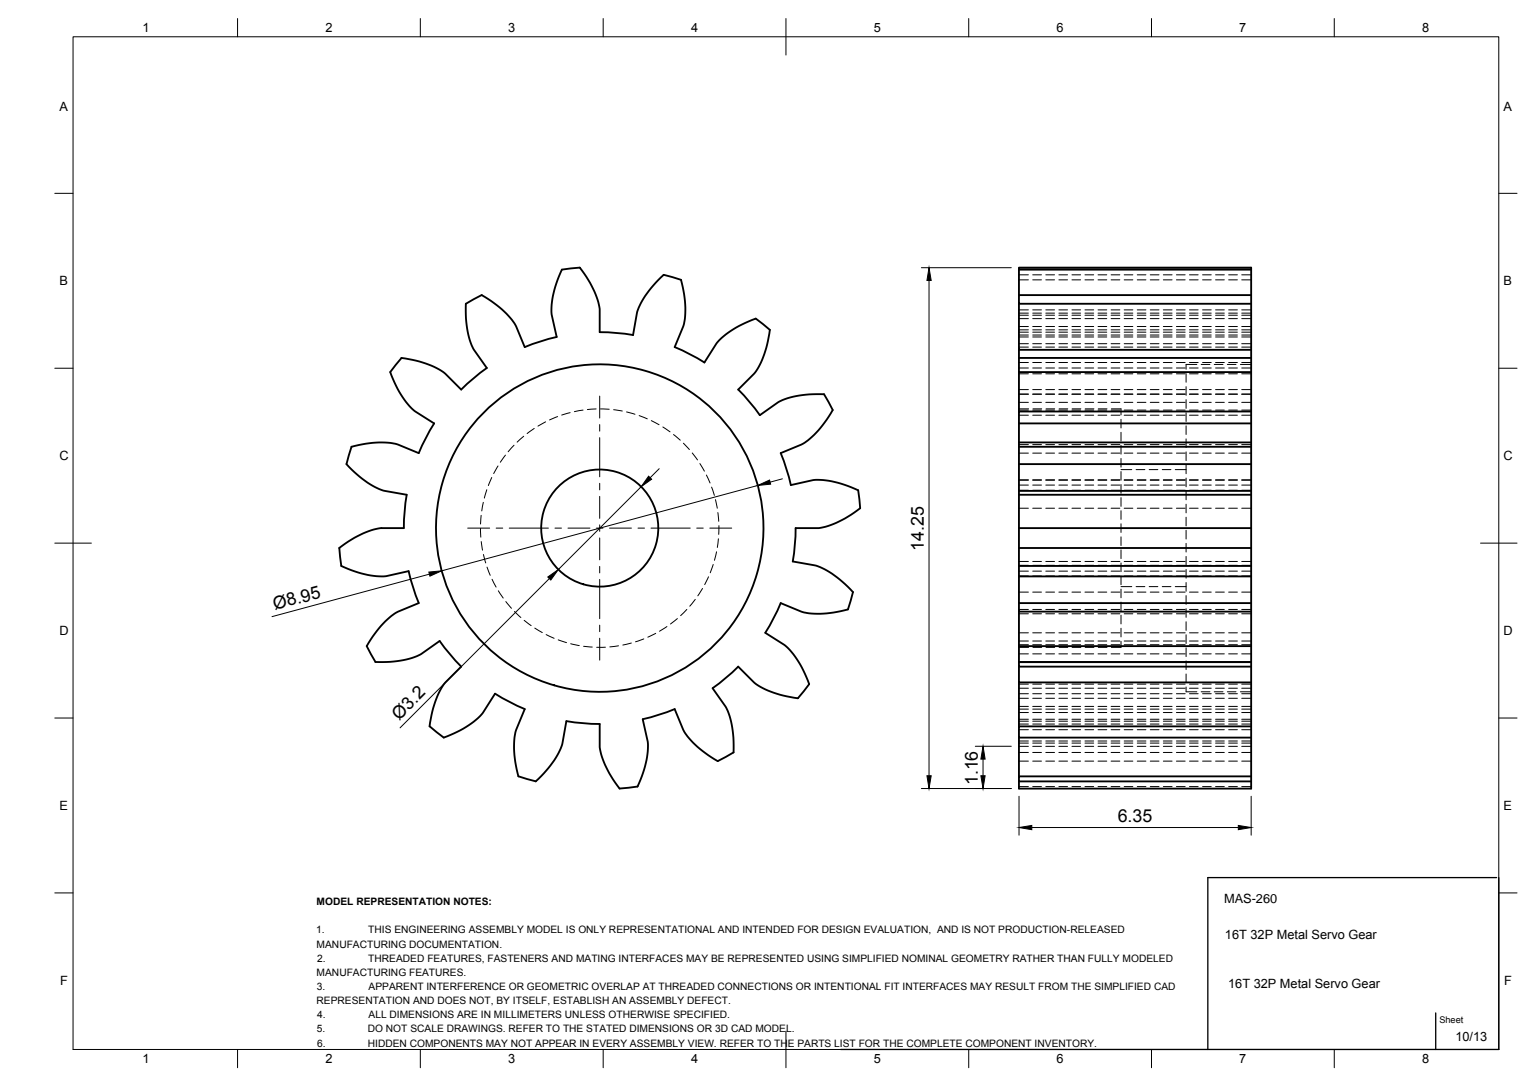
ISO-10303-21;
HEADER;
/* Generated by software containing ST-Developer
 * from STEP Tools, Inc. (www.steptools.com) 
 */

FILE_DESCRIPTION(
/* description */ (''),
/* implementation_level */ '2;1');

FILE_NAME(
/* name */ '16T 32P Metal Servo Gear.step',
/* time_stamp */ '2026-10-15T13:29:10-07:00',
/* author */ (''),
/* organization */ (''),
/* preprocessor_version */ 'ST-DEVELOPER v20.2',
/* originating_system */ 'Autodesk Translation Framework v15.15.0.0',
/* authorisation */ '');

FILE_SCHEMA (('AUTOMOTIVE_DESIGN { 1 0 10303 214 3 1 1 }'));
ENDSEC;

DATA;
#10=MECHANICAL_DESIGN_GEOMETRIC_PRESENTATION_REPRESENTATION('',(#936),#83219);
#508=B_SPLINE_CURVE_WITH_KNOTS('',5,(#37220,#37221,#37222,#37223,#37224,
#37225,#37226,#37227,#37228,#37229,#37230,#37231,#37232,#37233,#37234,#37235,
#37236,#37237,#37238,#37239,#37240,#37241,#37242,#37243,#37244,#37245,#37246,
#37247,#37248,#37249,#37250,#37251,#37252,#37253,#37254),.UNSPECIFIED.,
 .F.,.F.,(6,1,1,1,1,1,1,1,1,1,1,1,1,1,1,1,1,1,1,1,1,1,1,1,1,1,1,1,1,1,6),
(0.,0.0333333333333333,0.0666666666666667,0.1,0.133333333333333,0.166666666666667,
0.2,0.233333333333333,0.266666666666667,0.3,0.333333333333333,0.366666666666667,
0.4,0.433333333333333,0.466666666666667,0.5,0.533333333333333,0.566666666666667,
0.6,0.633333333333333,0.666666666666667,0.7,0.733333333333333,0.766666666666667,
0.8,0.833333333333333,0.866666666666667,0.9,0.933333333333333,0.966666666666667,
1.),.UNSPECIFIED.);
#509=B_SPLINE_CURVE_WITH_KNOTS('',5,(#37256,#37257,#37258,#37259,#37260,
#37261,#37262,#37263,#37264,#37265,#37266,#37267,#37268,#37269,#37270,#37271,
#37272,#37273,#37274,#37275,#37276,#37277,#37278,#37279,#37280,#37281,#37282,
#37283,#37284,#37285,#37286,#37287,#37288,#37289,#37290),.UNSPECIFIED.,
 .F.,.F.,(6,1,1,1,1,1,1,1,1,1,1,1,1,1,1,1,1,1,1,1,1,1,1,1,1,1,1,1,1,1,6),
(0.,0.0333333333333333,0.0666666666666667,0.1,0.133333333333333,0.166666666666667,
0.2,0.233333333333333,0.266666666666667,0.3,0.333333333333333,0.366666666666667,
0.4,0.433333333333333,0.466666666666667,0.5,0.533333333333333,0.566666666666667,
0.6,0.633333333333333,0.666666666666667,0.7,0.733333333333333,0.766666666666667,
0.8,0.833333333333333,0.866666666666667,0.9,0.933333333333333,0.966666666666667,
1.),.UNSPECIFIED.);
#510=B_SPLINE_CURVE_WITH_KNOTS('',5,(#37368,#37369,#37370,#37371,#37372,
#37373,#37374,#37375,#37376,#37377,#37378,#37379,#37380,#37381,#37382,#37383,
#37384,#37385,#37386,#37387,#37388,#37389,#37390,#37391,#37392,#37393,#37394,
#37395,#37396,#37397,#37398,#37399,#37400,#37401,#37402),.UNSPECIFIED.,
 .F.,.F.,(6,1,1,1,1,1,1,1,1,1,1,1,1,1,1,1,1,1,1,1,1,1,1,1,1,1,1,1,1,1,6),
(0.,0.0333333333333333,0.0666666666666667,0.1,0.133333333333333,0.166666666666667,
0.2,0.233333333333333,0.266666666666667,0.3,0.333333333333333,0.366666666666667,
0.4,0.433333333333333,0.466666666666667,0.5,0.533333333333333,0.566666666666667,
0.6,0.633333333333333,0.666666666666667,0.7,0.733333333333333,0.766666666666667,
0.8,0.833333333333333,0.866666666666667,0.9,0.933333333333333,0.966666666666667,
1.),.UNSPECIFIED.);
#511=B_SPLINE_CURVE_WITH_KNOTS('',5,(#37403,#37404,#37405,#37406,#37407,
#37408,#37409,#37410,#37411,#37412,#37413,#37414,#37415,#37416,#37417,#37418,
#37419,#37420,#37421,#37422,#37423,#37424,#37425,#37426,#37427,#37428,#37429,
#37430,#37431,#37432,#37433,#37434,#37435,#37436,#37437),.UNSPECIFIED.,
 .F.,.F.,(6,1,1,1,1,1,1,1,1,1,1,1,1,1,1,1,1,1,1,1,1,1,1,1,1,1,1,1,1,1,6),
(-1.,-0.966666666666667,-0.933333333333333,-0.9,-0.866666666666667,-0.833333333333333,
-0.8,-0.766666666666667,-0.733333333333333,-0.7,-0.666666666666667,-0.633333333333333,
-0.6,-0.566666666666667,-0.533333333333333,-0.5,-0.466666666666667,-0.433333333333333,
-0.4,-0.366666666666667,-0.333333333333333,-0.3,-0.266666666666667,-0.233333333333333,
-0.2,-0.166666666666667,-0.133333333333333,-0.1,-0.0666666666666667,-0.0333333333333333,
0.),.UNSPECIFIED.);
#512=B_SPLINE_CURVE_WITH_KNOTS('',5,(#37444,#37445,#37446,#37447,#37448,
#37449,#37450,#37451,#37452,#37453,#37454,#37455,#37456,#37457,#37458,#37459,
#37460,#37461,#37462,#37463,#37464,#37465,#37466,#37467,#37468,#37469,#37470,
#37471,#37472,#37473,#37474,#37475,#37476,#37477,#37478),.UNSPECIFIED.,
 .F.,.F.,(6,1,1,1,1,1,1,1,1,1,1,1,1,1,1,1,1,1,1,1,1,1,1,1,1,1,1,1,1,1,6),
(0.,0.0333333333333333,0.0666666666666667,0.1,0.133333333333333,0.166666666666667,
0.2,0.233333333333333,0.266666666666667,0.3,0.333333333333333,0.366666666666667,
0.4,0.433333333333333,0.466666666666667,0.5,0.533333333333333,0.566666666666667,
0.6,0.633333333333333,0.666666666666667,0.7,0.733333333333333,0.766666666666667,
0.8,0.833333333333333,0.866666666666667,0.9,0.933333333333333,0.966666666666667,
1.),.UNSPECIFIED.);
#513=B_SPLINE_CURVE_WITH_KNOTS('',5,(#37482,#37483,#37484,#37485,#37486,
#37487,#37488,#37489,#37490,#37491,#37492,#37493,#37494,#37495,#37496,#37497,
#37498,#37499,#37500,#37501,#37502,#37503,#37504,#37505,#37506,#37507,#37508,
#37509,#37510,#37511,#37512,#37513,#37514,#37515,#37516),.UNSPECIFIED.,
 .F.,.F.,(6,1,1,1,1,1,1,1,1,1,1,1,1,1,1,1,1,1,1,1,1,1,1,1,1,1,1,1,1,1,6),
(0.,0.0333333333333333,0.0666666666666667,0.1,0.133333333333333,0.166666666666667,
0.2,0.233333333333333,0.266666666666667,0.3,0.333333333333333,0.366666666666667,
0.4,0.433333333333333,0.466666666666667,0.5,0.533333333333333,0.566666666666667,
0.6,0.633333333333333,0.666666666666667,0.7,0.733333333333333,0.766666666666667,
0.8,0.833333333333333,0.866666666666667,0.9,0.933333333333333,0.966666666666667,
1.),.UNSPECIFIED.);
#514=B_SPLINE_CURVE_WITH_KNOTS('',5,(#37524,#37525,#37526,#37527,#37528,
#37529,#37530,#37531,#37532,#37533,#37534,#37535,#37536,#37537,#37538,#37539,
#37540,#37541,#37542,#37543,#37544,#37545,#37546,#37547,#37548,#37549,#37550,
#37551,#37552,#37553,#37554,#37555,#37556,#37557,#37558),.UNSPECIFIED.,
 .F.,.F.,(6,1,1,1,1,1,1,1,1,1,1,1,1,1,1,1,1,1,1,1,1,1,1,1,1,1,1,1,1,1,6),
(0.,0.0333333333333333,0.0666666666666667,0.1,0.133333333333333,0.166666666666667,
0.2,0.233333333333333,0.266666666666667,0.3,0.333333333333333,0.366666666666667,
0.4,0.433333333333333,0.466666666666667,0.5,0.533333333333333,0.566666666666667,
0.6,0.633333333333333,0.666666666666667,0.7,0.733333333333333,0.766666666666667,
0.8,0.833333333333333,0.866666666666667,0.9,0.933333333333333,0.966666666666667,
1.),.UNSPECIFIED.);
#515=B_SPLINE_CURVE_WITH_KNOTS('',5,(#37562,#37563,#37564,#37565,#37566,
#37567,#37568,#37569,#37570,#37571,#37572,#37573,#37574,#37575,#37576,#37577,
#37578,#37579,#37580,#37581,#37582,#37583,#37584,#37585,#37586,#37587,#37588,
#37589,#37590,#37591,#37592,#37593,#37594,#37595,#37596),.UNSPECIFIED.,
 .F.,.F.,(6,1,1,1,1,1,1,1,1,1,1,1,1,1,1,1,1,1,1,1,1,1,1,1,1,1,1,1,1,1,6),
(0.,0.0333333333333333,0.0666666666666667,0.1,0.133333333333333,0.166666666666667,
0.2,0.233333333333333,0.266666666666667,0.3,0.333333333333333,0.366666666666667,
0.4,0.433333333333333,0.466666666666667,0.5,0.533333333333333,0.566666666666667,
0.6,0.633333333333333,0.666666666666667,0.7,0.733333333333333,0.766666666666667,
0.8,0.833333333333333,0.866666666666667,0.9,0.933333333333333,0.966666666666667,
1.),.UNSPECIFIED.);
#516=B_SPLINE_CURVE_WITH_KNOTS('',5,(#37604,#37605,#37606,#37607,#37608,
#37609,#37610,#37611,#37612,#37613,#37614,#37615,#37616,#37617,#37618,#37619,
#37620,#37621,#37622,#37623,#37624,#37625,#37626,#37627,#37628,#37629,#37630,
#37631,#37632,#37633,#37634,#37635,#37636,#37637,#37638),.UNSPECIFIED.,
 .F.,.F.,(6,1,1,1,1,1,1,1,1,1,1,1,1,1,1,1,1,1,1,1,1,1,1,1,1,1,1,1,1,1,6),
(0.,0.0333333333333333,0.0666666666666667,0.1,0.133333333333333,0.166666666666667,
0.2,0.233333333333333,0.266666666666667,0.3,0.333333333333333,0.366666666666667,
0.4,0.433333333333333,0.466666666666667,0.5,0.533333333333333,0.566666666666667,
0.6,0.633333333333333,0.666666666666667,0.7,0.733333333333333,0.766666666666667,
0.8,0.833333333333333,0.866666666666667,0.9,0.933333333333333,0.966666666666667,
1.),.UNSPECIFIED.);
#517=B_SPLINE_CURVE_WITH_KNOTS('',5,(#37642,#37643,#37644,#37645,#37646,
#37647,#37648,#37649,#37650,#37651,#37652,#37653,#37654,#37655,#37656,#37657,
#37658,#37659,#37660,#37661,#37662,#37663,#37664,#37665,#37666,#37667,#37668,
#37669,#37670,#37671,#37672,#37673,#37674,#37675,#37676),.UNSPECIFIED.,
 .F.,.F.,(6,1,1,1,1,1,1,1,1,1,1,1,1,1,1,1,1,1,1,1,1,1,1,1,1,1,1,1,1,1,6),
(0.,0.0333333333333333,0.0666666666666667,0.1,0.133333333333333,0.166666666666667,
0.2,0.233333333333333,0.266666666666667,0.3,0.333333333333333,0.366666666666667,
0.4,0.433333333333333,0.466666666666667,0.5,0.533333333333333,0.566666666666667,
0.6,0.633333333333333,0.666666666666667,0.7,0.733333333333333,0.766666666666667,
0.8,0.833333333333333,0.866666666666667,0.9,0.933333333333333,0.966666666666667,
1.),.UNSPECIFIED.);
#518=B_SPLINE_CURVE_WITH_KNOTS('',5,(#37684,#37685,#37686,#37687,#37688,
#37689,#37690,#37691,#37692,#37693,#37694,#37695,#37696,#37697,#37698,#37699,
#37700,#37701,#37702,#37703,#37704,#37705,#37706,#37707,#37708,#37709,#37710,
#37711,#37712,#37713,#37714,#37715,#37716,#37717,#37718),.UNSPECIFIED.,
 .F.,.F.,(6,1,1,1,1,1,1,1,1,1,1,1,1,1,1,1,1,1,1,1,1,1,1,1,1,1,1,1,1,1,6),
(0.,0.0333333333333333,0.0666666666666667,0.1,0.133333333333333,0.166666666666667,
0.2,0.233333333333333,0.266666666666667,0.3,0.333333333333333,0.366666666666667,
0.4,0.433333333333333,0.466666666666667,0.5,0.533333333333333,0.566666666666667,
0.6,0.633333333333333,0.666666666666667,0.7,0.733333333333333,0.766666666666667,
0.8,0.833333333333333,0.866666666666667,0.9,0.933333333333333,0.966666666666667,
1.),.UNSPECIFIED.);
#519=B_SPLINE_CURVE_WITH_KNOTS('',5,(#37722,#37723,#37724,#37725,#37726,
#37727,#37728,#37729,#37730,#37731,#37732,#37733,#37734,#37735,#37736,#37737,
#37738,#37739,#37740,#37741,#37742,#37743,#37744,#37745,#37746,#37747,#37748,
#37749,#37750,#37751,#37752,#37753,#37754,#37755,#37756),.UNSPECIFIED.,
 .F.,.F.,(6,1,1,1,1,1,1,1,1,1,1,1,1,1,1,1,1,1,1,1,1,1,1,1,1,1,1,1,1,1,6),
(0.,0.0333333333333333,0.0666666666666667,0.1,0.133333333333333,0.166666666666667,
0.2,0.233333333333333,0.266666666666667,0.3,0.333333333333333,0.366666666666667,
0.4,0.433333333333333,0.466666666666667,0.5,0.533333333333333,0.566666666666667,
0.6,0.633333333333333,0.666666666666667,0.7,0.733333333333333,0.766666666666667,
0.8,0.833333333333333,0.866666666666667,0.9,0.933333333333333,0.966666666666667,
1.),.UNSPECIFIED.);
#520=B_SPLINE_CURVE_WITH_KNOTS('',5,(#37764,#37765,#37766,#37767,#37768,
#37769,#37770,#37771,#37772,#37773,#37774,#37775,#37776,#37777,#37778,#37779,
#37780,#37781,#37782,#37783,#37784,#37785,#37786,#37787,#37788,#37789,#37790,
#37791,#37792,#37793,#37794,#37795,#37796,#37797,#37798),.UNSPECIFIED.,
 .F.,.F.,(6,1,1,1,1,1,1,1,1,1,1,1,1,1,1,1,1,1,1,1,1,1,1,1,1,1,1,1,1,1,6),
(0.,0.0333333333333333,0.0666666666666667,0.1,0.133333333333333,0.166666666666667,
0.2,0.233333333333333,0.266666666666667,0.3,0.333333333333333,0.366666666666667,
0.4,0.433333333333333,0.466666666666667,0.5,0.533333333333333,0.566666666666667,
0.6,0.633333333333333,0.666666666666667,0.7,0.733333333333333,0.766666666666667,
0.8,0.833333333333333,0.866666666666667,0.9,0.933333333333333,0.966666666666667,
1.),.UNSPECIFIED.);
#521=B_SPLINE_CURVE_WITH_KNOTS('',5,(#37802,#37803,#37804,#37805,#37806,
#37807,#37808,#37809,#37810,#37811,#37812,#37813,#37814,#37815,#37816,#37817,
#37818,#37819,#37820,#37821,#37822,#37823,#37824,#37825,#37826,#37827,#37828,
#37829,#37830,#37831,#37832,#37833,#37834,#37835,#37836),.UNSPECIFIED.,
 .F.,.F.,(6,1,1,1,1,1,1,1,1,1,1,1,1,1,1,1,1,1,1,1,1,1,1,1,1,1,1,1,1,1,6),
(0.,0.0333333333333333,0.0666666666666667,0.1,0.133333333333333,0.166666666666667,
0.2,0.233333333333333,0.266666666666667,0.3,0.333333333333333,0.366666666666667,
0.4,0.433333333333333,0.466666666666667,0.5,0.533333333333333,0.566666666666667,
0.6,0.633333333333333,0.666666666666667,0.7,0.733333333333333,0.766666666666667,
0.8,0.833333333333333,0.866666666666667,0.9,0.933333333333333,0.966666666666667,
1.),.UNSPECIFIED.);
#522=B_SPLINE_CURVE_WITH_KNOTS('',5,(#37844,#37845,#37846,#37847,#37848,
#37849,#37850,#37851,#37852,#37853,#37854,#37855,#37856,#37857,#37858,#37859,
#37860,#37861,#37862,#37863,#37864,#37865,#37866,#37867,#37868,#37869,#37870,
#37871,#37872,#37873,#37874,#37875,#37876,#37877,#37878),.UNSPECIFIED.,
 .F.,.F.,(6,1,1,1,1,1,1,1,1,1,1,1,1,1,1,1,1,1,1,1,1,1,1,1,1,1,1,1,1,1,6),
(0.,0.0333333333333333,0.0666666666666667,0.1,0.133333333333333,0.166666666666667,
0.2,0.233333333333333,0.266666666666667,0.3,0.333333333333333,0.366666666666667,
0.4,0.433333333333333,0.466666666666667,0.5,0.533333333333333,0.566666666666667,
0.6,0.633333333333333,0.666666666666667,0.7,0.733333333333333,0.766666666666667,
0.8,0.833333333333333,0.866666666666667,0.9,0.933333333333333,0.966666666666667,
1.),.UNSPECIFIED.);
#523=B_SPLINE_CURVE_WITH_KNOTS('',5,(#37882,#37883,#37884,#37885,#37886,
#37887,#37888,#37889,#37890,#37891,#37892,#37893,#37894,#37895,#37896,#37897,
#37898,#37899,#37900,#37901,#37902,#37903,#37904,#37905,#37906,#37907,#37908,
#37909,#37910,#37911,#37912,#37913,#37914,#37915,#37916),.UNSPECIFIED.,
 .F.,.F.,(6,1,1,1,1,1,1,1,1,1,1,1,1,1,1,1,1,1,1,1,1,1,1,1,1,1,1,1,1,1,6),
(0.,0.0333333333333333,0.0666666666666667,0.1,0.133333333333333,0.166666666666667,
0.2,0.233333333333333,0.266666666666667,0.3,0.333333333333333,0.366666666666667,
0.4,0.433333333333333,0.466666666666667,0.5,0.533333333333333,0.566666666666667,
0.6,0.633333333333333,0.666666666666667,0.7,0.733333333333333,0.766666666666667,
0.8,0.833333333333333,0.866666666666667,0.9,0.933333333333333,0.966666666666667,
1.),.UNSPECIFIED.);
#524=B_SPLINE_CURVE_WITH_KNOTS('',5,(#37924,#37925,#37926,#37927,#37928,
#37929,#37930,#37931,#37932,#37933,#37934,#37935,#37936,#37937,#37938,#37939,
#37940,#37941,#37942,#37943,#37944,#37945,#37946,#37947,#37948,#37949,#37950,
#37951,#37952,#37953,#37954,#37955,#37956,#37957,#37958),.UNSPECIFIED.,
 .F.,.F.,(6,1,1,1,1,1,1,1,1,1,1,1,1,1,1,1,1,1,1,1,1,1,1,1,1,1,1,1,1,1,6),
(0.,0.0333333333333333,0.0666666666666667,0.1,0.133333333333333,0.166666666666667,
0.2,0.233333333333333,0.266666666666667,0.3,0.333333333333333,0.366666666666667,
0.4,0.433333333333333,0.466666666666667,0.5,0.533333333333333,0.566666666666667,
0.6,0.633333333333333,0.666666666666667,0.7,0.733333333333333,0.766666666666667,
0.8,0.833333333333333,0.866666666666667,0.9,0.933333333333333,0.966666666666667,
1.),.UNSPECIFIED.);
#525=B_SPLINE_CURVE_WITH_KNOTS('',5,(#37962,#37963,#37964,#37965,#37966,
#37967,#37968,#37969,#37970,#37971,#37972,#37973,#37974,#37975,#37976,#37977,
#37978,#37979,#37980,#37981,#37982,#37983,#37984,#37985,#37986,#37987,#37988,
#37989,#37990,#37991,#37992,#37993,#37994,#37995,#37996),.UNSPECIFIED.,
 .F.,.F.,(6,1,1,1,1,1,1,1,1,1,1,1,1,1,1,1,1,1,1,1,1,1,1,1,1,1,1,1,1,1,6),
(0.,0.0333333333333333,0.0666666666666667,0.1,0.133333333333333,0.166666666666667,
0.2,0.233333333333333,0.266666666666667,0.3,0.333333333333333,0.366666666666667,
0.4,0.433333333333333,0.466666666666667,0.5,0.533333333333333,0.566666666666667,
0.6,0.633333333333333,0.666666666666667,0.7,0.733333333333333,0.766666666666667,
0.8,0.833333333333333,0.866666666666667,0.9,0.933333333333333,0.966666666666667,
1.),.UNSPECIFIED.);
#526=B_SPLINE_CURVE_WITH_KNOTS('',5,(#38004,#38005,#38006,#38007,#38008,
#38009,#38010,#38011,#38012,#38013,#38014,#38015,#38016,#38017,#38018,#38019,
#38020,#38021,#38022,#38023,#38024,#38025,#38026,#38027,#38028,#38029,#38030,
#38031,#38032,#38033,#38034,#38035,#38036,#38037,#38038),.UNSPECIFIED.,
 .F.,.F.,(6,1,1,1,1,1,1,1,1,1,1,1,1,1,1,1,1,1,1,1,1,1,1,1,1,1,1,1,1,1,6),
(0.,0.0333333333333333,0.0666666666666667,0.1,0.133333333333333,0.166666666666667,
0.2,0.233333333333333,0.266666666666667,0.3,0.333333333333333,0.366666666666667,
0.4,0.433333333333333,0.466666666666667,0.5,0.533333333333333,0.566666666666667,
0.6,0.633333333333333,0.666666666666667,0.7,0.733333333333333,0.766666666666667,
0.8,0.833333333333333,0.866666666666667,0.9,0.933333333333333,0.966666666666667,
1.),.UNSPECIFIED.);
#527=B_SPLINE_CURVE_WITH_KNOTS('',5,(#38042,#38043,#38044,#38045,#38046,
#38047,#38048,#38049,#38050,#38051,#38052,#38053,#38054,#38055,#38056,#38057,
#38058,#38059,#38060,#38061,#38062,#38063,#38064,#38065,#38066,#38067,#38068,
#38069,#38070,#38071,#38072,#38073,#38074,#38075,#38076),.UNSPECIFIED.,
 .F.,.F.,(6,1,1,1,1,1,1,1,1,1,1,1,1,1,1,1,1,1,1,1,1,1,1,1,1,1,1,1,1,1,6),
(0.,0.0333333333333333,0.0666666666666667,0.1,0.133333333333333,0.166666666666667,
0.2,0.233333333333333,0.266666666666667,0.3,0.333333333333333,0.366666666666667,
0.4,0.433333333333333,0.466666666666667,0.5,0.533333333333333,0.566666666666667,
0.6,0.633333333333333,0.666666666666667,0.7,0.733333333333333,0.766666666666667,
0.8,0.833333333333333,0.866666666666667,0.9,0.933333333333333,0.966666666666667,
1.),.UNSPECIFIED.);
#528=B_SPLINE_CURVE_WITH_KNOTS('',5,(#38084,#38085,#38086,#38087,#38088,
#38089,#38090,#38091,#38092,#38093,#38094,#38095,#38096,#38097,#38098,#38099,
#38100,#38101,#38102,#38103,#38104,#38105,#38106,#38107,#38108,#38109,#38110,
#38111,#38112,#38113,#38114,#38115,#38116,#38117,#38118),.UNSPECIFIED.,
 .F.,.F.,(6,1,1,1,1,1,1,1,1,1,1,1,1,1,1,1,1,1,1,1,1,1,1,1,1,1,1,1,1,1,6),
(0.,0.0333333333333333,0.0666666666666667,0.1,0.133333333333333,0.166666666666667,
0.2,0.233333333333333,0.266666666666667,0.3,0.333333333333333,0.366666666666667,
0.4,0.433333333333333,0.466666666666667,0.5,0.533333333333333,0.566666666666667,
0.6,0.633333333333333,0.666666666666667,0.7,0.733333333333333,0.766666666666667,
0.8,0.833333333333333,0.866666666666667,0.9,0.933333333333333,0.966666666666667,
1.),.UNSPECIFIED.);
#529=B_SPLINE_CURVE_WITH_KNOTS('',5,(#38122,#38123,#38124,#38125,#38126,
#38127,#38128,#38129,#38130,#38131,#38132,#38133,#38134,#38135,#38136,#38137,
#38138,#38139,#38140,#38141,#38142,#38143,#38144,#38145,#38146,#38147,#38148,
#38149,#38150,#38151,#38152,#38153,#38154,#38155,#38156),.UNSPECIFIED.,
 .F.,.F.,(6,1,1,1,1,1,1,1,1,1,1,1,1,1,1,1,1,1,1,1,1,1,1,1,1,1,1,1,1,1,6),
(0.,0.0333333333333333,0.0666666666666667,0.1,0.133333333333333,0.166666666666667,
0.2,0.233333333333333,0.266666666666667,0.3,0.333333333333333,0.366666666666667,
0.4,0.433333333333333,0.466666666666667,0.5,0.533333333333333,0.566666666666667,
0.6,0.633333333333333,0.666666666666667,0.7,0.733333333333333,0.766666666666667,
0.8,0.833333333333333,0.866666666666667,0.9,0.933333333333333,0.966666666666667,
1.),.UNSPECIFIED.);
#530=B_SPLINE_CURVE_WITH_KNOTS('',5,(#38164,#38165,#38166,#38167,#38168,
#38169,#38170,#38171,#38172,#38173,#38174,#38175,#38176,#38177,#38178,#38179,
#38180,#38181,#38182,#38183,#38184,#38185,#38186,#38187,#38188,#38189,#38190,
#38191,#38192,#38193,#38194,#38195,#38196,#38197,#38198),.UNSPECIFIED.,
 .F.,.F.,(6,1,1,1,1,1,1,1,1,1,1,1,1,1,1,1,1,1,1,1,1,1,1,1,1,1,1,1,1,1,6),
(0.,0.0333333333333333,0.0666666666666667,0.1,0.133333333333333,0.166666666666667,
0.2,0.233333333333333,0.266666666666667,0.3,0.333333333333333,0.366666666666667,
0.4,0.433333333333333,0.466666666666667,0.5,0.533333333333333,0.566666666666667,
0.6,0.633333333333333,0.666666666666667,0.7,0.733333333333333,0.766666666666667,
0.8,0.833333333333333,0.866666666666667,0.9,0.933333333333333,0.966666666666667,
1.),.UNSPECIFIED.);
#531=B_SPLINE_CURVE_WITH_KNOTS('',5,(#38202,#38203,#38204,#38205,#38206,
#38207,#38208,#38209,#38210,#38211,#38212,#38213,#38214,#38215,#38216,#38217,
#38218,#38219,#38220,#38221,#38222,#38223,#38224,#38225,#38226,#38227,#38228,
#38229,#38230,#38231,#38232,#38233,#38234,#38235,#38236),.UNSPECIFIED.,
 .F.,.F.,(6,1,1,1,1,1,1,1,1,1,1,1,1,1,1,1,1,1,1,1,1,1,1,1,1,1,1,1,1,1,6),
(0.,0.0333333333333333,0.0666666666666667,0.1,0.133333333333333,0.166666666666667,
0.2,0.233333333333333,0.266666666666667,0.3,0.333333333333333,0.366666666666667,
0.4,0.433333333333333,0.466666666666667,0.5,0.533333333333333,0.566666666666667,
0.6,0.633333333333333,0.666666666666667,0.7,0.733333333333333,0.766666666666667,
0.8,0.833333333333333,0.866666666666667,0.9,0.933333333333333,0.966666666666667,
1.),.UNSPECIFIED.);
#532=B_SPLINE_CURVE_WITH_KNOTS('',5,(#38244,#38245,#38246,#38247,#38248,
#38249,#38250,#38251,#38252,#38253,#38254,#38255,#38256,#38257,#38258,#38259,
#38260,#38261,#38262,#38263,#38264,#38265,#38266,#38267,#38268,#38269,#38270,
#38271,#38272,#38273,#38274,#38275,#38276,#38277,#38278),.UNSPECIFIED.,
 .F.,.F.,(6,1,1,1,1,1,1,1,1,1,1,1,1,1,1,1,1,1,1,1,1,1,1,1,1,1,1,1,1,1,6),
(0.,0.0333333333333333,0.0666666666666667,0.1,0.133333333333333,0.166666666666667,
0.2,0.233333333333333,0.266666666666667,0.3,0.333333333333333,0.366666666666667,
0.4,0.433333333333333,0.466666666666667,0.5,0.533333333333333,0.566666666666667,
0.6,0.633333333333333,0.666666666666667,0.7,0.733333333333333,0.766666666666667,
0.8,0.833333333333333,0.866666666666667,0.9,0.933333333333333,0.966666666666667,
1.),.UNSPECIFIED.);
#533=B_SPLINE_CURVE_WITH_KNOTS('',5,(#38282,#38283,#38284,#38285,#38286,
#38287,#38288,#38289,#38290,#38291,#38292,#38293,#38294,#38295,#38296,#38297,
#38298,#38299,#38300,#38301,#38302,#38303,#38304,#38305,#38306,#38307,#38308,
#38309,#38310,#38311,#38312,#38313,#38314,#38315,#38316),.UNSPECIFIED.,
 .F.,.F.,(6,1,1,1,1,1,1,1,1,1,1,1,1,1,1,1,1,1,1,1,1,1,1,1,1,1,1,1,1,1,6),
(0.,0.0333333333333333,0.0666666666666667,0.1,0.133333333333333,0.166666666666667,
0.2,0.233333333333333,0.266666666666667,0.3,0.333333333333333,0.366666666666667,
0.4,0.433333333333333,0.466666666666667,0.5,0.533333333333333,0.566666666666667,
0.6,0.633333333333333,0.666666666666667,0.7,0.733333333333333,0.766666666666667,
0.8,0.833333333333333,0.866666666666667,0.9,0.933333333333333,0.966666666666667,
1.),.UNSPECIFIED.);
#534=B_SPLINE_CURVE_WITH_KNOTS('',5,(#38324,#38325,#38326,#38327,#38328,
#38329,#38330,#38331,#38332,#38333,#38334,#38335,#38336,#38337,#38338,#38339,
#38340,#38341,#38342,#38343,#38344,#38345,#38346,#38347,#38348,#38349,#38350,
#38351,#38352,#38353,#38354,#38355,#38356,#38357,#38358),.UNSPECIFIED.,
 .F.,.F.,(6,1,1,1,1,1,1,1,1,1,1,1,1,1,1,1,1,1,1,1,1,1,1,1,1,1,1,1,1,1,6),
(0.,0.0333333333333333,0.0666666666666667,0.1,0.133333333333333,0.166666666666667,
0.2,0.233333333333333,0.266666666666667,0.3,0.333333333333333,0.366666666666667,
0.4,0.433333333333333,0.466666666666667,0.5,0.533333333333333,0.566666666666667,
0.6,0.633333333333333,0.666666666666667,0.7,0.733333333333333,0.766666666666667,
0.8,0.833333333333333,0.866666666666667,0.9,0.933333333333333,0.966666666666667,
1.),.UNSPECIFIED.);
#535=B_SPLINE_CURVE_WITH_KNOTS('',5,(#38362,#38363,#38364,#38365,#38366,
#38367,#38368,#38369,#38370,#38371,#38372,#38373,#38374,#38375,#38376,#38377,
#38378,#38379,#38380,#38381,#38382,#38383,#38384,#38385,#38386,#38387,#38388,
#38389,#38390,#38391,#38392,#38393,#38394,#38395,#38396),.UNSPECIFIED.,
 .F.,.F.,(6,1,1,1,1,1,1,1,1,1,1,1,1,1,1,1,1,1,1,1,1,1,1,1,1,1,1,1,1,1,6),
(0.,0.0333333333333333,0.0666666666666667,0.1,0.133333333333333,0.166666666666667,
0.2,0.233333333333333,0.266666666666667,0.3,0.333333333333333,0.366666666666667,
0.4,0.433333333333333,0.466666666666667,0.5,0.533333333333333,0.566666666666667,
0.6,0.633333333333333,0.666666666666667,0.7,0.733333333333333,0.766666666666667,
0.8,0.833333333333333,0.866666666666667,0.9,0.933333333333333,0.966666666666667,
1.),.UNSPECIFIED.);
#536=B_SPLINE_CURVE_WITH_KNOTS('',5,(#38404,#38405,#38406,#38407,#38408,
#38409,#38410,#38411,#38412,#38413,#38414,#38415,#38416,#38417,#38418,#38419,
#38420,#38421,#38422,#38423,#38424,#38425,#38426,#38427,#38428,#38429,#38430,
#38431,#38432,#38433,#38434,#38435,#38436,#38437,#38438),.UNSPECIFIED.,
 .F.,.F.,(6,1,1,1,1,1,1,1,1,1,1,1,1,1,1,1,1,1,1,1,1,1,1,1,1,1,1,1,1,1,6),
(0.,0.0333333333333333,0.0666666666666667,0.1,0.133333333333333,0.166666666666667,
0.2,0.233333333333333,0.266666666666667,0.3,0.333333333333333,0.366666666666667,
0.4,0.433333333333333,0.466666666666667,0.5,0.533333333333333,0.566666666666667,
0.6,0.633333333333333,0.666666666666667,0.7,0.733333333333333,0.766666666666667,
0.8,0.833333333333333,0.866666666666667,0.9,0.933333333333333,0.966666666666667,
1.),.UNSPECIFIED.);
#537=B_SPLINE_CURVE_WITH_KNOTS('',5,(#38442,#38443,#38444,#38445,#38446,
#38447,#38448,#38449,#38450,#38451,#38452,#38453,#38454,#38455,#38456,#38457,
#38458,#38459,#38460,#38461,#38462,#38463,#38464,#38465,#38466,#38467,#38468,
#38469,#38470,#38471,#38472,#38473,#38474,#38475,#38476),.UNSPECIFIED.,
 .F.,.F.,(6,1,1,1,1,1,1,1,1,1,1,1,1,1,1,1,1,1,1,1,1,1,1,1,1,1,1,1,1,1,6),
(0.,0.0333333333333333,0.0666666666666667,0.1,0.133333333333333,0.166666666666667,
0.2,0.233333333333333,0.266666666666667,0.3,0.333333333333333,0.366666666666667,
0.4,0.433333333333333,0.466666666666667,0.5,0.533333333333333,0.566666666666667,
0.6,0.633333333333333,0.666666666666667,0.7,0.733333333333333,0.766666666666667,
0.8,0.833333333333333,0.866666666666667,0.9,0.933333333333333,0.966666666666667,
1.),.UNSPECIFIED.);
#538=B_SPLINE_CURVE_WITH_KNOTS('',5,(#38484,#38485,#38486,#38487,#38488,
#38489,#38490,#38491,#38492,#38493,#38494,#38495,#38496,#38497,#38498,#38499,
#38500,#38501,#38502,#38503,#38504,#38505,#38506,#38507,#38508,#38509,#38510,
#38511,#38512,#38513,#38514,#38515,#38516,#38517,#38518),.UNSPECIFIED.,
 .F.,.F.,(6,1,1,1,1,1,1,1,1,1,1,1,1,1,1,1,1,1,1,1,1,1,1,1,1,1,1,1,1,1,6),
(0.,0.0333333333333333,0.0666666666666667,0.1,0.133333333333333,0.166666666666667,
0.2,0.233333333333333,0.266666666666667,0.3,0.333333333333333,0.366666666666667,
0.4,0.433333333333333,0.466666666666667,0.5,0.533333333333333,0.566666666666667,
0.6,0.633333333333333,0.666666666666667,0.7,0.733333333333333,0.766666666666667,
0.8,0.833333333333333,0.866666666666667,0.9,0.933333333333333,0.966666666666667,
1.),.UNSPECIFIED.);
#539=B_SPLINE_CURVE_WITH_KNOTS('',5,(#38522,#38523,#38524,#38525,#38526,
#38527,#38528,#38529,#38530,#38531,#38532,#38533,#38534,#38535,#38536,#38537,
#38538,#38539,#38540,#38541,#38542,#38543,#38544,#38545,#38546,#38547,#38548,
#38549,#38550,#38551,#38552,#38553,#38554,#38555,#38556),.UNSPECIFIED.,
 .F.,.F.,(6,1,1,1,1,1,1,1,1,1,1,1,1,1,1,1,1,1,1,1,1,1,1,1,1,1,1,1,1,1,6),
(0.,0.0333333333333333,0.0666666666666667,0.1,0.133333333333333,0.166666666666667,
0.2,0.233333333333333,0.266666666666667,0.3,0.333333333333333,0.366666666666667,
0.4,0.433333333333333,0.466666666666667,0.5,0.533333333333333,0.566666666666667,
0.6,0.633333333333333,0.666666666666667,0.7,0.733333333333333,0.766666666666667,
0.8,0.833333333333333,0.866666666666667,0.9,0.933333333333333,0.966666666666667,
1.),.UNSPECIFIED.);
#540=B_SPLINE_CURVE_WITH_KNOTS('',5,(#38564,#38565,#38566,#38567,#38568,
#38569,#38570,#38571,#38572,#38573,#38574,#38575,#38576,#38577,#38578,#38579,
#38580,#38581,#38582,#38583,#38584,#38585,#38586,#38587,#38588,#38589,#38590,
#38591,#38592,#38593,#38594,#38595,#38596,#38597,#38598),.UNSPECIFIED.,
 .F.,.F.,(6,1,1,1,1,1,1,1,1,1,1,1,1,1,1,1,1,1,1,1,1,1,1,1,1,1,1,1,1,1,6),
(0.,0.0333333333333333,0.0666666666666667,0.1,0.133333333333333,0.166666666666667,
0.2,0.233333333333333,0.266666666666667,0.3,0.333333333333333,0.366666666666667,
0.4,0.433333333333333,0.466666666666667,0.5,0.533333333333333,0.566666666666667,
0.6,0.633333333333333,0.666666666666667,0.7,0.733333333333333,0.766666666666667,
0.8,0.833333333333333,0.866666666666667,0.9,0.933333333333333,0.966666666666667,
1.),.UNSPECIFIED.);
#541=B_SPLINE_CURVE_WITH_KNOTS('',5,(#38602,#38603,#38604,#38605,#38606,
#38607,#38608,#38609,#38610,#38611,#38612,#38613,#38614,#38615,#38616,#38617,
#38618,#38619,#38620,#38621,#38622,#38623,#38624,#38625,#38626,#38627,#38628,
#38629,#38630,#38631,#38632,#38633,#38634,#38635,#38636),.UNSPECIFIED.,
 .F.,.F.,(6,1,1,1,1,1,1,1,1,1,1,1,1,1,1,1,1,1,1,1,1,1,1,1,1,1,1,1,1,1,6),
(0.,0.0333333333333333,0.0666666666666667,0.1,0.133333333333333,0.166666666666667,
0.2,0.233333333333333,0.266666666666667,0.3,0.333333333333333,0.366666666666667,
0.4,0.433333333333333,0.466666666666667,0.5,0.533333333333333,0.566666666666667,
0.6,0.633333333333333,0.666666666666667,0.7,0.733333333333333,0.766666666666667,
0.8,0.833333333333333,0.866666666666667,0.9,0.933333333333333,0.966666666666667,
1.),.UNSPECIFIED.);
#542=B_SPLINE_CURVE_WITH_KNOTS('',5,(#38727,#38728,#38729,#38730,#38731,
#38732,#38733,#38734,#38735,#38736,#38737,#38738,#38739,#38740,#38741,#38742,
#38743,#38744,#38745,#38746,#38747,#38748,#38749,#38750,#38751,#38752,#38753,
#38754,#38755,#38756,#38757,#38758,#38759,#38760,#38761),.UNSPECIFIED.,
 .F.,.F.,(6,1,1,1,1,1,1,1,1,1,1,1,1,1,1,1,1,1,1,1,1,1,1,1,1,1,1,1,1,1,6),
(0.,0.0333333333333333,0.0666666666666667,0.1,0.133333333333333,0.166666666666667,
0.2,0.233333333333333,0.266666666666667,0.3,0.333333333333333,0.366666666666667,
0.4,0.433333333333333,0.466666666666667,0.5,0.533333333333333,0.566666666666667,
0.6,0.633333333333333,0.666666666666667,0.7,0.733333333333333,0.766666666666667,
0.8,0.833333333333333,0.866666666666667,0.9,0.933333333333333,0.966666666666667,
1.),.UNSPECIFIED.);
#543=B_SPLINE_CURVE_WITH_KNOTS('',5,(#38837,#38838,#38839,#38840,#38841,
#38842,#38843,#38844,#38845,#38846,#38847,#38848,#38849,#38850,#38851,#38852,
#38853,#38854,#38855,#38856,#38857,#38858,#38859,#38860,#38861,#38862,#38863,
#38864,#38865,#38866,#38867,#38868,#38869,#38870,#38871),.UNSPECIFIED.,
 .F.,.F.,(6,1,1,1,1,1,1,1,1,1,1,1,1,1,1,1,1,1,1,1,1,1,1,1,1,1,1,1,1,1,6),
(-1.,-0.966666666666667,-0.933333333333333,-0.9,-0.866666666666667,-0.833333333333333,
-0.8,-0.766666666666667,-0.733333333333333,-0.7,-0.666666666666667,-0.633333333333333,
-0.6,-0.566666666666667,-0.533333333333333,-0.5,-0.466666666666667,-0.433333333333333,
-0.4,-0.366666666666667,-0.333333333333333,-0.3,-0.266666666666667,-0.233333333333333,
-0.2,-0.166666666666667,-0.133333333333333,-0.1,-0.0666666666666667,-0.0333333333333333,
0.),.UNSPECIFIED.);
#544=B_SPLINE_CURVE_WITH_KNOTS('',5,(#38957,#38958,#38959,#38960,#38961,
#38962,#38963,#38964,#38965,#38966,#38967,#38968,#38969,#38970,#38971,#38972,
#38973,#38974,#38975,#38976,#38977,#38978,#38979,#38980,#38981,#38982,#38983,
#38984,#38985,#38986,#38987,#38988,#38989,#38990,#38991),.UNSPECIFIED.,
 .F.,.F.,(6,1,1,1,1,1,1,1,1,1,1,1,1,1,1,1,1,1,1,1,1,1,1,1,1,1,1,1,1,1,6),
(0.,0.0333333333333333,0.0666666666666667,0.1,0.133333333333333,0.166666666666667,
0.2,0.233333333333333,0.266666666666667,0.3,0.333333333333333,0.366666666666667,
0.4,0.433333333333333,0.466666666666667,0.5,0.533333333333333,0.566666666666667,
0.6,0.633333333333333,0.666666666666667,0.7,0.733333333333333,0.766666666666667,
0.8,0.833333333333333,0.866666666666667,0.9,0.933333333333333,0.966666666666667,
1.),.UNSPECIFIED.);
#545=B_SPLINE_CURVE_WITH_KNOTS('',5,(#39067,#39068,#39069,#39070,#39071,
#39072,#39073,#39074,#39075,#39076,#39077,#39078,#39079,#39080,#39081,#39082,
#39083,#39084,#39085,#39086,#39087,#39088,#39089,#39090,#39091,#39092,#39093,
#39094,#39095,#39096,#39097,#39098,#39099,#39100,#39101),.UNSPECIFIED.,
 .F.,.F.,(6,1,1,1,1,1,1,1,1,1,1,1,1,1,1,1,1,1,1,1,1,1,1,1,1,1,1,1,1,1,6),
(-1.,-0.966666666666667,-0.933333333333333,-0.9,-0.866666666666667,-0.833333333333333,
-0.8,-0.766666666666667,-0.733333333333333,-0.7,-0.666666666666667,-0.633333333333333,
-0.6,-0.566666666666667,-0.533333333333333,-0.5,-0.466666666666667,-0.433333333333333,
-0.4,-0.366666666666667,-0.333333333333333,-0.3,-0.266666666666667,-0.233333333333333,
-0.2,-0.166666666666667,-0.133333333333333,-0.1,-0.0666666666666667,-0.0333333333333333,
0.),.UNSPECIFIED.);
#546=B_SPLINE_CURVE_WITH_KNOTS('',5,(#39187,#39188,#39189,#39190,#39191,
#39192,#39193,#39194,#39195,#39196,#39197,#39198,#39199,#39200,#39201,#39202,
#39203,#39204,#39205,#39206,#39207,#39208,#39209,#39210,#39211,#39212,#39213,
#39214,#39215,#39216,#39217,#39218,#39219,#39220,#39221),.UNSPECIFIED.,
 .F.,.F.,(6,1,1,1,1,1,1,1,1,1,1,1,1,1,1,1,1,1,1,1,1,1,1,1,1,1,1,1,1,1,6),
(0.,0.0333333333333333,0.0666666666666667,0.1,0.133333333333333,0.166666666666667,
0.2,0.233333333333333,0.266666666666667,0.3,0.333333333333333,0.366666666666667,
0.4,0.433333333333333,0.466666666666667,0.5,0.533333333333333,0.566666666666667,
0.6,0.633333333333333,0.666666666666667,0.7,0.733333333333333,0.766666666666667,
0.8,0.833333333333333,0.866666666666667,0.9,0.933333333333333,0.966666666666667,
1.),.UNSPECIFIED.);
#547=B_SPLINE_CURVE_WITH_KNOTS('',5,(#39297,#39298,#39299,#39300,#39301,
#39302,#39303,#39304,#39305,#39306,#39307,#39308,#39309,#39310,#39311,#39312,
#39313,#39314,#39315,#39316,#39317,#39318,#39319,#39320,#39321,#39322,#39323,
#39324,#39325,#39326,#39327,#39328,#39329,#39330,#39331),.UNSPECIFIED.,
 .F.,.F.,(6,1,1,1,1,1,1,1,1,1,1,1,1,1,1,1,1,1,1,1,1,1,1,1,1,1,1,1,1,1,6),
(-1.,-0.966666666666667,-0.933333333333333,-0.9,-0.866666666666667,-0.833333333333333,
-0.8,-0.766666666666667,-0.733333333333333,-0.7,-0.666666666666667,-0.633333333333333,
-0.6,-0.566666666666667,-0.533333333333333,-0.5,-0.466666666666667,-0.433333333333333,
-0.4,-0.366666666666667,-0.333333333333333,-0.3,-0.266666666666667,-0.233333333333333,
-0.2,-0.166666666666667,-0.133333333333333,-0.1,-0.0666666666666667,-0.0333333333333333,
0.),.UNSPECIFIED.);
#548=B_SPLINE_CURVE_WITH_KNOTS('',5,(#39417,#39418,#39419,#39420,#39421,
#39422,#39423,#39424,#39425,#39426,#39427,#39428,#39429,#39430,#39431,#39432,
#39433,#39434,#39435,#39436,#39437,#39438,#39439,#39440,#39441,#39442,#39443,
#39444,#39445,#39446,#39447,#39448,#39449,#39450,#39451),.UNSPECIFIED.,
 .F.,.F.,(6,1,1,1,1,1,1,1,1,1,1,1,1,1,1,1,1,1,1,1,1,1,1,1,1,1,1,1,1,1,6),
(0.,0.0333333333333333,0.0666666666666667,0.1,0.133333333333333,0.166666666666667,
0.2,0.233333333333333,0.266666666666667,0.3,0.333333333333333,0.366666666666667,
0.4,0.433333333333333,0.466666666666667,0.5,0.533333333333333,0.566666666666667,
0.6,0.633333333333333,0.666666666666667,0.7,0.733333333333333,0.766666666666667,
0.8,0.833333333333333,0.866666666666667,0.9,0.933333333333333,0.966666666666667,
1.),.UNSPECIFIED.);
#549=B_SPLINE_CURVE_WITH_KNOTS('',5,(#39527,#39528,#39529,#39530,#39531,
#39532,#39533,#39534,#39535,#39536,#39537,#39538,#39539,#39540,#39541,#39542,
#39543,#39544,#39545,#39546,#39547,#39548,#39549,#39550,#39551,#39552,#39553,
#39554,#39555,#39556,#39557,#39558,#39559,#39560,#39561),.UNSPECIFIED.,
 .F.,.F.,(6,1,1,1,1,1,1,1,1,1,1,1,1,1,1,1,1,1,1,1,1,1,1,1,1,1,1,1,1,1,6),
(-1.,-0.966666666666667,-0.933333333333333,-0.9,-0.866666666666667,-0.833333333333333,
-0.8,-0.766666666666667,-0.733333333333333,-0.7,-0.666666666666667,-0.633333333333333,
-0.6,-0.566666666666667,-0.533333333333333,-0.5,-0.466666666666667,-0.433333333333333,
-0.4,-0.366666666666667,-0.333333333333333,-0.3,-0.266666666666667,-0.233333333333333,
-0.2,-0.166666666666667,-0.133333333333333,-0.1,-0.0666666666666667,-0.0333333333333333,
0.),.UNSPECIFIED.);
#550=B_SPLINE_CURVE_WITH_KNOTS('',5,(#39647,#39648,#39649,#39650,#39651,
#39652,#39653,#39654,#39655,#39656,#39657,#39658,#39659,#39660,#39661,#39662,
#39663,#39664,#39665,#39666,#39667,#39668,#39669,#39670,#39671,#39672,#39673,
#39674,#39675,#39676,#39677,#39678,#39679,#39680,#39681),.UNSPECIFIED.,
 .F.,.F.,(6,1,1,1,1,1,1,1,1,1,1,1,1,1,1,1,1,1,1,1,1,1,1,1,1,1,1,1,1,1,6),
(0.,0.0333333333333333,0.0666666666666667,0.1,0.133333333333333,0.166666666666667,
0.2,0.233333333333333,0.266666666666667,0.3,0.333333333333333,0.366666666666667,
0.4,0.433333333333333,0.466666666666667,0.5,0.533333333333333,0.566666666666667,
0.6,0.633333333333333,0.666666666666667,0.7,0.733333333333333,0.766666666666667,
0.8,0.833333333333333,0.866666666666667,0.9,0.933333333333333,0.966666666666667,
1.),.UNSPECIFIED.);
#551=B_SPLINE_CURVE_WITH_KNOTS('',5,(#39757,#39758,#39759,#39760,#39761,
#39762,#39763,#39764,#39765,#39766,#39767,#39768,#39769,#39770,#39771,#39772,
#39773,#39774,#39775,#39776,#39777,#39778,#39779,#39780,#39781,#39782,#39783,
#39784,#39785,#39786,#39787,#39788,#39789,#39790,#39791),.UNSPECIFIED.,
 .F.,.F.,(6,1,1,1,1,1,1,1,1,1,1,1,1,1,1,1,1,1,1,1,1,1,1,1,1,1,1,1,1,1,6),
(-1.,-0.966666666666667,-0.933333333333333,-0.9,-0.866666666666667,-0.833333333333333,
-0.8,-0.766666666666667,-0.733333333333333,-0.7,-0.666666666666667,-0.633333333333333,
-0.6,-0.566666666666667,-0.533333333333333,-0.5,-0.466666666666667,-0.433333333333333,
-0.4,-0.366666666666667,-0.333333333333333,-0.3,-0.266666666666667,-0.233333333333333,
-0.2,-0.166666666666667,-0.133333333333333,-0.1,-0.0666666666666667,-0.0333333333333333,
0.),.UNSPECIFIED.);
#552=B_SPLINE_CURVE_WITH_KNOTS('',5,(#39877,#39878,#39879,#39880,#39881,
#39882,#39883,#39884,#39885,#39886,#39887,#39888,#39889,#39890,#39891,#39892,
#39893,#39894,#39895,#39896,#39897,#39898,#39899,#39900,#39901,#39902,#39903,
#39904,#39905,#39906,#39907,#39908,#39909,#39910,#39911),.UNSPECIFIED.,
 .F.,.F.,(6,1,1,1,1,1,1,1,1,1,1,1,1,1,1,1,1,1,1,1,1,1,1,1,1,1,1,1,1,1,6),
(0.,0.0333333333333333,0.0666666666666667,0.1,0.133333333333333,0.166666666666667,
0.2,0.233333333333333,0.266666666666667,0.3,0.333333333333333,0.366666666666667,
0.4,0.433333333333333,0.466666666666667,0.5,0.533333333333333,0.566666666666667,
0.6,0.633333333333333,0.666666666666667,0.7,0.733333333333333,0.766666666666667,
0.8,0.833333333333333,0.866666666666667,0.9,0.933333333333333,0.966666666666667,
1.),.UNSPECIFIED.);
#553=B_SPLINE_CURVE_WITH_KNOTS('',5,(#39987,#39988,#39989,#39990,#39991,
#39992,#39993,#39994,#39995,#39996,#39997,#39998,#39999,#40000,#40001,#40002,
#40003,#40004,#40005,#40006,#40007,#40008,#40009,#40010,#40011,#40012,#40013,
#40014,#40015,#40016,#40017,#40018,#40019,#40020,#40021),.UNSPECIFIED.,
 .F.,.F.,(6,1,1,1,1,1,1,1,1,1,1,1,1,1,1,1,1,1,1,1,1,1,1,1,1,1,1,1,1,1,6),
(-1.,-0.966666666666667,-0.933333333333333,-0.9,-0.866666666666667,-0.833333333333333,
-0.8,-0.766666666666667,-0.733333333333333,-0.7,-0.666666666666667,-0.633333333333333,
-0.6,-0.566666666666667,-0.533333333333333,-0.5,-0.466666666666667,-0.433333333333333,
-0.4,-0.366666666666667,-0.333333333333333,-0.3,-0.266666666666667,-0.233333333333333,
-0.2,-0.166666666666667,-0.133333333333333,-0.1,-0.0666666666666667,-0.0333333333333333,
0.),.UNSPECIFIED.);
#554=B_SPLINE_CURVE_WITH_KNOTS('',5,(#40107,#40108,#40109,#40110,#40111,
#40112,#40113,#40114,#40115,#40116,#40117,#40118,#40119,#40120,#40121,#40122,
#40123,#40124,#40125,#40126,#40127,#40128,#40129,#40130,#40131,#40132,#40133,
#40134,#40135,#40136,#40137,#40138,#40139,#40140,#40141),.UNSPECIFIED.,
 .F.,.F.,(6,1,1,1,1,1,1,1,1,1,1,1,1,1,1,1,1,1,1,1,1,1,1,1,1,1,1,1,1,1,6),
(0.,0.0333333333333333,0.0666666666666667,0.1,0.133333333333333,0.166666666666667,
0.2,0.233333333333333,0.266666666666667,0.3,0.333333333333333,0.366666666666667,
0.4,0.433333333333333,0.466666666666667,0.5,0.533333333333333,0.566666666666667,
0.6,0.633333333333333,0.666666666666667,0.7,0.733333333333333,0.766666666666667,
0.8,0.833333333333333,0.866666666666667,0.9,0.933333333333333,0.966666666666667,
1.),.UNSPECIFIED.);
#555=B_SPLINE_CURVE_WITH_KNOTS('',5,(#40217,#40218,#40219,#40220,#40221,
#40222,#40223,#40224,#40225,#40226,#40227,#40228,#40229,#40230,#40231,#40232,
#40233,#40234,#40235,#40236,#40237,#40238,#40239,#40240,#40241,#40242,#40243,
#40244,#40245,#40246,#40247,#40248,#40249,#40250,#40251),.UNSPECIFIED.,
 .F.,.F.,(6,1,1,1,1,1,1,1,1,1,1,1,1,1,1,1,1,1,1,1,1,1,1,1,1,1,1,1,1,1,6),
(-1.,-0.966666666666667,-0.933333333333333,-0.9,-0.866666666666667,-0.833333333333333,
-0.8,-0.766666666666667,-0.733333333333333,-0.7,-0.666666666666667,-0.633333333333333,
-0.6,-0.566666666666667,-0.533333333333333,-0.5,-0.466666666666667,-0.433333333333333,
-0.4,-0.366666666666667,-0.333333333333333,-0.3,-0.266666666666667,-0.233333333333333,
-0.2,-0.166666666666667,-0.133333333333333,-0.1,-0.0666666666666667,-0.0333333333333333,
0.),.UNSPECIFIED.);
#556=B_SPLINE_CURVE_WITH_KNOTS('',5,(#40337,#40338,#40339,#40340,#40341,
#40342,#40343,#40344,#40345,#40346,#40347,#40348,#40349,#40350,#40351,#40352,
#40353,#40354,#40355,#40356,#40357,#40358,#40359,#40360,#40361,#40362,#40363,
#40364,#40365,#40366,#40367,#40368,#40369,#40370,#40371),.UNSPECIFIED.,
 .F.,.F.,(6,1,1,1,1,1,1,1,1,1,1,1,1,1,1,1,1,1,1,1,1,1,1,1,1,1,1,1,1,1,6),
(0.,0.0333333333333333,0.0666666666666667,0.1,0.133333333333333,0.166666666666667,
0.2,0.233333333333333,0.266666666666667,0.3,0.333333333333333,0.366666666666667,
0.4,0.433333333333333,0.466666666666667,0.5,0.533333333333333,0.566666666666667,
0.6,0.633333333333333,0.666666666666667,0.7,0.733333333333333,0.766666666666667,
0.8,0.833333333333333,0.866666666666667,0.9,0.933333333333333,0.966666666666667,
1.),.UNSPECIFIED.);
#557=B_SPLINE_CURVE_WITH_KNOTS('',5,(#40447,#40448,#40449,#40450,#40451,
#40452,#40453,#40454,#40455,#40456,#40457,#40458,#40459,#40460,#40461,#40462,
#40463,#40464,#40465,#40466,#40467,#40468,#40469,#40470,#40471,#40472,#40473,
#40474,#40475,#40476,#40477,#40478,#40479,#40480,#40481),.UNSPECIFIED.,
 .F.,.F.,(6,1,1,1,1,1,1,1,1,1,1,1,1,1,1,1,1,1,1,1,1,1,1,1,1,1,1,1,1,1,6),
(-1.,-0.966666666666667,-0.933333333333333,-0.9,-0.866666666666667,-0.833333333333333,
-0.8,-0.766666666666667,-0.733333333333333,-0.7,-0.666666666666667,-0.633333333333333,
-0.6,-0.566666666666667,-0.533333333333333,-0.5,-0.466666666666667,-0.433333333333333,
-0.4,-0.366666666666667,-0.333333333333333,-0.3,-0.266666666666667,-0.233333333333333,
-0.2,-0.166666666666667,-0.133333333333333,-0.1,-0.0666666666666667,-0.0333333333333333,
0.),.UNSPECIFIED.);
#558=B_SPLINE_CURVE_WITH_KNOTS('',5,(#40567,#40568,#40569,#40570,#40571,
#40572,#40573,#40574,#40575,#40576,#40577,#40578,#40579,#40580,#40581,#40582,
#40583,#40584,#40585,#40586,#40587,#40588,#40589,#40590,#40591,#40592,#40593,
#40594,#40595,#40596,#40597,#40598,#40599,#40600,#40601),.UNSPECIFIED.,
 .F.,.F.,(6,1,1,1,1,1,1,1,1,1,1,1,1,1,1,1,1,1,1,1,1,1,1,1,1,1,1,1,1,1,6),
(0.,0.0333333333333333,0.0666666666666667,0.1,0.133333333333333,0.166666666666667,
0.2,0.233333333333333,0.266666666666667,0.3,0.333333333333333,0.366666666666667,
0.4,0.433333333333333,0.466666666666667,0.5,0.533333333333333,0.566666666666667,
0.6,0.633333333333333,0.666666666666667,0.7,0.733333333333333,0.766666666666667,
0.8,0.833333333333333,0.866666666666667,0.9,0.933333333333333,0.966666666666667,
1.),.UNSPECIFIED.);
#559=B_SPLINE_CURVE_WITH_KNOTS('',5,(#40677,#40678,#40679,#40680,#40681,
#40682,#40683,#40684,#40685,#40686,#40687,#40688,#40689,#40690,#40691,#40692,
#40693,#40694,#40695,#40696,#40697,#40698,#40699,#40700,#40701,#40702,#40703,
#40704,#40705,#40706,#40707,#40708,#40709,#40710,#40711),.UNSPECIFIED.,
 .F.,.F.,(6,1,1,1,1,1,1,1,1,1,1,1,1,1,1,1,1,1,1,1,1,1,1,1,1,1,1,1,1,1,6),
(-1.,-0.966666666666667,-0.933333333333333,-0.9,-0.866666666666667,-0.833333333333333,
-0.8,-0.766666666666667,-0.733333333333333,-0.7,-0.666666666666667,-0.633333333333333,
-0.6,-0.566666666666667,-0.533333333333333,-0.5,-0.466666666666667,-0.433333333333333,
-0.4,-0.366666666666667,-0.333333333333333,-0.3,-0.266666666666667,-0.233333333333333,
-0.2,-0.166666666666667,-0.133333333333333,-0.1,-0.0666666666666667,-0.0333333333333333,
0.),.UNSPECIFIED.);
#560=B_SPLINE_CURVE_WITH_KNOTS('',5,(#40797,#40798,#40799,#40800,#40801,
#40802,#40803,#40804,#40805,#40806,#40807,#40808,#40809,#40810,#40811,#40812,
#40813,#40814,#40815,#40816,#40817,#40818,#40819,#40820,#40821,#40822,#40823,
#40824,#40825,#40826,#40827,#40828,#40829,#40830,#40831),.UNSPECIFIED.,
 .F.,.F.,(6,1,1,1,1,1,1,1,1,1,1,1,1,1,1,1,1,1,1,1,1,1,1,1,1,1,1,1,1,1,6),
(0.,0.0333333333333333,0.0666666666666667,0.1,0.133333333333333,0.166666666666667,
0.2,0.233333333333333,0.266666666666667,0.3,0.333333333333333,0.366666666666667,
0.4,0.433333333333333,0.466666666666667,0.5,0.533333333333333,0.566666666666667,
0.6,0.633333333333333,0.666666666666667,0.7,0.733333333333333,0.766666666666667,
0.8,0.833333333333333,0.866666666666667,0.9,0.933333333333333,0.966666666666667,
1.),.UNSPECIFIED.);
#561=B_SPLINE_CURVE_WITH_KNOTS('',5,(#40907,#40908,#40909,#40910,#40911,
#40912,#40913,#40914,#40915,#40916,#40917,#40918,#40919,#40920,#40921,#40922,
#40923,#40924,#40925,#40926,#40927,#40928,#40929,#40930,#40931,#40932,#40933,
#40934,#40935,#40936,#40937,#40938,#40939,#40940,#40941),.UNSPECIFIED.,
 .F.,.F.,(6,1,1,1,1,1,1,1,1,1,1,1,1,1,1,1,1,1,1,1,1,1,1,1,1,1,1,1,1,1,6),
(-1.,-0.966666666666667,-0.933333333333333,-0.9,-0.866666666666667,-0.833333333333333,
-0.8,-0.766666666666667,-0.733333333333333,-0.7,-0.666666666666667,-0.633333333333333,
-0.6,-0.566666666666667,-0.533333333333333,-0.5,-0.466666666666667,-0.433333333333333,
-0.4,-0.366666666666667,-0.333333333333333,-0.3,-0.266666666666667,-0.233333333333333,
-0.2,-0.166666666666667,-0.133333333333333,-0.1,-0.0666666666666667,-0.0333333333333333,
0.),.UNSPECIFIED.);
#562=B_SPLINE_CURVE_WITH_KNOTS('',5,(#41027,#41028,#41029,#41030,#41031,
#41032,#41033,#41034,#41035,#41036,#41037,#41038,#41039,#41040,#41041,#41042,
#41043,#41044,#41045,#41046,#41047,#41048,#41049,#41050,#41051,#41052,#41053,
#41054,#41055,#41056,#41057,#41058,#41059,#41060,#41061),.UNSPECIFIED.,
 .F.,.F.,(6,1,1,1,1,1,1,1,1,1,1,1,1,1,1,1,1,1,1,1,1,1,1,1,1,1,1,1,1,1,6),
(0.,0.0333333333333333,0.0666666666666667,0.1,0.133333333333333,0.166666666666667,
0.2,0.233333333333333,0.266666666666667,0.3,0.333333333333333,0.366666666666667,
0.4,0.433333333333333,0.466666666666667,0.5,0.533333333333333,0.566666666666667,
0.6,0.633333333333333,0.666666666666667,0.7,0.733333333333333,0.766666666666667,
0.8,0.833333333333333,0.866666666666667,0.9,0.933333333333333,0.966666666666667,
1.),.UNSPECIFIED.);
#563=B_SPLINE_CURVE_WITH_KNOTS('',5,(#41137,#41138,#41139,#41140,#41141,
#41142,#41143,#41144,#41145,#41146,#41147,#41148,#41149,#41150,#41151,#41152,
#41153,#41154,#41155,#41156,#41157,#41158,#41159,#41160,#41161,#41162,#41163,
#41164,#41165,#41166,#41167,#41168,#41169,#41170,#41171),.UNSPECIFIED.,
 .F.,.F.,(6,1,1,1,1,1,1,1,1,1,1,1,1,1,1,1,1,1,1,1,1,1,1,1,1,1,1,1,1,1,6),
(-1.,-0.966666666666667,-0.933333333333333,-0.9,-0.866666666666667,-0.833333333333333,
-0.8,-0.766666666666667,-0.733333333333333,-0.7,-0.666666666666667,-0.633333333333333,
-0.6,-0.566666666666667,-0.533333333333333,-0.5,-0.466666666666667,-0.433333333333333,
-0.4,-0.366666666666667,-0.333333333333333,-0.3,-0.266666666666667,-0.233333333333333,
-0.2,-0.166666666666667,-0.133333333333333,-0.1,-0.0666666666666667,-0.0333333333333333,
0.),.UNSPECIFIED.);
#564=B_SPLINE_CURVE_WITH_KNOTS('',5,(#41257,#41258,#41259,#41260,#41261,
#41262,#41263,#41264,#41265,#41266,#41267,#41268,#41269,#41270,#41271,#41272,
#41273,#41274,#41275,#41276,#41277,#41278,#41279,#41280,#41281,#41282,#41283,
#41284,#41285,#41286,#41287,#41288,#41289,#41290,#41291),.UNSPECIFIED.,
 .F.,.F.,(6,1,1,1,1,1,1,1,1,1,1,1,1,1,1,1,1,1,1,1,1,1,1,1,1,1,1,1,1,1,6),
(0.,0.0333333333333333,0.0666666666666667,0.1,0.133333333333333,0.166666666666667,
0.2,0.233333333333333,0.266666666666667,0.3,0.333333333333333,0.366666666666667,
0.4,0.433333333333333,0.466666666666667,0.5,0.533333333333333,0.566666666666667,
0.6,0.633333333333333,0.666666666666667,0.7,0.733333333333333,0.766666666666667,
0.8,0.833333333333333,0.866666666666667,0.9,0.933333333333333,0.966666666666667,
1.),.UNSPECIFIED.);
#565=B_SPLINE_CURVE_WITH_KNOTS('',5,(#41367,#41368,#41369,#41370,#41371,
#41372,#41373,#41374,#41375,#41376,#41377,#41378,#41379,#41380,#41381,#41382,
#41383,#41384,#41385,#41386,#41387,#41388,#41389,#41390,#41391,#41392,#41393,
#41394,#41395,#41396,#41397,#41398,#41399,#41400,#41401),.UNSPECIFIED.,
 .F.,.F.,(6,1,1,1,1,1,1,1,1,1,1,1,1,1,1,1,1,1,1,1,1,1,1,1,1,1,1,1,1,1,6),
(-1.,-0.966666666666667,-0.933333333333333,-0.9,-0.866666666666667,-0.833333333333333,
-0.8,-0.766666666666667,-0.733333333333333,-0.7,-0.666666666666667,-0.633333333333333,
-0.6,-0.566666666666667,-0.533333333333333,-0.5,-0.466666666666667,-0.433333333333333,
-0.4,-0.366666666666667,-0.333333333333333,-0.3,-0.266666666666667,-0.233333333333333,
-0.2,-0.166666666666667,-0.133333333333333,-0.1,-0.0666666666666667,-0.0333333333333333,
0.),.UNSPECIFIED.);
#566=B_SPLINE_CURVE_WITH_KNOTS('',5,(#41487,#41488,#41489,#41490,#41491,
#41492,#41493,#41494,#41495,#41496,#41497,#41498,#41499,#41500,#41501,#41502,
#41503,#41504,#41505,#41506,#41507,#41508,#41509,#41510,#41511,#41512,#41513,
#41514,#41515,#41516,#41517,#41518,#41519,#41520,#41521),.UNSPECIFIED.,
 .F.,.F.,(6,1,1,1,1,1,1,1,1,1,1,1,1,1,1,1,1,1,1,1,1,1,1,1,1,1,1,1,1,1,6),
(0.,0.0333333333333333,0.0666666666666667,0.1,0.133333333333333,0.166666666666667,
0.2,0.233333333333333,0.266666666666667,0.3,0.333333333333333,0.366666666666667,
0.4,0.433333333333333,0.466666666666667,0.5,0.533333333333333,0.566666666666667,
0.6,0.633333333333333,0.666666666666667,0.7,0.733333333333333,0.766666666666667,
0.8,0.833333333333333,0.866666666666667,0.9,0.933333333333333,0.966666666666667,
1.),.UNSPECIFIED.);
#567=B_SPLINE_CURVE_WITH_KNOTS('',5,(#41597,#41598,#41599,#41600,#41601,
#41602,#41603,#41604,#41605,#41606,#41607,#41608,#41609,#41610,#41611,#41612,
#41613,#41614,#41615,#41616,#41617,#41618,#41619,#41620,#41621,#41622,#41623,
#41624,#41625,#41626,#41627,#41628,#41629,#41630,#41631),.UNSPECIFIED.,
 .F.,.F.,(6,1,1,1,1,1,1,1,1,1,1,1,1,1,1,1,1,1,1,1,1,1,1,1,1,1,1,1,1,1,6),
(-1.,-0.966666666666667,-0.933333333333333,-0.9,-0.866666666666667,-0.833333333333333,
-0.8,-0.766666666666667,-0.733333333333333,-0.7,-0.666666666666667,-0.633333333333333,
-0.6,-0.566666666666667,-0.533333333333333,-0.5,-0.466666666666667,-0.433333333333333,
-0.4,-0.366666666666667,-0.333333333333333,-0.3,-0.266666666666667,-0.233333333333333,
-0.2,-0.166666666666667,-0.133333333333333,-0.1,-0.0666666666666667,-0.0333333333333333,
0.),.UNSPECIFIED.);
#568=B_SPLINE_CURVE_WITH_KNOTS('',5,(#41722,#41723,#41724,#41725,#41726,
#41727,#41728,#41729,#41730,#41731,#41732,#41733,#41734,#41735,#41736,#41737,
#41738,#41739,#41740,#41741,#41742,#41743,#41744,#41745,#41746,#41747,#41748,
#41749,#41750,#41751,#41752,#41753,#41754,#41755,#41756),.UNSPECIFIED.,
 .F.,.F.,(6,1,1,1,1,1,1,1,1,1,1,1,1,1,1,1,1,1,1,1,1,1,1,1,1,1,1,1,1,1,6),
(0.,0.0333333333333333,0.0666666666666667,0.1,0.133333333333333,0.166666666666667,
0.2,0.233333333333333,0.266666666666667,0.3,0.333333333333333,0.366666666666667,
0.4,0.433333333333333,0.466666666666667,0.5,0.533333333333333,0.566666666666667,
0.6,0.633333333333333,0.666666666666667,0.7,0.733333333333333,0.766666666666667,
0.8,0.833333333333333,0.866666666666667,0.9,0.933333333333333,0.966666666666667,
1.),.UNSPECIFIED.);
#569=B_SPLINE_CURVE_WITH_KNOTS('',5,(#41827,#41828,#41829,#41830,#41831,
#41832,#41833,#41834,#41835,#41836,#41837,#41838,#41839,#41840,#41841,#41842,
#41843,#41844,#41845,#41846,#41847,#41848,#41849,#41850,#41851,#41852,#41853,
#41854,#41855,#41856,#41857,#41858,#41859,#41860,#41861),.UNSPECIFIED.,
 .F.,.F.,(6,1,1,1,1,1,1,1,1,1,1,1,1,1,1,1,1,1,1,1,1,1,1,1,1,1,1,1,1,1,6),
(-1.,-0.966666666666667,-0.933333333333333,-0.9,-0.866666666666667,-0.833333333333333,
-0.8,-0.766666666666667,-0.733333333333333,-0.7,-0.666666666666667,-0.633333333333333,
-0.6,-0.566666666666667,-0.533333333333333,-0.5,-0.466666666666667,-0.433333333333333,
-0.4,-0.366666666666667,-0.333333333333333,-0.3,-0.266666666666667,-0.233333333333333,
-0.2,-0.166666666666667,-0.133333333333333,-0.1,-0.0666666666666667,-0.0333333333333333,
0.),.UNSPECIFIED.);
#570=B_SPLINE_CURVE_WITH_KNOTS('',5,(#41868,#41869,#41870,#41871,#41872,
#41873,#41874,#41875,#41876,#41877,#41878,#41879,#41880,#41881,#41882,#41883,
#41884,#41885,#41886,#41887,#41888,#41889,#41890,#41891,#41892,#41893,#41894,
#41895,#41896,#41897,#41898,#41899,#41900,#41901,#41902),.UNSPECIFIED.,
 .F.,.F.,(6,1,1,1,1,1,1,1,1,1,1,1,1,1,1,1,1,1,1,1,1,1,1,1,1,1,1,1,1,1,6),
(0.,0.0333333333333333,0.0666666666666667,0.1,0.133333333333333,0.166666666666667,
0.2,0.233333333333333,0.266666666666667,0.3,0.333333333333333,0.366666666666667,
0.4,0.433333333333333,0.466666666666667,0.5,0.533333333333333,0.566666666666667,
0.6,0.633333333333333,0.666666666666667,0.7,0.733333333333333,0.766666666666667,
0.8,0.833333333333333,0.866666666666667,0.9,0.933333333333333,0.966666666666667,
1.),.UNSPECIFIED.);
#571=B_SPLINE_CURVE_WITH_KNOTS('',5,(#41906,#41907,#41908,#41909,#41910,
#41911,#41912,#41913,#41914,#41915,#41916,#41917,#41918,#41919,#41920,#41921,
#41922,#41923,#41924,#41925,#41926,#41927,#41928,#41929,#41930,#41931,#41932,
#41933,#41934,#41935,#41936,#41937,#41938,#41939,#41940),.UNSPECIFIED.,
 .F.,.F.,(6,1,1,1,1,1,1,1,1,1,1,1,1,1,1,1,1,1,1,1,1,1,1,1,1,1,1,1,1,1,6),
(-1.,-0.966666666666667,-0.933333333333333,-0.9,-0.866666666666667,-0.833333333333333,
-0.8,-0.766666666666667,-0.733333333333333,-0.7,-0.666666666666667,-0.633333333333333,
-0.6,-0.566666666666667,-0.533333333333333,-0.5,-0.466666666666667,-0.433333333333333,
-0.4,-0.366666666666667,-0.333333333333333,-0.3,-0.266666666666667,-0.233333333333333,
-0.2,-0.166666666666667,-0.133333333333333,-0.1,-0.0666666666666667,-0.0333333333333333,
0.),.UNSPECIFIED.);
#865=B_SPLINE_SURFACE_WITH_KNOTS('',5,1,((#37149,#37150),(#37151,#37152),
(#37153,#37154),(#37155,#37156),(#37157,#37158),(#37159,#37160),(#37161,
#37162),(#37163,#37164),(#37165,#37166),(#37167,#37168),(#37169,#37170),
(#37171,#37172),(#37173,#37174),(#37175,#37176),(#37177,#37178),(#37179,
#37180),(#37181,#37182),(#37183,#37184),(#37185,#37186),(#37187,#37188),
(#37189,#37190),(#37191,#37192),(#37193,#37194),(#37195,#37196),(#37197,
#37198),(#37199,#37200),(#37201,#37202),(#37203,#37204),(#37205,#37206),
(#37207,#37208),(#37209,#37210),(#37211,#37212),(#37213,#37214),(#37215,
#37216),(#37217,#37218)),.UNSPECIFIED.,.F.,.F.,.F.,(6,1,1,1,1,1,1,1,1,1,
1,1,1,1,1,1,1,1,1,1,1,1,1,1,1,1,1,1,1,1,6),(2,2),(0.,0.0333333333333333,
0.0666666666666667,0.1,0.133333333333333,0.166666666666667,0.2,0.233333333333333,
0.266666666666667,0.3,0.333333333333333,0.366666666666667,0.4,0.433333333333333,
0.466666666666667,0.5,0.533333333333333,0.566666666666667,0.6,0.633333333333333,
0.666666666666667,0.7,0.733333333333333,0.766666666666667,0.8,0.833333333333333,
0.866666666666667,0.9,0.933333333333333,0.966666666666667,1.),(0.,0.762),
 .UNSPECIFIED.);
#866=B_SPLINE_SURFACE_WITH_KNOTS('',5,1,((#37298,#37299),(#37300,#37301),
(#37302,#37303),(#37304,#37305),(#37306,#37307),(#37308,#37309),(#37310,
#37311),(#37312,#37313),(#37314,#37315),(#37316,#37317),(#37318,#37319),
(#37320,#37321),(#37322,#37323),(#37324,#37325),(#37326,#37327),(#37328,
#37329),(#37330,#37331),(#37332,#37333),(#37334,#37335),(#37336,#37337),
(#37338,#37339),(#37340,#37341),(#37342,#37343),(#37344,#37345),(#37346,
#37347),(#37348,#37349),(#37350,#37351),(#37352,#37353),(#37354,#37355),
(#37356,#37357),(#37358,#37359),(#37360,#37361),(#37362,#37363),(#37364,
#37365),(#37366,#37367)),.UNSPECIFIED.,.F.,.F.,.F.,(6,1,1,1,1,1,1,1,1,1,
1,1,1,1,1,1,1,1,1,1,1,1,1,1,1,1,1,1,1,1,6),(2,2),(-1.,-0.966666666666667,
-0.933333333333333,-0.9,-0.866666666666667,-0.833333333333333,-0.8,-0.766666666666667,
-0.733333333333333,-0.7,-0.666666666666667,-0.633333333333333,-0.6,-0.566666666666667,
-0.533333333333333,-0.5,-0.466666666666667,-0.433333333333333,-0.4,-0.366666666666667,
-0.333333333333333,-0.3,-0.266666666666667,-0.233333333333333,-0.2,-0.166666666666667,
-0.133333333333333,-0.1,-0.0666666666666667,-0.0333333333333333,0.),(0.,
0.762),.UNSPECIFIED.);
#867=B_SPLINE_SURFACE_WITH_KNOTS('',5,1,((#38656,#38657),(#38658,#38659),
(#38660,#38661),(#38662,#38663),(#38664,#38665),(#38666,#38667),(#38668,
#38669),(#38670,#38671),(#38672,#38673),(#38674,#38675),(#38676,#38677),
(#38678,#38679),(#38680,#38681),(#38682,#38683),(#38684,#38685),(#38686,
#38687),(#38688,#38689),(#38690,#38691),(#38692,#38693),(#38694,#38695),
(#38696,#38697),(#38698,#38699),(#38700,#38701),(#38702,#38703),(#38704,
#38705),(#38706,#38707),(#38708,#38709),(#38710,#38711),(#38712,#38713),
(#38714,#38715),(#38716,#38717),(#38718,#38719),(#38720,#38721),(#38722,
#38723),(#38724,#38725)),.UNSPECIFIED.,.F.,.F.,.F.,(6,1,1,1,1,1,1,1,1,1,
1,1,1,1,1,1,1,1,1,1,1,1,1,1,1,1,1,1,1,1,6),(2,2),(0.,0.0333333333333333,
0.0666666666666667,0.1,0.133333333333333,0.166666666666667,0.2,0.233333333333333,
0.266666666666667,0.3,0.333333333333333,0.366666666666667,0.4,0.433333333333333,
0.466666666666667,0.5,0.533333333333333,0.566666666666667,0.6,0.633333333333333,
0.666666666666667,0.7,0.733333333333333,0.766666666666667,0.8,0.833333333333333,
0.866666666666667,0.9,0.933333333333333,0.966666666666667,1.),(0.,0.762),
 .UNSPECIFIED.);
#868=B_SPLINE_SURFACE_WITH_KNOTS('',5,1,((#38767,#38768),(#38769,#38770),
(#38771,#38772),(#38773,#38774),(#38775,#38776),(#38777,#38778),(#38779,
#38780),(#38781,#38782),(#38783,#38784),(#38785,#38786),(#38787,#38788),
(#38789,#38790),(#38791,#38792),(#38793,#38794),(#38795,#38796),(#38797,
#38798),(#38799,#38800),(#38801,#38802),(#38803,#38804),(#38805,#38806),
(#38807,#38808),(#38809,#38810),(#38811,#38812),(#38813,#38814),(#38815,
#38816),(#38817,#38818),(#38819,#38820),(#38821,#38822),(#38823,#38824),
(#38825,#38826),(#38827,#38828),(#38829,#38830),(#38831,#38832),(#38833,
#38834),(#38835,#38836)),.UNSPECIFIED.,.F.,.F.,.F.,(6,1,1,1,1,1,1,1,1,1,
1,1,1,1,1,1,1,1,1,1,1,1,1,1,1,1,1,1,1,1,6),(2,2),(-1.,-0.966666666666667,
-0.933333333333333,-0.9,-0.866666666666667,-0.833333333333333,-0.8,-0.766666666666667,
-0.733333333333333,-0.7,-0.666666666666667,-0.633333333333333,-0.6,-0.566666666666667,
-0.533333333333333,-0.5,-0.466666666666667,-0.433333333333333,-0.4,-0.366666666666667,
-0.333333333333333,-0.3,-0.266666666666667,-0.233333333333333,-0.2,-0.166666666666667,
-0.133333333333333,-0.1,-0.0666666666666667,-0.0333333333333333,0.),(0.,
0.762),.UNSPECIFIED.);
#869=B_SPLINE_SURFACE_WITH_KNOTS('',5,1,((#38886,#38887),(#38888,#38889),
(#38890,#38891),(#38892,#38893),(#38894,#38895),(#38896,#38897),(#38898,
#38899),(#38900,#38901),(#38902,#38903),(#38904,#38905),(#38906,#38907),
(#38908,#38909),(#38910,#38911),(#38912,#38913),(#38914,#38915),(#38916,
#38917),(#38918,#38919),(#38920,#38921),(#38922,#38923),(#38924,#38925),
(#38926,#38927),(#38928,#38929),(#38930,#38931),(#38932,#38933),(#38934,
#38935),(#38936,#38937),(#38938,#38939),(#38940,#38941),(#38942,#38943),
(#38944,#38945),(#38946,#38947),(#38948,#38949),(#38950,#38951),(#38952,
#38953),(#38954,#38955)),.UNSPECIFIED.,.F.,.F.,.F.,(6,1,1,1,1,1,1,1,1,1,
1,1,1,1,1,1,1,1,1,1,1,1,1,1,1,1,1,1,1,1,6),(2,2),(0.,0.0333333333333333,
0.0666666666666667,0.1,0.133333333333333,0.166666666666667,0.2,0.233333333333333,
0.266666666666667,0.3,0.333333333333333,0.366666666666667,0.4,0.433333333333333,
0.466666666666667,0.5,0.533333333333333,0.566666666666667,0.6,0.633333333333333,
0.666666666666667,0.7,0.733333333333333,0.766666666666667,0.8,0.833333333333333,
0.866666666666667,0.9,0.933333333333333,0.966666666666667,1.),(0.,0.762),
 .UNSPECIFIED.);
#870=B_SPLINE_SURFACE_WITH_KNOTS('',5,1,((#38997,#38998),(#38999,#39000),
(#39001,#39002),(#39003,#39004),(#39005,#39006),(#39007,#39008),(#39009,
#39010),(#39011,#39012),(#39013,#39014),(#39015,#39016),(#39017,#39018),
(#39019,#39020),(#39021,#39022),(#39023,#39024),(#39025,#39026),(#39027,
#39028),(#39029,#39030),(#39031,#39032),(#39033,#39034),(#39035,#39036),
(#39037,#39038),(#39039,#39040),(#39041,#39042),(#39043,#39044),(#39045,
#39046),(#39047,#39048),(#39049,#39050),(#39051,#39052),(#39053,#39054),
(#39055,#39056),(#39057,#39058),(#39059,#39060),(#39061,#39062),(#39063,
#39064),(#39065,#39066)),.UNSPECIFIED.,.F.,.F.,.F.,(6,1,1,1,1,1,1,1,1,1,
1,1,1,1,1,1,1,1,1,1,1,1,1,1,1,1,1,1,1,1,6),(2,2),(-1.,-0.966666666666667,
-0.933333333333333,-0.9,-0.866666666666667,-0.833333333333333,-0.8,-0.766666666666667,
-0.733333333333333,-0.7,-0.666666666666667,-0.633333333333333,-0.6,-0.566666666666667,
-0.533333333333333,-0.5,-0.466666666666667,-0.433333333333333,-0.4,-0.366666666666667,
-0.333333333333333,-0.3,-0.266666666666667,-0.233333333333333,-0.2,-0.166666666666667,
-0.133333333333333,-0.1,-0.0666666666666667,-0.0333333333333333,0.),(0.,
0.762),.UNSPECIFIED.);
#871=B_SPLINE_SURFACE_WITH_KNOTS('',5,1,((#39116,#39117),(#39118,#39119),
(#39120,#39121),(#39122,#39123),(#39124,#39125),(#39126,#39127),(#39128,
#39129),(#39130,#39131),(#39132,#39133),(#39134,#39135),(#39136,#39137),
(#39138,#39139),(#39140,#39141),(#39142,#39143),(#39144,#39145),(#39146,
#39147),(#39148,#39149),(#39150,#39151),(#39152,#39153),(#39154,#39155),
(#39156,#39157),(#39158,#39159),(#39160,#39161),(#39162,#39163),(#39164,
#39165),(#39166,#39167),(#39168,#39169),(#39170,#39171),(#39172,#39173),
(#39174,#39175),(#39176,#39177),(#39178,#39179),(#39180,#39181),(#39182,
#39183),(#39184,#39185)),.UNSPECIFIED.,.F.,.F.,.F.,(6,1,1,1,1,1,1,1,1,1,
1,1,1,1,1,1,1,1,1,1,1,1,1,1,1,1,1,1,1,1,6),(2,2),(0.,0.0333333333333333,
0.0666666666666667,0.1,0.133333333333333,0.166666666666667,0.2,0.233333333333333,
0.266666666666667,0.3,0.333333333333333,0.366666666666667,0.4,0.433333333333333,
0.466666666666667,0.5,0.533333333333333,0.566666666666667,0.6,0.633333333333333,
0.666666666666667,0.7,0.733333333333333,0.766666666666667,0.8,0.833333333333333,
0.866666666666667,0.9,0.933333333333333,0.966666666666667,1.),(0.,0.762),
 .UNSPECIFIED.);
#872=B_SPLINE_SURFACE_WITH_KNOTS('',5,1,((#39227,#39228),(#39229,#39230),
(#39231,#39232),(#39233,#39234),(#39235,#39236),(#39237,#39238),(#39239,
#39240),(#39241,#39242),(#39243,#39244),(#39245,#39246),(#39247,#39248),
(#39249,#39250),(#39251,#39252),(#39253,#39254),(#39255,#39256),(#39257,
#39258),(#39259,#39260),(#39261,#39262),(#39263,#39264),(#39265,#39266),
(#39267,#39268),(#39269,#39270),(#39271,#39272),(#39273,#39274),(#39275,
#39276),(#39277,#39278),(#39279,#39280),(#39281,#39282),(#39283,#39284),
(#39285,#39286),(#39287,#39288),(#39289,#39290),(#39291,#39292),(#39293,
#39294),(#39295,#39296)),.UNSPECIFIED.,.F.,.F.,.F.,(6,1,1,1,1,1,1,1,1,1,
1,1,1,1,1,1,1,1,1,1,1,1,1,1,1,1,1,1,1,1,6),(2,2),(-1.,-0.966666666666667,
-0.933333333333333,-0.9,-0.866666666666667,-0.833333333333333,-0.8,-0.766666666666667,
-0.733333333333333,-0.7,-0.666666666666667,-0.633333333333333,-0.6,-0.566666666666667,
-0.533333333333333,-0.5,-0.466666666666667,-0.433333333333333,-0.4,-0.366666666666667,
-0.333333333333333,-0.3,-0.266666666666667,-0.233333333333333,-0.2,-0.166666666666667,
-0.133333333333333,-0.1,-0.0666666666666667,-0.0333333333333333,0.),(0.,
0.762),.UNSPECIFIED.);
#873=B_SPLINE_SURFACE_WITH_KNOTS('',5,1,((#39346,#39347),(#39348,#39349),
(#39350,#39351),(#39352,#39353),(#39354,#39355),(#39356,#39357),(#39358,
#39359),(#39360,#39361),(#39362,#39363),(#39364,#39365),(#39366,#39367),
(#39368,#39369),(#39370,#39371),(#39372,#39373),(#39374,#39375),(#39376,
#39377),(#39378,#39379),(#39380,#39381),(#39382,#39383),(#39384,#39385),
(#39386,#39387),(#39388,#39389),(#39390,#39391),(#39392,#39393),(#39394,
#39395),(#39396,#39397),(#39398,#39399),(#39400,#39401),(#39402,#39403),
(#39404,#39405),(#39406,#39407),(#39408,#39409),(#39410,#39411),(#39412,
#39413),(#39414,#39415)),.UNSPECIFIED.,.F.,.F.,.F.,(6,1,1,1,1,1,1,1,1,1,
1,1,1,1,1,1,1,1,1,1,1,1,1,1,1,1,1,1,1,1,6),(2,2),(0.,0.0333333333333333,
0.0666666666666667,0.1,0.133333333333333,0.166666666666667,0.2,0.233333333333333,
0.266666666666667,0.3,0.333333333333333,0.366666666666667,0.4,0.433333333333333,
0.466666666666667,0.5,0.533333333333333,0.566666666666667,0.6,0.633333333333333,
0.666666666666667,0.7,0.733333333333333,0.766666666666667,0.8,0.833333333333333,
0.866666666666667,0.9,0.933333333333333,0.966666666666667,1.),(0.,0.762),
 .UNSPECIFIED.);
#874=B_SPLINE_SURFACE_WITH_KNOTS('',5,1,((#39457,#39458),(#39459,#39460),
(#39461,#39462),(#39463,#39464),(#39465,#39466),(#39467,#39468),(#39469,
#39470),(#39471,#39472),(#39473,#39474),(#39475,#39476),(#39477,#39478),
(#39479,#39480),(#39481,#39482),(#39483,#39484),(#39485,#39486),(#39487,
#39488),(#39489,#39490),(#39491,#39492),(#39493,#39494),(#39495,#39496),
(#39497,#39498),(#39499,#39500),(#39501,#39502),(#39503,#39504),(#39505,
#39506),(#39507,#39508),(#39509,#39510),(#39511,#39512),(#39513,#39514),
(#39515,#39516),(#39517,#39518),(#39519,#39520),(#39521,#39522),(#39523,
#39524),(#39525,#39526)),.UNSPECIFIED.,.F.,.F.,.F.,(6,1,1,1,1,1,1,1,1,1,
1,1,1,1,1,1,1,1,1,1,1,1,1,1,1,1,1,1,1,1,6),(2,2),(-1.,-0.966666666666667,
-0.933333333333333,-0.9,-0.866666666666667,-0.833333333333333,-0.8,-0.766666666666667,
-0.733333333333333,-0.7,-0.666666666666667,-0.633333333333333,-0.6,-0.566666666666667,
-0.533333333333333,-0.5,-0.466666666666667,-0.433333333333333,-0.4,-0.366666666666667,
-0.333333333333333,-0.3,-0.266666666666667,-0.233333333333333,-0.2,-0.166666666666667,
-0.133333333333333,-0.1,-0.0666666666666667,-0.0333333333333333,0.),(0.,
0.762),.UNSPECIFIED.);
#875=B_SPLINE_SURFACE_WITH_KNOTS('',5,1,((#39576,#39577),(#39578,#39579),
(#39580,#39581),(#39582,#39583),(#39584,#39585),(#39586,#39587),(#39588,
#39589),(#39590,#39591),(#39592,#39593),(#39594,#39595),(#39596,#39597),
(#39598,#39599),(#39600,#39601),(#39602,#39603),(#39604,#39605),(#39606,
#39607),(#39608,#39609),(#39610,#39611),(#39612,#39613),(#39614,#39615),
(#39616,#39617),(#39618,#39619),(#39620,#39621),(#39622,#39623),(#39624,
#39625),(#39626,#39627),(#39628,#39629),(#39630,#39631),(#39632,#39633),
(#39634,#39635),(#39636,#39637),(#39638,#39639),(#39640,#39641),(#39642,
#39643),(#39644,#39645)),.UNSPECIFIED.,.F.,.F.,.F.,(6,1,1,1,1,1,1,1,1,1,
1,1,1,1,1,1,1,1,1,1,1,1,1,1,1,1,1,1,1,1,6),(2,2),(0.,0.0333333333333333,
0.0666666666666667,0.1,0.133333333333333,0.166666666666667,0.2,0.233333333333333,
0.266666666666667,0.3,0.333333333333333,0.366666666666667,0.4,0.433333333333333,
0.466666666666667,0.5,0.533333333333333,0.566666666666667,0.6,0.633333333333333,
0.666666666666667,0.7,0.733333333333333,0.766666666666667,0.8,0.833333333333333,
0.866666666666667,0.9,0.933333333333333,0.966666666666667,1.),(0.,0.762),
 .UNSPECIFIED.);
#876=B_SPLINE_SURFACE_WITH_KNOTS('',5,1,((#39687,#39688),(#39689,#39690),
(#39691,#39692),(#39693,#39694),(#39695,#39696),(#39697,#39698),(#39699,
#39700),(#39701,#39702),(#39703,#39704),(#39705,#39706),(#39707,#39708),
(#39709,#39710),(#39711,#39712),(#39713,#39714),(#39715,#39716),(#39717,
#39718),(#39719,#39720),(#39721,#39722),(#39723,#39724),(#39725,#39726),
(#39727,#39728),(#39729,#39730),(#39731,#39732),(#39733,#39734),(#39735,
#39736),(#39737,#39738),(#39739,#39740),(#39741,#39742),(#39743,#39744),
(#39745,#39746),(#39747,#39748),(#39749,#39750),(#39751,#39752),(#39753,
#39754),(#39755,#39756)),.UNSPECIFIED.,.F.,.F.,.F.,(6,1,1,1,1,1,1,1,1,1,
1,1,1,1,1,1,1,1,1,1,1,1,1,1,1,1,1,1,1,1,6),(2,2),(-1.,-0.966666666666667,
-0.933333333333333,-0.9,-0.866666666666667,-0.833333333333333,-0.8,-0.766666666666667,
-0.733333333333333,-0.7,-0.666666666666667,-0.633333333333333,-0.6,-0.566666666666667,
-0.533333333333333,-0.5,-0.466666666666667,-0.433333333333333,-0.4,-0.366666666666667,
-0.333333333333333,-0.3,-0.266666666666667,-0.233333333333333,-0.2,-0.166666666666667,
-0.133333333333333,-0.1,-0.0666666666666667,-0.0333333333333333,0.),(0.,
0.762),.UNSPECIFIED.);
#877=B_SPLINE_SURFACE_WITH_KNOTS('',5,1,((#39806,#39807),(#39808,#39809),
(#39810,#39811),(#39812,#39813),(#39814,#39815),(#39816,#39817),(#39818,
#39819),(#39820,#39821),(#39822,#39823),(#39824,#39825),(#39826,#39827),
(#39828,#39829),(#39830,#39831),(#39832,#39833),(#39834,#39835),(#39836,
#39837),(#39838,#39839),(#39840,#39841),(#39842,#39843),(#39844,#39845),
(#39846,#39847),(#39848,#39849),(#39850,#39851),(#39852,#39853),(#39854,
#39855),(#39856,#39857),(#39858,#39859),(#39860,#39861),(#39862,#39863),
(#39864,#39865),(#39866,#39867),(#39868,#39869),(#39870,#39871),(#39872,
#39873),(#39874,#39875)),.UNSPECIFIED.,.F.,.F.,.F.,(6,1,1,1,1,1,1,1,1,1,
1,1,1,1,1,1,1,1,1,1,1,1,1,1,1,1,1,1,1,1,6),(2,2),(0.,0.0333333333333333,
0.0666666666666667,0.1,0.133333333333333,0.166666666666667,0.2,0.233333333333333,
0.266666666666667,0.3,0.333333333333333,0.366666666666667,0.4,0.433333333333333,
0.466666666666667,0.5,0.533333333333333,0.566666666666667,0.6,0.633333333333333,
0.666666666666667,0.7,0.733333333333333,0.766666666666667,0.8,0.833333333333333,
0.866666666666667,0.9,0.933333333333333,0.966666666666667,1.),(0.,0.762),
 .UNSPECIFIED.);
#878=B_SPLINE_SURFACE_WITH_KNOTS('',5,1,((#39917,#39918),(#39919,#39920),
(#39921,#39922),(#39923,#39924),(#39925,#39926),(#39927,#39928),(#39929,
#39930),(#39931,#39932),(#39933,#39934),(#39935,#39936),(#39937,#39938),
(#39939,#39940),(#39941,#39942),(#39943,#39944),(#39945,#39946),(#39947,
#39948),(#39949,#39950),(#39951,#39952),(#39953,#39954),(#39955,#39956),
(#39957,#39958),(#39959,#39960),(#39961,#39962),(#39963,#39964),(#39965,
#39966),(#39967,#39968),(#39969,#39970),(#39971,#39972),(#39973,#39974),
(#39975,#39976),(#39977,#39978),(#39979,#39980),(#39981,#39982),(#39983,
#39984),(#39985,#39986)),.UNSPECIFIED.,.F.,.F.,.F.,(6,1,1,1,1,1,1,1,1,1,
1,1,1,1,1,1,1,1,1,1,1,1,1,1,1,1,1,1,1,1,6),(2,2),(-1.,-0.966666666666667,
-0.933333333333333,-0.9,-0.866666666666667,-0.833333333333333,-0.8,-0.766666666666667,
-0.733333333333333,-0.7,-0.666666666666667,-0.633333333333333,-0.6,-0.566666666666667,
-0.533333333333333,-0.5,-0.466666666666667,-0.433333333333333,-0.4,-0.366666666666667,
-0.333333333333333,-0.3,-0.266666666666667,-0.233333333333333,-0.2,-0.166666666666667,
-0.133333333333333,-0.1,-0.0666666666666667,-0.0333333333333333,0.),(0.,
0.762),.UNSPECIFIED.);
#879=B_SPLINE_SURFACE_WITH_KNOTS('',5,1,((#40036,#40037),(#40038,#40039),
(#40040,#40041),(#40042,#40043),(#40044,#40045),(#40046,#40047),(#40048,
#40049),(#40050,#40051),(#40052,#40053),(#40054,#40055),(#40056,#40057),
(#40058,#40059),(#40060,#40061),(#40062,#40063),(#40064,#40065),(#40066,
#40067),(#40068,#40069),(#40070,#40071),(#40072,#40073),(#40074,#40075),
(#40076,#40077),(#40078,#40079),(#40080,#40081),(#40082,#40083),(#40084,
#40085),(#40086,#40087),(#40088,#40089),(#40090,#40091),(#40092,#40093),
(#40094,#40095),(#40096,#40097),(#40098,#40099),(#40100,#40101),(#40102,
#40103),(#40104,#40105)),.UNSPECIFIED.,.F.,.F.,.F.,(6,1,1,1,1,1,1,1,1,1,
1,1,1,1,1,1,1,1,1,1,1,1,1,1,1,1,1,1,1,1,6),(2,2),(0.,0.0333333333333333,
0.0666666666666667,0.1,0.133333333333333,0.166666666666667,0.2,0.233333333333333,
0.266666666666667,0.3,0.333333333333333,0.366666666666667,0.4,0.433333333333333,
0.466666666666667,0.5,0.533333333333333,0.566666666666667,0.6,0.633333333333333,
0.666666666666667,0.7,0.733333333333333,0.766666666666667,0.8,0.833333333333333,
0.866666666666667,0.9,0.933333333333333,0.966666666666667,1.),(0.,0.762),
 .UNSPECIFIED.);
#880=B_SPLINE_SURFACE_WITH_KNOTS('',5,1,((#40147,#40148),(#40149,#40150),
(#40151,#40152),(#40153,#40154),(#40155,#40156),(#40157,#40158),(#40159,
#40160),(#40161,#40162),(#40163,#40164),(#40165,#40166),(#40167,#40168),
(#40169,#40170),(#40171,#40172),(#40173,#40174),(#40175,#40176),(#40177,
#40178),(#40179,#40180),(#40181,#40182),(#40183,#40184),(#40185,#40186),
(#40187,#40188),(#40189,#40190),(#40191,#40192),(#40193,#40194),(#40195,
#40196),(#40197,#40198),(#40199,#40200),(#40201,#40202),(#40203,#40204),
(#40205,#40206),(#40207,#40208),(#40209,#40210),(#40211,#40212),(#40213,
#40214),(#40215,#40216)),.UNSPECIFIED.,.F.,.F.,.F.,(6,1,1,1,1,1,1,1,1,1,
1,1,1,1,1,1,1,1,1,1,1,1,1,1,1,1,1,1,1,1,6),(2,2),(-1.,-0.966666666666667,
-0.933333333333333,-0.9,-0.866666666666667,-0.833333333333333,-0.8,-0.766666666666667,
-0.733333333333333,-0.7,-0.666666666666667,-0.633333333333333,-0.6,-0.566666666666667,
-0.533333333333333,-0.5,-0.466666666666667,-0.433333333333333,-0.4,-0.366666666666667,
-0.333333333333333,-0.3,-0.266666666666667,-0.233333333333333,-0.2,-0.166666666666667,
-0.133333333333333,-0.1,-0.0666666666666667,-0.0333333333333333,0.),(0.,
0.762),.UNSPECIFIED.);
#881=B_SPLINE_SURFACE_WITH_KNOTS('',5,1,((#40266,#40267),(#40268,#40269),
(#40270,#40271),(#40272,#40273),(#40274,#40275),(#40276,#40277),(#40278,
#40279),(#40280,#40281),(#40282,#40283),(#40284,#40285),(#40286,#40287),
(#40288,#40289),(#40290,#40291),(#40292,#40293),(#40294,#40295),(#40296,
#40297),(#40298,#40299),(#40300,#40301),(#40302,#40303),(#40304,#40305),
(#40306,#40307),(#40308,#40309),(#40310,#40311),(#40312,#40313),(#40314,
#40315),(#40316,#40317),(#40318,#40319),(#40320,#40321),(#40322,#40323),
(#40324,#40325),(#40326,#40327),(#40328,#40329),(#40330,#40331),(#40332,
#40333),(#40334,#40335)),.UNSPECIFIED.,.F.,.F.,.F.,(6,1,1,1,1,1,1,1,1,1,
1,1,1,1,1,1,1,1,1,1,1,1,1,1,1,1,1,1,1,1,6),(2,2),(0.,0.0333333333333333,
0.0666666666666667,0.1,0.133333333333333,0.166666666666667,0.2,0.233333333333333,
0.266666666666667,0.3,0.333333333333333,0.366666666666667,0.4,0.433333333333333,
0.466666666666667,0.5,0.533333333333333,0.566666666666667,0.6,0.633333333333333,
0.666666666666667,0.7,0.733333333333333,0.766666666666667,0.8,0.833333333333333,
0.866666666666667,0.9,0.933333333333333,0.966666666666667,1.),(0.,0.762),
 .UNSPECIFIED.);
#882=B_SPLINE_SURFACE_WITH_KNOTS('',5,1,((#40377,#40378),(#40379,#40380),
(#40381,#40382),(#40383,#40384),(#40385,#40386),(#40387,#40388),(#40389,
#40390),(#40391,#40392),(#40393,#40394),(#40395,#40396),(#40397,#40398),
(#40399,#40400),(#40401,#40402),(#40403,#40404),(#40405,#40406),(#40407,
#40408),(#40409,#40410),(#40411,#40412),(#40413,#40414),(#40415,#40416),
(#40417,#40418),(#40419,#40420),(#40421,#40422),(#40423,#40424),(#40425,
#40426),(#40427,#40428),(#40429,#40430),(#40431,#40432),(#40433,#40434),
(#40435,#40436),(#40437,#40438),(#40439,#40440),(#40441,#40442),(#40443,
#40444),(#40445,#40446)),.UNSPECIFIED.,.F.,.F.,.F.,(6,1,1,1,1,1,1,1,1,1,
1,1,1,1,1,1,1,1,1,1,1,1,1,1,1,1,1,1,1,1,6),(2,2),(-1.,-0.966666666666667,
-0.933333333333333,-0.9,-0.866666666666667,-0.833333333333333,-0.8,-0.766666666666667,
-0.733333333333333,-0.7,-0.666666666666667,-0.633333333333333,-0.6,-0.566666666666667,
-0.533333333333333,-0.5,-0.466666666666667,-0.433333333333333,-0.4,-0.366666666666667,
-0.333333333333333,-0.3,-0.266666666666667,-0.233333333333333,-0.2,-0.166666666666667,
-0.133333333333333,-0.1,-0.0666666666666667,-0.0333333333333333,0.),(0.,
0.762),.UNSPECIFIED.);
#883=B_SPLINE_SURFACE_WITH_KNOTS('',5,1,((#40496,#40497),(#40498,#40499),
(#40500,#40501),(#40502,#40503),(#40504,#40505),(#40506,#40507),(#40508,
#40509),(#40510,#40511),(#40512,#40513),(#40514,#40515),(#40516,#40517),
(#40518,#40519),(#40520,#40521),(#40522,#40523),(#40524,#40525),(#40526,
#40527),(#40528,#40529),(#40530,#40531),(#40532,#40533),(#40534,#40535),
(#40536,#40537),(#40538,#40539),(#40540,#40541),(#40542,#40543),(#40544,
#40545),(#40546,#40547),(#40548,#40549),(#40550,#40551),(#40552,#40553),
(#40554,#40555),(#40556,#40557),(#40558,#40559),(#40560,#40561),(#40562,
#40563),(#40564,#40565)),.UNSPECIFIED.,.F.,.F.,.F.,(6,1,1,1,1,1,1,1,1,1,
1,1,1,1,1,1,1,1,1,1,1,1,1,1,1,1,1,1,1,1,6),(2,2),(0.,0.0333333333333333,
0.0666666666666667,0.1,0.133333333333333,0.166666666666667,0.2,0.233333333333333,
0.266666666666667,0.3,0.333333333333333,0.366666666666667,0.4,0.433333333333333,
0.466666666666667,0.5,0.533333333333333,0.566666666666667,0.6,0.633333333333333,
0.666666666666667,0.7,0.733333333333333,0.766666666666667,0.8,0.833333333333333,
0.866666666666667,0.9,0.933333333333333,0.966666666666667,1.),(0.,0.762),
 .UNSPECIFIED.);
#884=B_SPLINE_SURFACE_WITH_KNOTS('',5,1,((#40607,#40608),(#40609,#40610),
(#40611,#40612),(#40613,#40614),(#40615,#40616),(#40617,#40618),(#40619,
#40620),(#40621,#40622),(#40623,#40624),(#40625,#40626),(#40627,#40628),
(#40629,#40630),(#40631,#40632),(#40633,#40634),(#40635,#40636),(#40637,
#40638),(#40639,#40640),(#40641,#40642),(#40643,#40644),(#40645,#40646),
(#40647,#40648),(#40649,#40650),(#40651,#40652),(#40653,#40654),(#40655,
#40656),(#40657,#40658),(#40659,#40660),(#40661,#40662),(#40663,#40664),
(#40665,#40666),(#40667,#40668),(#40669,#40670),(#40671,#40672),(#40673,
#40674),(#40675,#40676)),.UNSPECIFIED.,.F.,.F.,.F.,(6,1,1,1,1,1,1,1,1,1,
1,1,1,1,1,1,1,1,1,1,1,1,1,1,1,1,1,1,1,1,6),(2,2),(-1.,-0.966666666666667,
-0.933333333333333,-0.9,-0.866666666666667,-0.833333333333333,-0.8,-0.766666666666667,
-0.733333333333333,-0.7,-0.666666666666667,-0.633333333333333,-0.6,-0.566666666666667,
-0.533333333333333,-0.5,-0.466666666666667,-0.433333333333333,-0.4,-0.366666666666667,
-0.333333333333333,-0.3,-0.266666666666667,-0.233333333333333,-0.2,-0.166666666666667,
-0.133333333333333,-0.1,-0.0666666666666667,-0.0333333333333333,0.),(0.,
0.762),.UNSPECIFIED.);
#885=B_SPLINE_SURFACE_WITH_KNOTS('',5,1,((#40726,#40727),(#40728,#40729),
(#40730,#40731),(#40732,#40733),(#40734,#40735),(#40736,#40737),(#40738,
#40739),(#40740,#40741),(#40742,#40743),(#40744,#40745),(#40746,#40747),
(#40748,#40749),(#40750,#40751),(#40752,#40753),(#40754,#40755),(#40756,
#40757),(#40758,#40759),(#40760,#40761),(#40762,#40763),(#40764,#40765),
(#40766,#40767),(#40768,#40769),(#40770,#40771),(#40772,#40773),(#40774,
#40775),(#40776,#40777),(#40778,#40779),(#40780,#40781),(#40782,#40783),
(#40784,#40785),(#40786,#40787),(#40788,#40789),(#40790,#40791),(#40792,
#40793),(#40794,#40795)),.UNSPECIFIED.,.F.,.F.,.F.,(6,1,1,1,1,1,1,1,1,1,
1,1,1,1,1,1,1,1,1,1,1,1,1,1,1,1,1,1,1,1,6),(2,2),(0.,0.0333333333333333,
0.0666666666666667,0.1,0.133333333333333,0.166666666666667,0.2,0.233333333333333,
0.266666666666667,0.3,0.333333333333333,0.366666666666667,0.4,0.433333333333333,
0.466666666666667,0.5,0.533333333333333,0.566666666666667,0.6,0.633333333333333,
0.666666666666667,0.7,0.733333333333333,0.766666666666667,0.8,0.833333333333333,
0.866666666666667,0.9,0.933333333333333,0.966666666666667,1.),(0.,0.762),
 .UNSPECIFIED.);
#886=B_SPLINE_SURFACE_WITH_KNOTS('',5,1,((#40837,#40838),(#40839,#40840),
(#40841,#40842),(#40843,#40844),(#40845,#40846),(#40847,#40848),(#40849,
#40850),(#40851,#40852),(#40853,#40854),(#40855,#40856),(#40857,#40858),
(#40859,#40860),(#40861,#40862),(#40863,#40864),(#40865,#40866),(#40867,
#40868),(#40869,#40870),(#40871,#40872),(#40873,#40874),(#40875,#40876),
(#40877,#40878),(#40879,#40880),(#40881,#40882),(#40883,#40884),(#40885,
#40886),(#40887,#40888),(#40889,#40890),(#40891,#40892),(#40893,#40894),
(#40895,#40896),(#40897,#40898),(#40899,#40900),(#40901,#40902),(#40903,
#40904),(#40905,#40906)),.UNSPECIFIED.,.F.,.F.,.F.,(6,1,1,1,1,1,1,1,1,1,
1,1,1,1,1,1,1,1,1,1,1,1,1,1,1,1,1,1,1,1,6),(2,2),(-1.,-0.966666666666667,
-0.933333333333333,-0.9,-0.866666666666667,-0.833333333333333,-0.8,-0.766666666666667,
-0.733333333333333,-0.7,-0.666666666666667,-0.633333333333333,-0.6,-0.566666666666667,
-0.533333333333333,-0.5,-0.466666666666667,-0.433333333333333,-0.4,-0.366666666666667,
-0.333333333333333,-0.3,-0.266666666666667,-0.233333333333333,-0.2,-0.166666666666667,
-0.133333333333333,-0.1,-0.0666666666666667,-0.0333333333333333,0.),(0.,
0.762),.UNSPECIFIED.);
#887=B_SPLINE_SURFACE_WITH_KNOTS('',5,1,((#40956,#40957),(#40958,#40959),
(#40960,#40961),(#40962,#40963),(#40964,#40965),(#40966,#40967),(#40968,
#40969),(#40970,#40971),(#40972,#40973),(#40974,#40975),(#40976,#40977),
(#40978,#40979),(#40980,#40981),(#40982,#40983),(#40984,#40985),(#40986,
#40987),(#40988,#40989),(#40990,#40991),(#40992,#40993),(#40994,#40995),
(#40996,#40997),(#40998,#40999),(#41000,#41001),(#41002,#41003),(#41004,
#41005),(#41006,#41007),(#41008,#41009),(#41010,#41011),(#41012,#41013),
(#41014,#41015),(#41016,#41017),(#41018,#41019),(#41020,#41021),(#41022,
#41023),(#41024,#41025)),.UNSPECIFIED.,.F.,.F.,.F.,(6,1,1,1,1,1,1,1,1,1,
1,1,1,1,1,1,1,1,1,1,1,1,1,1,1,1,1,1,1,1,6),(2,2),(0.,0.0333333333333333,
0.0666666666666667,0.1,0.133333333333333,0.166666666666667,0.2,0.233333333333333,
0.266666666666667,0.3,0.333333333333333,0.366666666666667,0.4,0.433333333333333,
0.466666666666667,0.5,0.533333333333333,0.566666666666667,0.6,0.633333333333333,
0.666666666666667,0.7,0.733333333333333,0.766666666666667,0.8,0.833333333333333,
0.866666666666667,0.9,0.933333333333333,0.966666666666667,1.),(0.,0.762),
 .UNSPECIFIED.);
#888=B_SPLINE_SURFACE_WITH_KNOTS('',5,1,((#41067,#41068),(#41069,#41070),
(#41071,#41072),(#41073,#41074),(#41075,#41076),(#41077,#41078),(#41079,
#41080),(#41081,#41082),(#41083,#41084),(#41085,#41086),(#41087,#41088),
(#41089,#41090),(#41091,#41092),(#41093,#41094),(#41095,#41096),(#41097,
#41098),(#41099,#41100),(#41101,#41102),(#41103,#41104),(#41105,#41106),
(#41107,#41108),(#41109,#41110),(#41111,#41112),(#41113,#41114),(#41115,
#41116),(#41117,#41118),(#41119,#41120),(#41121,#41122),(#41123,#41124),
(#41125,#41126),(#41127,#41128),(#41129,#41130),(#41131,#41132),(#41133,
#41134),(#41135,#41136)),.UNSPECIFIED.,.F.,.F.,.F.,(6,1,1,1,1,1,1,1,1,1,
1,1,1,1,1,1,1,1,1,1,1,1,1,1,1,1,1,1,1,1,6),(2,2),(-1.,-0.966666666666667,
-0.933333333333333,-0.9,-0.866666666666667,-0.833333333333333,-0.8,-0.766666666666667,
-0.733333333333333,-0.7,-0.666666666666667,-0.633333333333333,-0.6,-0.566666666666667,
-0.533333333333333,-0.5,-0.466666666666667,-0.433333333333333,-0.4,-0.366666666666667,
-0.333333333333333,-0.3,-0.266666666666667,-0.233333333333333,-0.2,-0.166666666666667,
-0.133333333333333,-0.1,-0.0666666666666667,-0.0333333333333333,0.),(0.,
0.762),.UNSPECIFIED.);
#889=B_SPLINE_SURFACE_WITH_KNOTS('',5,1,((#41186,#41187),(#41188,#41189),
(#41190,#41191),(#41192,#41193),(#41194,#41195),(#41196,#41197),(#41198,
#41199),(#41200,#41201),(#41202,#41203),(#41204,#41205),(#41206,#41207),
(#41208,#41209),(#41210,#41211),(#41212,#41213),(#41214,#41215),(#41216,
#41217),(#41218,#41219),(#41220,#41221),(#41222,#41223),(#41224,#41225),
(#41226,#41227),(#41228,#41229),(#41230,#41231),(#41232,#41233),(#41234,
#41235),(#41236,#41237),(#41238,#41239),(#41240,#41241),(#41242,#41243),
(#41244,#41245),(#41246,#41247),(#41248,#41249),(#41250,#41251),(#41252,
#41253),(#41254,#41255)),.UNSPECIFIED.,.F.,.F.,.F.,(6,1,1,1,1,1,1,1,1,1,
1,1,1,1,1,1,1,1,1,1,1,1,1,1,1,1,1,1,1,1,6),(2,2),(0.,0.0333333333333333,
0.0666666666666667,0.1,0.133333333333333,0.166666666666667,0.2,0.233333333333333,
0.266666666666667,0.3,0.333333333333333,0.366666666666667,0.4,0.433333333333333,
0.466666666666667,0.5,0.533333333333333,0.566666666666667,0.6,0.633333333333333,
0.666666666666667,0.7,0.733333333333333,0.766666666666667,0.8,0.833333333333333,
0.866666666666667,0.9,0.933333333333333,0.966666666666667,1.),(0.,0.762),
 .UNSPECIFIED.);
#890=B_SPLINE_SURFACE_WITH_KNOTS('',5,1,((#41297,#41298),(#41299,#41300),
(#41301,#41302),(#41303,#41304),(#41305,#41306),(#41307,#41308),(#41309,
#41310),(#41311,#41312),(#41313,#41314),(#41315,#41316),(#41317,#41318),
(#41319,#41320),(#41321,#41322),(#41323,#41324),(#41325,#41326),(#41327,
#41328),(#41329,#41330),(#41331,#41332),(#41333,#41334),(#41335,#41336),
(#41337,#41338),(#41339,#41340),(#41341,#41342),(#41343,#41344),(#41345,
#41346),(#41347,#41348),(#41349,#41350),(#41351,#41352),(#41353,#41354),
(#41355,#41356),(#41357,#41358),(#41359,#41360),(#41361,#41362),(#41363,
#41364),(#41365,#41366)),.UNSPECIFIED.,.F.,.F.,.F.,(6,1,1,1,1,1,1,1,1,1,
1,1,1,1,1,1,1,1,1,1,1,1,1,1,1,1,1,1,1,1,6),(2,2),(-1.,-0.966666666666667,
-0.933333333333333,-0.9,-0.866666666666667,-0.833333333333333,-0.8,-0.766666666666667,
-0.733333333333333,-0.7,-0.666666666666667,-0.633333333333333,-0.6,-0.566666666666667,
-0.533333333333333,-0.5,-0.466666666666667,-0.433333333333333,-0.4,-0.366666666666667,
-0.333333333333333,-0.3,-0.266666666666667,-0.233333333333333,-0.2,-0.166666666666667,
-0.133333333333333,-0.1,-0.0666666666666667,-0.0333333333333333,0.),(0.,
0.762),.UNSPECIFIED.);
#891=B_SPLINE_SURFACE_WITH_KNOTS('',5,1,((#41416,#41417),(#41418,#41419),
(#41420,#41421),(#41422,#41423),(#41424,#41425),(#41426,#41427),(#41428,
#41429),(#41430,#41431),(#41432,#41433),(#41434,#41435),(#41436,#41437),
(#41438,#41439),(#41440,#41441),(#41442,#41443),(#41444,#41445),(#41446,
#41447),(#41448,#41449),(#41450,#41451),(#41452,#41453),(#41454,#41455),
(#41456,#41457),(#41458,#41459),(#41460,#41461),(#41462,#41463),(#41464,
#41465),(#41466,#41467),(#41468,#41469),(#41470,#41471),(#41472,#41473),
(#41474,#41475),(#41476,#41477),(#41478,#41479),(#41480,#41481),(#41482,
#41483),(#41484,#41485)),.UNSPECIFIED.,.F.,.F.,.F.,(6,1,1,1,1,1,1,1,1,1,
1,1,1,1,1,1,1,1,1,1,1,1,1,1,1,1,1,1,1,1,6),(2,2),(0.,0.0333333333333333,
0.0666666666666667,0.1,0.133333333333333,0.166666666666667,0.2,0.233333333333333,
0.266666666666667,0.3,0.333333333333333,0.366666666666667,0.4,0.433333333333333,
0.466666666666667,0.5,0.533333333333333,0.566666666666667,0.6,0.633333333333333,
0.666666666666667,0.7,0.733333333333333,0.766666666666667,0.8,0.833333333333333,
0.866666666666667,0.9,0.933333333333333,0.966666666666667,1.),(0.,0.762),
 .UNSPECIFIED.);
#892=B_SPLINE_SURFACE_WITH_KNOTS('',5,1,((#41527,#41528),(#41529,#41530),
(#41531,#41532),(#41533,#41534),(#41535,#41536),(#41537,#41538),(#41539,
#41540),(#41541,#41542),(#41543,#41544),(#41545,#41546),(#41547,#41548),
(#41549,#41550),(#41551,#41552),(#41553,#41554),(#41555,#41556),(#41557,
#41558),(#41559,#41560),(#41561,#41562),(#41563,#41564),(#41565,#41566),
(#41567,#41568),(#41569,#41570),(#41571,#41572),(#41573,#41574),(#41575,
#41576),(#41577,#41578),(#41579,#41580),(#41581,#41582),(#41583,#41584),
(#41585,#41586),(#41587,#41588),(#41589,#41590),(#41591,#41592),(#41593,
#41594),(#41595,#41596)),.UNSPECIFIED.,.F.,.F.,.F.,(6,1,1,1,1,1,1,1,1,1,
1,1,1,1,1,1,1,1,1,1,1,1,1,1,1,1,1,1,1,1,6),(2,2),(-1.,-0.966666666666667,
-0.933333333333333,-0.9,-0.866666666666667,-0.833333333333333,-0.8,-0.766666666666667,
-0.733333333333333,-0.7,-0.666666666666667,-0.633333333333333,-0.6,-0.566666666666667,
-0.533333333333333,-0.5,-0.466666666666667,-0.433333333333333,-0.4,-0.366666666666667,
-0.333333333333333,-0.3,-0.266666666666667,-0.233333333333333,-0.2,-0.166666666666667,
-0.133333333333333,-0.1,-0.0666666666666667,-0.0333333333333333,0.),(0.,
0.762),.UNSPECIFIED.);
#893=B_SPLINE_SURFACE_WITH_KNOTS('',5,1,((#41652,#41653),(#41654,#41655),
(#41656,#41657),(#41658,#41659),(#41660,#41661),(#41662,#41663),(#41664,
#41665),(#41666,#41667),(#41668,#41669),(#41670,#41671),(#41672,#41673),
(#41674,#41675),(#41676,#41677),(#41678,#41679),(#41680,#41681),(#41682,
#41683),(#41684,#41685),(#41686,#41687),(#41688,#41689),(#41690,#41691),
(#41692,#41693),(#41694,#41695),(#41696,#41697),(#41698,#41699),(#41700,
#41701),(#41702,#41703),(#41704,#41705),(#41706,#41707),(#41708,#41709),
(#41710,#41711),(#41712,#41713),(#41714,#41715),(#41716,#41717),(#41718,
#41719),(#41720,#41721)),.UNSPECIFIED.,.F.,.F.,.F.,(6,1,1,1,1,1,1,1,1,1,
1,1,1,1,1,1,1,1,1,1,1,1,1,1,1,1,1,1,1,1,6),(2,2),(0.,0.0333333333333333,
0.0666666666666667,0.1,0.133333333333333,0.166666666666667,0.2,0.233333333333333,
0.266666666666667,0.3,0.333333333333333,0.366666666666667,0.4,0.433333333333333,
0.466666666666667,0.5,0.533333333333333,0.566666666666667,0.6,0.633333333333333,
0.666666666666667,0.7,0.733333333333333,0.766666666666667,0.8,0.833333333333333,
0.866666666666667,0.9,0.933333333333333,0.966666666666667,1.),(0.,0.762),
 .UNSPECIFIED.);
#894=B_SPLINE_SURFACE_WITH_KNOTS('',5,1,((#41757,#41758),(#41759,#41760),
(#41761,#41762),(#41763,#41764),(#41765,#41766),(#41767,#41768),(#41769,
#41770),(#41771,#41772),(#41773,#41774),(#41775,#41776),(#41777,#41778),
(#41779,#41780),(#41781,#41782),(#41783,#41784),(#41785,#41786),(#41787,
#41788),(#41789,#41790),(#41791,#41792),(#41793,#41794),(#41795,#41796),
(#41797,#41798),(#41799,#41800),(#41801,#41802),(#41803,#41804),(#41805,
#41806),(#41807,#41808),(#41809,#41810),(#41811,#41812),(#41813,#41814),
(#41815,#41816),(#41817,#41818),(#41819,#41820),(#41821,#41822),(#41823,
#41824),(#41825,#41826)),.UNSPECIFIED.,.F.,.F.,.F.,(6,1,1,1,1,1,1,1,1,1,
1,1,1,1,1,1,1,1,1,1,1,1,1,1,1,1,1,1,1,1,6),(2,2),(-1.,-0.966666666666667,
-0.933333333333333,-0.9,-0.866666666666667,-0.833333333333333,-0.8,-0.766666666666667,
-0.733333333333333,-0.7,-0.666666666666667,-0.633333333333333,-0.6,-0.566666666666667,
-0.533333333333333,-0.5,-0.466666666666667,-0.433333333333333,-0.4,-0.366666666666667,
-0.333333333333333,-0.3,-0.266666666666667,-0.233333333333333,-0.2,-0.166666666666667,
-0.133333333333333,-0.1,-0.0666666666666667,-0.0333333333333333,0.),(0.,
0.762),.UNSPECIFIED.);
#895=B_SPLINE_SURFACE_WITH_KNOTS('',5,1,((#41953,#41954),(#41955,#41956),
(#41957,#41958),(#41959,#41960),(#41961,#41962),(#41963,#41964),(#41965,
#41966),(#41967,#41968),(#41969,#41970),(#41971,#41972),(#41973,#41974),
(#41975,#41976),(#41977,#41978),(#41979,#41980),(#41981,#41982),(#41983,
#41984),(#41985,#41986),(#41987,#41988),(#41989,#41990),(#41991,#41992),
(#41993,#41994),(#41995,#41996),(#41997,#41998),(#41999,#42000),(#42001,
#42002),(#42003,#42004),(#42005,#42006),(#42007,#42008),(#42009,#42010),
(#42011,#42012),(#42013,#42014),(#42015,#42016),(#42017,#42018),(#42019,
#42020),(#42021,#42022)),.UNSPECIFIED.,.F.,.F.,.F.,(6,1,1,1,1,1,1,1,1,1,
1,1,1,1,1,1,1,1,1,1,1,1,1,1,1,1,1,1,1,1,6),(2,2),(0.,0.0333333333333333,
0.0666666666666667,0.1,0.133333333333333,0.166666666666667,0.2,0.233333333333333,
0.266666666666667,0.3,0.333333333333333,0.366666666666667,0.4,0.433333333333333,
0.466666666666667,0.5,0.533333333333333,0.566666666666667,0.6,0.633333333333333,
0.666666666666667,0.7,0.733333333333333,0.766666666666667,0.8,0.833333333333333,
0.866666666666667,0.9,0.933333333333333,0.966666666666667,1.),(0.,0.762),
 .UNSPECIFIED.);
#896=B_SPLINE_SURFACE_WITH_KNOTS('',5,1,((#42026,#42027),(#42028,#42029),
(#42030,#42031),(#42032,#42033),(#42034,#42035),(#42036,#42037),(#42038,
#42039),(#42040,#42041),(#42042,#42043),(#42044,#42045),(#42046,#42047),
(#42048,#42049),(#42050,#42051),(#42052,#42053),(#42054,#42055),(#42056,
#42057),(#42058,#42059),(#42060,#42061),(#42062,#42063),(#42064,#42065),
(#42066,#42067),(#42068,#42069),(#42070,#42071),(#42072,#42073),(#42074,
#42075),(#42076,#42077),(#42078,#42079),(#42080,#42081),(#42082,#42083),
(#42084,#42085),(#42086,#42087),(#42088,#42089),(#42090,#42091),(#42092,
#42093),(#42094,#42095)),.UNSPECIFIED.,.F.,.F.,.F.,(6,1,1,1,1,1,1,1,1,1,
1,1,1,1,1,1,1,1,1,1,1,1,1,1,1,1,1,1,1,1,6),(2,2),(-1.,-0.966666666666667,
-0.933333333333333,-0.9,-0.866666666666667,-0.833333333333333,-0.8,-0.766666666666667,
-0.733333333333333,-0.7,-0.666666666666667,-0.633333333333333,-0.6,-0.566666666666667,
-0.533333333333333,-0.5,-0.466666666666667,-0.433333333333333,-0.4,-0.366666666666667,
-0.333333333333333,-0.3,-0.266666666666667,-0.233333333333333,-0.2,-0.166666666666667,
-0.133333333333333,-0.1,-0.0666666666666667,-0.0333333333333333,0.),(0.,
0.762),.UNSPECIFIED.);
#908=SHAPE_REPRESENTATION_RELATIONSHIP('SRR','None',#83303,#922);
#922=ADVANCED_BREP_SHAPE_REPRESENTATION('',(#950),#83208);
#936=STYLED_ITEM('',(#83382),#950);
#950=MANIFOLD_SOLID_BREP('Body1',#26932);
#1013=FACE_BOUND('',#4005,.T.);
#1014=FACE_BOUND('',#4091,.T.);
#1015=FACE_BOUND('',#4100,.T.);
#1016=FACE_BOUND('',#4103,.T.);
#1248=PLANE('',#27454);
#1249=PLANE('',#27458);
#1250=PLANE('',#27459);
#1251=PLANE('',#27494);
#1252=PLANE('',#27497);
#1253=PLANE('',#27500);
#1254=PLANE('',#27503);
#1255=PLANE('',#27506);
#1256=PLANE('',#27509);
#1257=PLANE('',#27512);
#1258=PLANE('',#27515);
#1259=PLANE('',#27518);
#1260=PLANE('',#27521);
#1261=PLANE('',#27524);
#1262=PLANE('',#27527);
#1263=PLANE('',#27530);
#1264=PLANE('',#27533);
#1265=PLANE('',#27536);
#1266=PLANE('',#27539);
#1267=PLANE('',#27542);
#1268=PLANE('',#27545);
#1269=PLANE('',#27548);
#1270=PLANE('',#27551);
#1271=PLANE('',#27554);
#1272=PLANE('',#27557);
#1273=PLANE('',#27560);
#1274=PLANE('',#27563);
#1275=PLANE('',#27566);
#1276=PLANE('',#27569);
#1277=PLANE('',#27572);
#1278=PLANE('',#27573);
#1279=PLANE('',#27576);
#1280=PLANE('',#27582);
#1281=PLANE('',#27584);
#1282=PLANE('',#27586);
#1283=PLANE('',#27591);
#2193=CYLINDRICAL_SURFACE('',#27455,7.14399999999837);
#2194=CYLINDRICAL_SURFACE('',#27492,5.358);
#2195=CYLINDRICAL_SURFACE('',#27495,7.14399999999837);
#2196=CYLINDRICAL_SURFACE('',#27498,5.358);
#2197=CYLINDRICAL_SURFACE('',#27501,7.14399999999837);
#2198=CYLINDRICAL_SURFACE('',#27504,5.358);
#2199=CYLINDRICAL_SURFACE('',#27507,7.14399999999837);
#2200=CYLINDRICAL_SURFACE('',#27510,5.358);
#2201=CYLINDRICAL_SURFACE('',#27513,7.14399999999837);
#2202=CYLINDRICAL_SURFACE('',#27516,5.358);
#2203=CYLINDRICAL_SURFACE('',#27519,7.14399999999837);
#2204=CYLINDRICAL_SURFACE('',#27522,5.358);
#2205=CYLINDRICAL_SURFACE('',#27525,7.14399999999837);
#2206=CYLINDRICAL_SURFACE('',#27528,5.358);
#2207=CYLINDRICAL_SURFACE('',#27531,7.14399999999837);
#2208=CYLINDRICAL_SURFACE('',#27534,5.358);
#2209=CYLINDRICAL_SURFACE('',#27537,7.14399999999837);
#2210=CYLINDRICAL_SURFACE('',#27540,5.358);
#2211=CYLINDRICAL_SURFACE('',#27543,7.14399999999837);
#2212=CYLINDRICAL_SURFACE('',#27546,5.358);
#2213=CYLINDRICAL_SURFACE('',#27549,7.14399999999837);
#2214=CYLINDRICAL_SURFACE('',#27552,5.358);
#2215=CYLINDRICAL_SURFACE('',#27555,7.14399999999837);
#2216=CYLINDRICAL_SURFACE('',#27558,5.358);
#2217=CYLINDRICAL_SURFACE('',#27561,7.14399999999837);
#2218=CYLINDRICAL_SURFACE('',#27564,5.358);
#2219=CYLINDRICAL_SURFACE('',#27567,7.14399999999837);
#2220=CYLINDRICAL_SURFACE('',#27570,5.358);
#2221=CYLINDRICAL_SURFACE('',#27574,7.14399999999837);
#2222=CYLINDRICAL_SURFACE('',#27581,5.358);
#2223=CYLINDRICAL_SURFACE('',#27583,7.14399999999837);
#2224=CYLINDRICAL_SURFACE('',#27585,5.358);
#2225=CYLINDRICAL_SURFACE('',#27589,1.6);
#2226=CYLINDRICAL_SURFACE('',#27593,4.477);
#2227=CYLINDRICAL_SURFACE('',#27594,3.261);
#2568=FACE_OUTER_BOUND('',#3999,.T.);
#2569=FACE_OUTER_BOUND('',#4000,.T.);
#2570=FACE_OUTER_BOUND('',#4001,.T.);
#2571=FACE_OUTER_BOUND('',#4002,.T.);
#2572=FACE_OUTER_BOUND('',#4003,.T.);
#2573=FACE_OUTER_BOUND('',#4004,.T.);
#2574=FACE_OUTER_BOUND('',#4006,.T.);
#2575=FACE_OUTER_BOUND('',#4007,.T.);
#2576=FACE_OUTER_BOUND('',#4008,.T.);
#2577=FACE_OUTER_BOUND('',#4009,.T.);
#2578=FACE_OUTER_BOUND('',#4010,.T.);
#2579=FACE_OUTER_BOUND('',#4011,.T.);
#2580=FACE_OUTER_BOUND('',#4012,.T.);
#2581=FACE_OUTER_BOUND('',#4013,.T.);
#2582=FACE_OUTER_BOUND('',#4014,.T.);
#2583=FACE_OUTER_BOUND('',#4015,.T.);
#2584=FACE_OUTER_BOUND('',#4016,.T.);
#2585=FACE_OUTER_BOUND('',#4017,.T.);
#2586=FACE_OUTER_BOUND('',#4018,.T.);
#2587=FACE_OUTER_BOUND('',#4019,.T.);
#2588=FACE_OUTER_BOUND('',#4020,.T.);
#2589=FACE_OUTER_BOUND('',#4021,.T.);
#2590=FACE_OUTER_BOUND('',#4022,.T.);
#2591=FACE_OUTER_BOUND('',#4023,.T.);
#2592=FACE_OUTER_BOUND('',#4024,.T.);
#2593=FACE_OUTER_BOUND('',#4025,.T.);
#2594=FACE_OUTER_BOUND('',#4026,.T.);
#2595=FACE_OUTER_BOUND('',#4027,.T.);
#2596=FACE_OUTER_BOUND('',#4028,.T.);
#2597=FACE_OUTER_BOUND('',#4029,.T.);
#2598=FACE_OUTER_BOUND('',#4030,.T.);
#2599=FACE_OUTER_BOUND('',#4031,.T.);
#2600=FACE_OUTER_BOUND('',#4032,.T.);
#2601=FACE_OUTER_BOUND('',#4033,.T.);
#2602=FACE_OUTER_BOUND('',#4034,.T.);
#2603=FACE_OUTER_BOUND('',#4035,.T.);
#2604=FACE_OUTER_BOUND('',#4036,.T.);
#2605=FACE_OUTER_BOUND('',#4037,.T.);
#2606=FACE_OUTER_BOUND('',#4038,.T.);
#2607=FACE_OUTER_BOUND('',#4039,.T.);
#2608=FACE_OUTER_BOUND('',#4040,.T.);
#2609=FACE_OUTER_BOUND('',#4041,.T.);
#2610=FACE_OUTER_BOUND('',#4042,.T.);
#2611=FACE_OUTER_BOUND('',#4043,.T.);
#2612=FACE_OUTER_BOUND('',#4044,.T.);
#2613=FACE_OUTER_BOUND('',#4045,.T.);
#2614=FACE_OUTER_BOUND('',#4046,.T.);
#2615=FACE_OUTER_BOUND('',#4047,.T.);
#2616=FACE_OUTER_BOUND('',#4048,.T.);
#2617=FACE_OUTER_BOUND('',#4049,.T.);
#2618=FACE_OUTER_BOUND('',#4050,.T.);
#2619=FACE_OUTER_BOUND('',#4051,.T.);
#2620=FACE_OUTER_BOUND('',#4052,.T.);
#2621=FACE_OUTER_BOUND('',#4053,.T.);
#2622=FACE_OUTER_BOUND('',#4054,.T.);
#2623=FACE_OUTER_BOUND('',#4055,.T.);
#2624=FACE_OUTER_BOUND('',#4056,.T.);
#2625=FACE_OUTER_BOUND('',#4057,.T.);
#2626=FACE_OUTER_BOUND('',#4058,.T.);
#2627=FACE_OUTER_BOUND('',#4059,.T.);
#2628=FACE_OUTER_BOUND('',#4060,.T.);
#2629=FACE_OUTER_BOUND('',#4061,.T.);
#2630=FACE_OUTER_BOUND('',#4062,.T.);
#2631=FACE_OUTER_BOUND('',#4063,.T.);
#2632=FACE_OUTER_BOUND('',#4064,.T.);
#2633=FACE_OUTER_BOUND('',#4065,.T.);
#2634=FACE_OUTER_BOUND('',#4066,.T.);
#2635=FACE_OUTER_BOUND('',#4067,.T.);
#2636=FACE_OUTER_BOUND('',#4068,.T.);
#2637=FACE_OUTER_BOUND('',#4069,.T.);
#2638=FACE_OUTER_BOUND('',#4070,.T.);
#2639=FACE_OUTER_BOUND('',#4071,.T.);
#2640=FACE_OUTER_BOUND('',#4072,.T.);
#2641=FACE_OUTER_BOUND('',#4073,.T.);
#2642=FACE_OUTER_BOUND('',#4074,.T.);
#2643=FACE_OUTER_BOUND('',#4075,.T.);
#2644=FACE_OUTER_BOUND('',#4076,.T.);
#2645=FACE_OUTER_BOUND('',#4077,.T.);
#2646=FACE_OUTER_BOUND('',#4078,.T.);
#2647=FACE_OUTER_BOUND('',#4079,.T.);
#2648=FACE_OUTER_BOUND('',#4080,.T.);
#2649=FACE_OUTER_BOUND('',#4081,.T.);
#2650=FACE_OUTER_BOUND('',#4082,.T.);
#2651=FACE_OUTER_BOUND('',#4083,.T.);
#2652=FACE_OUTER_BOUND('',#4084,.T.);
#2653=FACE_OUTER_BOUND('',#4085,.T.);
#2654=FACE_OUTER_BOUND('',#4086,.T.);
#2655=FACE_OUTER_BOUND('',#4087,.T.);
#2656=FACE_OUTER_BOUND('',#4088,.T.);
#2657=FACE_OUTER_BOUND('',#4089,.T.);
#2658=FACE_OUTER_BOUND('',#4090,.T.);
#2659=FACE_OUTER_BOUND('',#4092,.T.);
#2660=FACE_OUTER_BOUND('',#4093,.T.);
#2661=FACE_OUTER_BOUND('',#4094,.T.);
#2662=FACE_OUTER_BOUND('',#4095,.T.);
#2663=FACE_OUTER_BOUND('',#4096,.T.);
#2664=FACE_OUTER_BOUND('',#4097,.T.);
#2665=FACE_OUTER_BOUND('',#4098,.T.);
#2666=FACE_OUTER_BOUND('',#4099,.T.);
#2667=FACE_OUTER_BOUND('',#4101,.T.);
#2668=FACE_OUTER_BOUND('',#4102,.T.);
#2669=FACE_OUTER_BOUND('',#4104,.T.);
#2670=FACE_OUTER_BOUND('',#4105,.T.);
#3999=EDGE_LOOP('',(#18618,#18619,#18620,#18621));
#4000=EDGE_LOOP('',(#18622,#18623,#18624,#18625));
#4001=EDGE_LOOP('',(#18626,#18627,#18628,#18629));
#4002=EDGE_LOOP('',(#18630,#18631,#18632,#18633));
#4003=EDGE_LOOP('',(#18634,#18635,#18636,#18637));
#4004=EDGE_LOOP('',(#18638,#18639,#18640,#18641,#18642,#18643,#18644,#18645,
#18646,#18647,#18648,#18649,#18650,#18651,#18652,#18653,#18654,#18655,#18656,
#18657,#18658,#18659,#18660,#18661,#18662,#18663,#18664,#18665,#18666,#18667,
#18668,#18669,#18670,#18671,#18672,#18673,#18674,#18675,#18676,#18677,#18678,
#18679,#18680,#18681,#18682,#18683,#18684,#18685,#18686,#18687,#18688,#18689,
#18690,#18691,#18692,#18693,#18694,#18695,#18696,#18697,#18698,#18699,#18700,
#18701,#18702,#18703,#18704,#18705,#18706,#18707,#18708,#18709,#18710,#18711,
#18712,#18713,#18714,#18715,#18716,#18717,#18718,#18719,#18720,#18721,#18722,
#18723,#18724,#18725,#18726,#18727,#18728,#18729,#18730,#18731,#18732,#18733));
#4005=EDGE_LOOP('',(#18734));
#4006=EDGE_LOOP('',(#18735,#18736,#18737,#18738));
#4007=EDGE_LOOP('',(#18739,#18740,#18741,#18742));
#4008=EDGE_LOOP('',(#18743,#18744,#18745,#18746));
#4009=EDGE_LOOP('',(#18747,#18748,#18749,#18750));
#4010=EDGE_LOOP('',(#18751,#18752,#18753,#18754));
#4011=EDGE_LOOP('',(#18755,#18756,#18757,#18758));
#4012=EDGE_LOOP('',(#18759,#18760,#18761,#18762));
#4013=EDGE_LOOP('',(#18763,#18764,#18765,#18766));
#4014=EDGE_LOOP('',(#18767,#18768,#18769,#18770));
#4015=EDGE_LOOP('',(#18771,#18772,#18773,#18774));
#4016=EDGE_LOOP('',(#18775,#18776,#18777,#18778));
#4017=EDGE_LOOP('',(#18779,#18780,#18781,#18782));
#4018=EDGE_LOOP('',(#18783,#18784,#18785,#18786));
#4019=EDGE_LOOP('',(#18787,#18788,#18789,#18790));
#4020=EDGE_LOOP('',(#18791,#18792,#18793,#18794));
#4021=EDGE_LOOP('',(#18795,#18796,#18797,#18798));
#4022=EDGE_LOOP('',(#18799,#18800,#18801,#18802));
#4023=EDGE_LOOP('',(#18803,#18804,#18805,#18806));
#4024=EDGE_LOOP('',(#18807,#18808,#18809,#18810));
#4025=EDGE_LOOP('',(#18811,#18812,#18813,#18814));
#4026=EDGE_LOOP('',(#18815,#18816,#18817,#18818));
#4027=EDGE_LOOP('',(#18819,#18820,#18821,#18822));
#4028=EDGE_LOOP('',(#18823,#18824,#18825,#18826));
#4029=EDGE_LOOP('',(#18827,#18828,#18829,#18830));
#4030=EDGE_LOOP('',(#18831,#18832,#18833,#18834));
#4031=EDGE_LOOP('',(#18835,#18836,#18837,#18838));
#4032=EDGE_LOOP('',(#18839,#18840,#18841,#18842));
#4033=EDGE_LOOP('',(#18843,#18844,#18845,#18846));
#4034=EDGE_LOOP('',(#18847,#18848,#18849,#18850));
#4035=EDGE_LOOP('',(#18851,#18852,#18853,#18854));
#4036=EDGE_LOOP('',(#18855,#18856,#18857,#18858));
#4037=EDGE_LOOP('',(#18859,#18860,#18861,#18862));
#4038=EDGE_LOOP('',(#18863,#18864,#18865,#18866));
#4039=EDGE_LOOP('',(#18867,#18868,#18869,#18870));
#4040=EDGE_LOOP('',(#18871,#18872,#18873,#18874));
#4041=EDGE_LOOP('',(#18875,#18876,#18877,#18878));
#4042=EDGE_LOOP('',(#18879,#18880,#18881,#18882));
#4043=EDGE_LOOP('',(#18883,#18884,#18885,#18886));
#4044=EDGE_LOOP('',(#18887,#18888,#18889,#18890));
#4045=EDGE_LOOP('',(#18891,#18892,#18893,#18894));
#4046=EDGE_LOOP('',(#18895,#18896,#18897,#18898));
#4047=EDGE_LOOP('',(#18899,#18900,#18901,#18902));
#4048=EDGE_LOOP('',(#18903,#18904,#18905,#18906));
#4049=EDGE_LOOP('',(#18907,#18908,#18909,#18910));
#4050=EDGE_LOOP('',(#18911,#18912,#18913,#18914));
#4051=EDGE_LOOP('',(#18915,#18916,#18917,#18918));
#4052=EDGE_LOOP('',(#18919,#18920,#18921,#18922));
#4053=EDGE_LOOP('',(#18923,#18924,#18925,#18926));
#4054=EDGE_LOOP('',(#18927,#18928,#18929,#18930));
#4055=EDGE_LOOP('',(#18931,#18932,#18933,#18934));
#4056=EDGE_LOOP('',(#18935,#18936,#18937,#18938));
#4057=EDGE_LOOP('',(#18939,#18940,#18941,#18942));
#4058=EDGE_LOOP('',(#18943,#18944,#18945,#18946));
#4059=EDGE_LOOP('',(#18947,#18948,#18949,#18950));
#4060=EDGE_LOOP('',(#18951,#18952,#18953,#18954));
#4061=EDGE_LOOP('',(#18955,#18956,#18957,#18958));
#4062=EDGE_LOOP('',(#18959,#18960,#18961,#18962));
#4063=EDGE_LOOP('',(#18963,#18964,#18965,#18966));
#4064=EDGE_LOOP('',(#18967,#18968,#18969,#18970));
#4065=EDGE_LOOP('',(#18971,#18972,#18973,#18974));
#4066=EDGE_LOOP('',(#18975,#18976,#18977,#18978));
#4067=EDGE_LOOP('',(#18979,#18980,#18981,#18982));
#4068=EDGE_LOOP('',(#18983,#18984,#18985,#18986));
#4069=EDGE_LOOP('',(#18987,#18988,#18989,#18990));
#4070=EDGE_LOOP('',(#18991,#18992,#18993,#18994));
#4071=EDGE_LOOP('',(#18995,#18996,#18997,#18998));
#4072=EDGE_LOOP('',(#18999,#19000,#19001,#19002));
#4073=EDGE_LOOP('',(#19003,#19004,#19005,#19006));
#4074=EDGE_LOOP('',(#19007,#19008,#19009,#19010));
#4075=EDGE_LOOP('',(#19011,#19012,#19013,#19014));
#4076=EDGE_LOOP('',(#19015,#19016,#19017,#19018));
#4077=EDGE_LOOP('',(#19019,#19020,#19021,#19022));
#4078=EDGE_LOOP('',(#19023,#19024,#19025,#19026));
#4079=EDGE_LOOP('',(#19027,#19028,#19029,#19030));
#4080=EDGE_LOOP('',(#19031,#19032,#19033,#19034));
#4081=EDGE_LOOP('',(#19035,#19036,#19037,#19038));
#4082=EDGE_LOOP('',(#19039,#19040,#19041,#19042));
#4083=EDGE_LOOP('',(#19043,#19044,#19045,#19046));
#4084=EDGE_LOOP('',(#19047,#19048,#19049,#19050));
#4085=EDGE_LOOP('',(#19051,#19052,#19053,#19054));
#4086=EDGE_LOOP('',(#19055,#19056,#19057,#19058));
#4087=EDGE_LOOP('',(#19059,#19060,#19061,#19062));
#4088=EDGE_LOOP('',(#19063,#19064,#19065,#19066));
#4089=EDGE_LOOP('',(#19067,#19068,#19069,#19070));
#4090=EDGE_LOOP('',(#19071,#19072,#19073,#19074,#19075,#19076,#19077,#19078,
#19079,#19080,#19081,#19082,#19083,#19084,#19085,#19086,#19087,#19088,#19089,
#19090,#19091,#19092,#19093,#19094,#19095,#19096,#19097,#19098,#19099,#19100,
#19101,#19102,#19103,#19104,#19105,#19106,#19107,#19108,#19109,#19110,#19111,
#19112,#19113,#19114,#19115,#19116,#19117,#19118,#19119,#19120,#19121,#19122,
#19123,#19124,#19125,#19126,#19127,#19128,#19129,#19130,#19131,#19132,#19133,
#19134,#19135,#19136,#19137,#19138,#19139,#19140,#19141,#19142,#19143,#19144,
#19145,#19146,#19147,#19148,#19149,#19150,#19151,#19152,#19153,#19154,#19155,
#19156,#19157,#19158,#19159,#19160,#19161,#19162,#19163,#19164,#19165,#19166));
#4091=EDGE_LOOP('',(#19167));
#4092=EDGE_LOOP('',(#19168,#19169,#19170,#19171));
#4093=EDGE_LOOP('',(#19172,#19173,#19174,#19175));
#4094=EDGE_LOOP('',(#19176,#19177,#19178,#19179));
#4095=EDGE_LOOP('',(#19180,#19181,#19182,#19183));
#4096=EDGE_LOOP('',(#19184,#19185,#19186,#19187));
#4097=EDGE_LOOP('',(#19188,#19189,#19190,#19191));
#4098=EDGE_LOOP('',(#19192,#19193,#19194,#19195));
#4099=EDGE_LOOP('',(#19196));
#4100=EDGE_LOOP('',(#19197));
#4101=EDGE_LOOP('',(#19198,#19199,#19200,#19201));
#4102=EDGE_LOOP('',(#19202));
#4103=EDGE_LOOP('',(#19203));
#4104=EDGE_LOOP('',(#19204,#19205,#19206,#19207));
#4105=EDGE_LOOP('',(#19208,#19209,#19210,#19211));
#5653=LINE('',#37134,#8164);
#5654=LINE('',#37136,#8165);
#5655=LINE('',#37138,#8166);
#5656=LINE('',#37139,#8167);
#5657=LINE('',#37145,#8168);
#5658=LINE('',#37148,#8169);
#5659=LINE('',#37291,#8170);
#5660=LINE('',#37295,#8171);
#5661=LINE('',#37296,#8172);
#5662=LINE('',#37297,#8173);
#5663=LINE('',#37442,#8174);
#5664=LINE('',#37518,#8175);
#5665=LINE('',#37522,#8176);
#5666=LINE('',#37598,#8177);
#5667=LINE('',#37602,#8178);
#5668=LINE('',#37678,#8179);
#5669=LINE('',#37682,#8180);
#5670=LINE('',#37758,#8181);
#5671=LINE('',#37762,#8182);
#5672=LINE('',#37838,#8183);
#5673=LINE('',#37842,#8184);
#5674=LINE('',#37918,#8185);
#5675=LINE('',#37922,#8186);
#5676=LINE('',#37998,#8187);
#5677=LINE('',#38002,#8188);
#5678=LINE('',#38078,#8189);
#5679=LINE('',#38082,#8190);
#5680=LINE('',#38158,#8191);
#5681=LINE('',#38162,#8192);
#5682=LINE('',#38238,#8193);
#5683=LINE('',#38242,#8194);
#5684=LINE('',#38318,#8195);
#5685=LINE('',#38322,#8196);
#5686=LINE('',#38398,#8197);
#5687=LINE('',#38402,#8198);
#5688=LINE('',#38478,#8199);
#5689=LINE('',#38482,#8200);
#5690=LINE('',#38558,#8201);
#5691=LINE('',#38562,#8202);
#5692=LINE('',#38638,#8203);
#5693=LINE('',#38645,#8204);
#5694=LINE('',#38648,#8205);
#5695=LINE('',#38649,#8206);
#5696=LINE('',#38652,#8207);
#5697=LINE('',#38655,#8208);
#5698=LINE('',#38762,#8209);
#5699=LINE('',#38765,#8210);
#5700=LINE('',#38766,#8211);
#5701=LINE('',#38875,#8212);
#5702=LINE('',#38878,#8213);
#5703=LINE('',#38879,#8214);
#5704=LINE('',#38882,#8215);
#5705=LINE('',#38885,#8216);
#5706=LINE('',#38992,#8217);
#5707=LINE('',#38995,#8218);
#5708=LINE('',#38996,#8219);
#5709=LINE('',#39105,#8220);
#5710=LINE('',#39108,#8221);
#5711=LINE('',#39109,#8222);
#5712=LINE('',#39112,#8223);
#5713=LINE('',#39115,#8224);
#5714=LINE('',#39222,#8225);
#5715=LINE('',#39225,#8226);
#5716=LINE('',#39226,#8227);
#5717=LINE('',#39335,#8228);
#5718=LINE('',#39338,#8229);
#5719=LINE('',#39339,#8230);
#5720=LINE('',#39342,#8231);
#5721=LINE('',#39345,#8232);
#5722=LINE('',#39452,#8233);
#5723=LINE('',#39455,#8234);
#5724=LINE('',#39456,#8235);
#5725=LINE('',#39565,#8236);
#5726=LINE('',#39568,#8237);
#5727=LINE('',#39569,#8238);
#5728=LINE('',#39572,#8239);
#5729=LINE('',#39575,#8240);
#5730=LINE('',#39682,#8241);
#5731=LINE('',#39685,#8242);
#5732=LINE('',#39686,#8243);
#5733=LINE('',#39795,#8244);
#5734=LINE('',#39798,#8245);
#5735=LINE('',#39799,#8246);
#5736=LINE('',#39802,#8247);
#5737=LINE('',#39805,#8248);
#5738=LINE('',#39912,#8249);
#5739=LINE('',#39915,#8250);
#5740=LINE('',#39916,#8251);
#5741=LINE('',#40025,#8252);
#5742=LINE('',#40028,#8253);
#5743=LINE('',#40029,#8254);
#5744=LINE('',#40032,#8255);
#5745=LINE('',#40035,#8256);
#5746=LINE('',#40142,#8257);
#5747=LINE('',#40145,#8258);
#5748=LINE('',#40146,#8259);
#5749=LINE('',#40255,#8260);
#5750=LINE('',#40258,#8261);
#5751=LINE('',#40259,#8262);
#5752=LINE('',#40262,#8263);
#5753=LINE('',#40265,#8264);
#5754=LINE('',#40372,#8265);
#5755=LINE('',#40375,#8266);
#5756=LINE('',#40376,#8267);
#5757=LINE('',#40485,#8268);
#5758=LINE('',#40488,#8269);
#5759=LINE('',#40489,#8270);
#5760=LINE('',#40492,#8271);
#5761=LINE('',#40495,#8272);
#5762=LINE('',#40602,#8273);
#5763=LINE('',#40605,#8274);
#5764=LINE('',#40606,#8275);
#5765=LINE('',#40715,#8276);
#5766=LINE('',#40718,#8277);
#5767=LINE('',#40719,#8278);
#5768=LINE('',#40722,#8279);
#5769=LINE('',#40725,#8280);
#5770=LINE('',#40832,#8281);
#5771=LINE('',#40835,#8282);
#5772=LINE('',#40836,#8283);
#5773=LINE('',#40945,#8284);
#5774=LINE('',#40948,#8285);
#5775=LINE('',#40949,#8286);
#5776=LINE('',#40952,#8287);
#5777=LINE('',#40955,#8288);
#5778=LINE('',#41062,#8289);
#5779=LINE('',#41065,#8290);
#5780=LINE('',#41066,#8291);
#5781=LINE('',#41175,#8292);
#5782=LINE('',#41178,#8293);
#5783=LINE('',#41179,#8294);
#5784=LINE('',#41182,#8295);
#5785=LINE('',#41185,#8296);
#5786=LINE('',#41292,#8297);
#5787=LINE('',#41295,#8298);
#5788=LINE('',#41296,#8299);
#5789=LINE('',#41405,#8300);
#5790=LINE('',#41408,#8301);
#5791=LINE('',#41409,#8302);
#5792=LINE('',#41412,#8303);
#5793=LINE('',#41415,#8304);
#5794=LINE('',#41522,#8305);
#5795=LINE('',#41525,#8306);
#5796=LINE('',#41526,#8307);
#5797=LINE('',#41635,#8308);
#5798=LINE('',#41638,#8309);
#5799=LINE('',#41640,#8310);
#5800=LINE('',#41641,#8311);
#5801=LINE('',#41644,#8312);
#5802=LINE('',#41645,#8313);
#5803=LINE('',#41648,#8314);
#5804=LINE('',#41651,#8315);
#5805=LINE('',#41866,#8316);
#5806=LINE('',#41942,#8317);
#5807=LINE('',#41947,#8318);
#5808=LINE('',#41949,#8319);
#5809=LINE('',#41951,#8320);
#5810=LINE('',#41952,#8321);
#5811=LINE('',#42024,#8322);
#5812=LINE('',#42025,#8323);
#5813=LINE('',#42105,#8324);
#5814=LINE('',#42110,#8325);
#5815=LINE('',#42112,#8326);
#8164=VECTOR('',#30345,10.);
#8165=VECTOR('',#30346,10.);
#8166=VECTOR('',#30347,10.);
#8167=VECTOR('',#30348,10.);
#8168=VECTOR('',#30353,10.);
#8169=VECTOR('',#30356,10.);
#8170=VECTOR('',#30357,10.);
#8171=VECTOR('',#30360,10.);
#8172=VECTOR('',#30361,10.);
#8173=VECTOR('',#30362,10.);
#8174=VECTOR('',#30367,10.);
#8175=VECTOR('',#30370,10.);
#8176=VECTOR('',#30373,9.99999999999999);
#8177=VECTOR('',#30376,10.);
#8178=VECTOR('',#30379,10.);
#8179=VECTOR('',#30382,10.);
#8180=VECTOR('',#30385,10.);
#8181=VECTOR('',#30388,10.);
#8182=VECTOR('',#30391,10.);
#8183=VECTOR('',#30394,10.);
#8184=VECTOR('',#30397,10.);
#8185=VECTOR('',#30400,10.);
#8186=VECTOR('',#30403,10.);
#8187=VECTOR('',#30406,10.);
#8188=VECTOR('',#30409,10.);
#8189=VECTOR('',#30412,10.);
#8190=VECTOR('',#30415,10.);
#8191=VECTOR('',#30418,10.);
#8192=VECTOR('',#30421,10.);
#8193=VECTOR('',#30424,10.);
#8194=VECTOR('',#30427,10.);
#8195=VECTOR('',#30430,10.);
#8196=VECTOR('',#30433,10.);
#8197=VECTOR('',#30436,10.);
#8198=VECTOR('',#30439,10.);
#8199=VECTOR('',#30442,10.);
#8200=VECTOR('',#30445,10.);
#8201=VECTOR('',#30448,10.);
#8202=VECTOR('',#30451,10.);
#8203=VECTOR('',#30454,10.);
#8204=VECTOR('',#30463,10.);
#8205=VECTOR('',#30466,10.);
#8206=VECTOR('',#30467,10.);
#8207=VECTOR('',#30470,10.);
#8208=VECTOR('',#30473,10.);
#8209=VECTOR('',#30474,10.);
#8210=VECTOR('',#30477,10.);
#8211=VECTOR('',#30478,10.);
#8212=VECTOR('',#30483,10.);
#8213=VECTOR('',#30486,9.99999999999999);
#8214=VECTOR('',#30487,10.);
#8215=VECTOR('',#30490,10.);
#8216=VECTOR('',#30493,10.);
#8217=VECTOR('',#30494,10.);
#8218=VECTOR('',#30497,10.);
#8219=VECTOR('',#30498,10.);
#8220=VECTOR('',#30503,10.);
#8221=VECTOR('',#30506,10.);
#8222=VECTOR('',#30507,10.);
#8223=VECTOR('',#30510,10.);
#8224=VECTOR('',#30513,10.);
#8225=VECTOR('',#30514,10.);
#8226=VECTOR('',#30517,10.);
#8227=VECTOR('',#30518,10.);
#8228=VECTOR('',#30523,10.);
#8229=VECTOR('',#30526,10.);
#8230=VECTOR('',#30527,10.);
#8231=VECTOR('',#30530,10.);
#8232=VECTOR('',#30533,10.);
#8233=VECTOR('',#30534,10.);
#8234=VECTOR('',#30537,10.);
#8235=VECTOR('',#30538,10.);
#8236=VECTOR('',#30543,10.);
#8237=VECTOR('',#30546,10.);
#8238=VECTOR('',#30547,10.);
#8239=VECTOR('',#30550,10.);
#8240=VECTOR('',#30553,10.);
#8241=VECTOR('',#30554,10.);
#8242=VECTOR('',#30557,10.);
#8243=VECTOR('',#30558,10.);
#8244=VECTOR('',#30563,10.);
#8245=VECTOR('',#30566,10.);
#8246=VECTOR('',#30567,10.);
#8247=VECTOR('',#30570,10.);
#8248=VECTOR('',#30573,10.);
#8249=VECTOR('',#30574,10.);
#8250=VECTOR('',#30577,10.);
#8251=VECTOR('',#30578,10.);
#8252=VECTOR('',#30583,10.);
#8253=VECTOR('',#30586,10.);
#8254=VECTOR('',#30587,10.);
#8255=VECTOR('',#30590,10.);
#8256=VECTOR('',#30593,10.);
#8257=VECTOR('',#30594,10.);
#8258=VECTOR('',#30597,10.);
#8259=VECTOR('',#30598,10.);
#8260=VECTOR('',#30603,10.);
#8261=VECTOR('',#30606,10.);
#8262=VECTOR('',#30607,10.);
#8263=VECTOR('',#30610,10.);
#8264=VECTOR('',#30613,10.);
#8265=VECTOR('',#30614,10.);
#8266=VECTOR('',#30617,10.);
#8267=VECTOR('',#30618,10.);
#8268=VECTOR('',#30623,10.);
#8269=VECTOR('',#30626,10.);
#8270=VECTOR('',#30627,10.);
#8271=VECTOR('',#30630,10.);
#8272=VECTOR('',#30633,10.);
#8273=VECTOR('',#30634,10.);
#8274=VECTOR('',#30637,10.);
#8275=VECTOR('',#30638,10.);
#8276=VECTOR('',#30643,10.);
#8277=VECTOR('',#30646,10.);
#8278=VECTOR('',#30647,10.);
#8279=VECTOR('',#30650,10.);
#8280=VECTOR('',#30653,10.);
#8281=VECTOR('',#30654,10.);
#8282=VECTOR('',#30657,10.);
#8283=VECTOR('',#30658,10.);
#8284=VECTOR('',#30663,10.);
#8285=VECTOR('',#30666,10.);
#8286=VECTOR('',#30667,10.);
#8287=VECTOR('',#30670,10.);
#8288=VECTOR('',#30673,10.);
#8289=VECTOR('',#30674,10.);
#8290=VECTOR('',#30677,10.);
#8291=VECTOR('',#30678,10.);
#8292=VECTOR('',#30683,10.);
#8293=VECTOR('',#30686,10.);
#8294=VECTOR('',#30687,10.);
#8295=VECTOR('',#30690,10.);
#8296=VECTOR('',#30693,10.);
#8297=VECTOR('',#30694,10.);
#8298=VECTOR('',#30697,10.);
#8299=VECTOR('',#30698,10.);
#8300=VECTOR('',#30703,10.);
#8301=VECTOR('',#30706,10.);
#8302=VECTOR('',#30707,10.);
#8303=VECTOR('',#30710,10.);
#8304=VECTOR('',#30713,10.);
#8305=VECTOR('',#30714,10.);
#8306=VECTOR('',#30717,10.);
#8307=VECTOR('',#30718,10.);
#8308=VECTOR('',#30723,10.);
#8309=VECTOR('',#30726,10.);
#8310=VECTOR('',#30727,10.);
#8311=VECTOR('',#30728,10.);
#8312=VECTOR('',#30731,10.);
#8313=VECTOR('',#30732,10.);
#8314=VECTOR('',#30735,10.);
#8315=VECTOR('',#30738,10.);
#8316=VECTOR('',#30743,10.);
#8317=VECTOR('',#30746,10.);
#8318=VECTOR('',#30753,10.);
#8319=VECTOR('',#30756,10.);
#8320=VECTOR('',#30759,10.);
#8321=VECTOR('',#30760,10.);
#8322=VECTOR('',#30763,10.);
#8323=VECTOR('',#30764,10.);
#8324=VECTOR('',#30777,1.6);
#8325=VECTOR('',#30784,4.477);
#8326=VECTOR('',#30787,3.261);
#10439=CIRCLE('',#27456,7.14399999999837);
#10440=CIRCLE('',#27457,7.14399999999837);
#10441=CIRCLE('',#27460,5.358);
#10442=CIRCLE('',#27461,7.14399999999837);
#10443=CIRCLE('',#27462,5.358);
#10444=CIRCLE('',#27463,7.14399999999837);
#10445=CIRCLE('',#27464,5.358);
#10446=CIRCLE('',#27465,7.14399999999837);
#10447=CIRCLE('',#27466,5.358);
#10448=CIRCLE('',#27467,7.14399999999837);
#10449=CIRCLE('',#27468,5.358);
#10450=CIRCLE('',#27469,7.14399999999837);
#10451=CIRCLE('',#27470,5.358);
#10452=CIRCLE('',#27471,7.14399999999837);
#10453=CIRCLE('',#27472,5.358);
#10454=CIRCLE('',#27473,7.14399999999837);
#10455=CIRCLE('',#27474,5.358);
#10456=CIRCLE('',#27475,7.14399999999837);
#10457=CIRCLE('',#27476,5.358);
#10458=CIRCLE('',#27477,7.14399999999837);
#10459=CIRCLE('',#27478,5.358);
#10460=CIRCLE('',#27479,7.14399999999837);
#10461=CIRCLE('',#27480,5.358);
#10462=CIRCLE('',#27481,7.14399999999837);
#10463=CIRCLE('',#27482,5.358);
#10464=CIRCLE('',#27483,7.14399999999837);
#10465=CIRCLE('',#27484,5.358);
#10466=CIRCLE('',#27485,7.14399999999837);
#10467=CIRCLE('',#27486,5.358);
#10468=CIRCLE('',#27487,7.14399999999837);
#10469=CIRCLE('',#27488,5.358);
#10470=CIRCLE('',#27489,7.14399999999837);
#10471=CIRCLE('',#27490,5.358);
#10472=CIRCLE('',#27491,4.477);
#10473=CIRCLE('',#27493,5.358);
#10474=CIRCLE('',#27496,7.14399999999837);
#10475=CIRCLE('',#27499,5.358);
#10476=CIRCLE('',#27502,7.14399999999837);
#10477=CIRCLE('',#27505,5.358);
#10478=CIRCLE('',#27508,7.14399999999837);
#10479=CIRCLE('',#27511,5.358);
#10480=CIRCLE('',#27514,7.14399999999837);
#10481=CIRCLE('',#27517,5.358);
#10482=CIRCLE('',#27520,7.14399999999837);
#10483=CIRCLE('',#27523,5.358);
#10484=CIRCLE('',#27526,7.14399999999837);
#10485=CIRCLE('',#27529,5.358);
#10486=CIRCLE('',#27532,7.14399999999837);
#10487=CIRCLE('',#27535,5.358);
#10488=CIRCLE('',#27538,7.14399999999837);
#10489=CIRCLE('',#27541,5.358);
#10490=CIRCLE('',#27544,7.14399999999837);
#10491=CIRCLE('',#27547,5.358);
#10492=CIRCLE('',#27550,7.14399999999837);
#10493=CIRCLE('',#27553,5.358);
#10494=CIRCLE('',#27556,7.14399999999837);
#10495=CIRCLE('',#27559,5.358);
#10496=CIRCLE('',#27562,7.14399999999837);
#10497=CIRCLE('',#27565,5.358);
#10498=CIRCLE('',#27568,7.14399999999837);
#10499=CIRCLE('',#27571,5.358);
#10500=CIRCLE('',#27575,7.14399999999837);
#10501=CIRCLE('',#27577,5.358);
#10502=CIRCLE('',#27578,7.14399999999837);
#10503=CIRCLE('',#27579,5.358);
#10504=CIRCLE('',#27580,3.261);
#10505=CIRCLE('',#27587,3.261);
#10506=CIRCLE('',#27588,1.6);
#10507=CIRCLE('',#27590,1.6);
#10508=CIRCLE('',#27592,4.477);
#11370=VERTEX_POINT('',#37132);
#11371=VERTEX_POINT('',#37133);
#11372=VERTEX_POINT('',#37135);
#11373=VERTEX_POINT('',#37137);
#11374=VERTEX_POINT('',#37141);
#11375=VERTEX_POINT('',#37142);
#11376=VERTEX_POINT('',#37144);
#11377=VERTEX_POINT('',#37146);
#11378=VERTEX_POINT('',#37219);
#11379=VERTEX_POINT('',#37255);
#11380=VERTEX_POINT('',#37293);
#11381=VERTEX_POINT('',#37294);
#11382=VERTEX_POINT('',#37439);
#11383=VERTEX_POINT('',#37441);
#11384=VERTEX_POINT('',#37443);
#11385=VERTEX_POINT('',#37479);
#11386=VERTEX_POINT('',#37481);
#11387=VERTEX_POINT('',#37517);
#11388=VERTEX_POINT('',#37519);
#11389=VERTEX_POINT('',#37521);
#11390=VERTEX_POINT('',#37523);
#11391=VERTEX_POINT('',#37559);
#11392=VERTEX_POINT('',#37561);
#11393=VERTEX_POINT('',#37597);
#11394=VERTEX_POINT('',#37599);
#11395=VERTEX_POINT('',#37601);
#11396=VERTEX_POINT('',#37603);
#11397=VERTEX_POINT('',#37639);
#11398=VERTEX_POINT('',#37641);
#11399=VERTEX_POINT('',#37677);
#11400=VERTEX_POINT('',#37679);
#11401=VERTEX_POINT('',#37681);
#11402=VERTEX_POINT('',#37683);
#11403=VERTEX_POINT('',#37719);
#11404=VERTEX_POINT('',#37721);
#11405=VERTEX_POINT('',#37757);
#11406=VERTEX_POINT('',#37759);
#11407=VERTEX_POINT('',#37761);
#11408=VERTEX_POINT('',#37763);
#11409=VERTEX_POINT('',#37799);
#11410=VERTEX_POINT('',#37801);
#11411=VERTEX_POINT('',#37837);
#11412=VERTEX_POINT('',#37839);
#11413=VERTEX_POINT('',#37841);
#11414=VERTEX_POINT('',#37843);
#11415=VERTEX_POINT('',#37879);
#11416=VERTEX_POINT('',#37881);
#11417=VERTEX_POINT('',#37917);
#11418=VERTEX_POINT('',#37919);
#11419=VERTEX_POINT('',#37921);
#11420=VERTEX_POINT('',#37923);
#11421=VERTEX_POINT('',#37959);
#11422=VERTEX_POINT('',#37961);
#11423=VERTEX_POINT('',#37997);
#11424=VERTEX_POINT('',#37999);
#11425=VERTEX_POINT('',#38001);
#11426=VERTEX_POINT('',#38003);
#11427=VERTEX_POINT('',#38039);
#11428=VERTEX_POINT('',#38041);
#11429=VERTEX_POINT('',#38077);
#11430=VERTEX_POINT('',#38079);
#11431=VERTEX_POINT('',#38081);
#11432=VERTEX_POINT('',#38083);
#11433=VERTEX_POINT('',#38119);
#11434=VERTEX_POINT('',#38121);
#11435=VERTEX_POINT('',#38157);
#11436=VERTEX_POINT('',#38159);
#11437=VERTEX_POINT('',#38161);
#11438=VERTEX_POINT('',#38163);
#11439=VERTEX_POINT('',#38199);
#11440=VERTEX_POINT('',#38201);
#11441=VERTEX_POINT('',#38237);
#11442=VERTEX_POINT('',#38239);
#11443=VERTEX_POINT('',#38241);
#11444=VERTEX_POINT('',#38243);
#11445=VERTEX_POINT('',#38279);
#11446=VERTEX_POINT('',#38281);
#11447=VERTEX_POINT('',#38317);
#11448=VERTEX_POINT('',#38319);
#11449=VERTEX_POINT('',#38321);
#11450=VERTEX_POINT('',#38323);
#11451=VERTEX_POINT('',#38359);
#11452=VERTEX_POINT('',#38361);
#11453=VERTEX_POINT('',#38397);
#11454=VERTEX_POINT('',#38399);
#11455=VERTEX_POINT('',#38401);
#11456=VERTEX_POINT('',#38403);
#11457=VERTEX_POINT('',#38439);
#11458=VERTEX_POINT('',#38441);
#11459=VERTEX_POINT('',#38477);
#11460=VERTEX_POINT('',#38479);
#11461=VERTEX_POINT('',#38481);
#11462=VERTEX_POINT('',#38483);
#11463=VERTEX_POINT('',#38519);
#11464=VERTEX_POINT('',#38521);
#11465=VERTEX_POINT('',#38557);
#11466=VERTEX_POINT('',#38559);
#11467=VERTEX_POINT('',#38561);
#11468=VERTEX_POINT('',#38563);
#11469=VERTEX_POINT('',#38599);
#11470=VERTEX_POINT('',#38601);
#11471=VERTEX_POINT('',#38637);
#11472=VERTEX_POINT('',#38640);
#11473=VERTEX_POINT('',#38643);
#11474=VERTEX_POINT('',#38647);
#11475=VERTEX_POINT('',#38651);
#11476=VERTEX_POINT('',#38653);
#11477=VERTEX_POINT('',#38726);
#11478=VERTEX_POINT('',#38764);
#11479=VERTEX_POINT('',#38873);
#11480=VERTEX_POINT('',#38877);
#11481=VERTEX_POINT('',#38881);
#11482=VERTEX_POINT('',#38883);
#11483=VERTEX_POINT('',#38956);
#11484=VERTEX_POINT('',#38994);
#11485=VERTEX_POINT('',#39103);
#11486=VERTEX_POINT('',#39107);
#11487=VERTEX_POINT('',#39111);
#11488=VERTEX_POINT('',#39113);
#11489=VERTEX_POINT('',#39186);
#11490=VERTEX_POINT('',#39224);
#11491=VERTEX_POINT('',#39333);
#11492=VERTEX_POINT('',#39337);
#11493=VERTEX_POINT('',#39341);
#11494=VERTEX_POINT('',#39343);
#11495=VERTEX_POINT('',#39416);
#11496=VERTEX_POINT('',#39454);
#11497=VERTEX_POINT('',#39563);
#11498=VERTEX_POINT('',#39567);
#11499=VERTEX_POINT('',#39571);
#11500=VERTEX_POINT('',#39573);
#11501=VERTEX_POINT('',#39646);
#11502=VERTEX_POINT('',#39684);
#11503=VERTEX_POINT('',#39793);
#11504=VERTEX_POINT('',#39797);
#11505=VERTEX_POINT('',#39801);
#11506=VERTEX_POINT('',#39803);
#11507=VERTEX_POINT('',#39876);
#11508=VERTEX_POINT('',#39914);
#11509=VERTEX_POINT('',#40023);
#11510=VERTEX_POINT('',#40027);
#11511=VERTEX_POINT('',#40031);
#11512=VERTEX_POINT('',#40033);
#11513=VERTEX_POINT('',#40106);
#11514=VERTEX_POINT('',#40144);
#11515=VERTEX_POINT('',#40253);
#11516=VERTEX_POINT('',#40257);
#11517=VERTEX_POINT('',#40261);
#11518=VERTEX_POINT('',#40263);
#11519=VERTEX_POINT('',#40336);
#11520=VERTEX_POINT('',#40374);
#11521=VERTEX_POINT('',#40483);
#11522=VERTEX_POINT('',#40487);
#11523=VERTEX_POINT('',#40491);
#11524=VERTEX_POINT('',#40493);
#11525=VERTEX_POINT('',#40566);
#11526=VERTEX_POINT('',#40604);
#11527=VERTEX_POINT('',#40713);
#11528=VERTEX_POINT('',#40717);
#11529=VERTEX_POINT('',#40721);
#11530=VERTEX_POINT('',#40723);
#11531=VERTEX_POINT('',#40796);
#11532=VERTEX_POINT('',#40834);
#11533=VERTEX_POINT('',#40943);
#11534=VERTEX_POINT('',#40947);
#11535=VERTEX_POINT('',#40951);
#11536=VERTEX_POINT('',#40953);
#11537=VERTEX_POINT('',#41026);
#11538=VERTEX_POINT('',#41064);
#11539=VERTEX_POINT('',#41173);
#11540=VERTEX_POINT('',#41177);
#11541=VERTEX_POINT('',#41181);
#11542=VERTEX_POINT('',#41183);
#11543=VERTEX_POINT('',#41256);
#11544=VERTEX_POINT('',#41294);
#11545=VERTEX_POINT('',#41403);
#11546=VERTEX_POINT('',#41407);
#11547=VERTEX_POINT('',#41411);
#11548=VERTEX_POINT('',#41413);
#11549=VERTEX_POINT('',#41486);
#11550=VERTEX_POINT('',#41524);
#11551=VERTEX_POINT('',#41633);
#11552=VERTEX_POINT('',#41637);
#11553=VERTEX_POINT('',#41639);
#11554=VERTEX_POINT('',#41643);
#11555=VERTEX_POINT('',#41647);
#11556=VERTEX_POINT('',#41649);
#11557=VERTEX_POINT('',#41863);
#11558=VERTEX_POINT('',#41865);
#11559=VERTEX_POINT('',#41867);
#11560=VERTEX_POINT('',#41903);
#11561=VERTEX_POINT('',#41905);
#11562=VERTEX_POINT('',#41941);
#11563=VERTEX_POINT('',#41944);
#11564=VERTEX_POINT('',#42098);
#11565=VERTEX_POINT('',#42100);
#11566=VERTEX_POINT('',#42103);
#11567=VERTEX_POINT('',#42107);
#14170=EDGE_CURVE('',#11370,#11371,#5653,.T.);
#14171=EDGE_CURVE('',#11372,#11370,#5654,.T.);
#14172=EDGE_CURVE('',#11373,#11372,#5655,.T.);
#14173=EDGE_CURVE('',#11373,#11371,#5656,.T.);
#14174=EDGE_CURVE('',#11374,#11375,#10439,.T.);
#14175=EDGE_CURVE('',#11374,#11376,#5657,.T.);
#14176=EDGE_CURVE('',#11377,#11376,#10440,.T.);
#14177=EDGE_CURVE('',#11375,#11377,#5658,.T.);
#14178=EDGE_CURVE('',#11378,#11375,#508,.T.);
#14179=EDGE_CURVE('',#11379,#11377,#509,.T.);
#14180=EDGE_CURVE('',#11378,#11379,#5659,.T.);
#14181=EDGE_CURVE('',#11380,#11381,#5660,.T.);
#14182=EDGE_CURVE('',#11380,#11378,#5661,.T.);
#14183=EDGE_CURVE('',#11381,#11379,#5662,.T.);
#14184=EDGE_CURVE('',#11373,#11374,#510,.T.);
#14185=EDGE_CURVE('',#11376,#11372,#511,.T.);
#14186=EDGE_CURVE('',#11382,#11380,#10441,.T.);
#14187=EDGE_CURVE('',#11383,#11382,#5663,.T.);
#14188=EDGE_CURVE('',#11383,#11384,#512,.T.);
#14189=EDGE_CURVE('',#11384,#11385,#10442,.T.);
#14190=EDGE_CURVE('',#11386,#11385,#513,.T.);
#14191=EDGE_CURVE('',#11387,#11386,#5664,.T.);
#14192=EDGE_CURVE('',#11388,#11387,#10443,.T.);
#14193=EDGE_CURVE('',#11389,#11388,#5665,.T.);
#14194=EDGE_CURVE('',#11389,#11390,#514,.T.);
#14195=EDGE_CURVE('',#11390,#11391,#10444,.T.);
#14196=EDGE_CURVE('',#11392,#11391,#515,.T.);
#14197=EDGE_CURVE('',#11393,#11392,#5666,.T.);
#14198=EDGE_CURVE('',#11394,#11393,#10445,.T.);
#14199=EDGE_CURVE('',#11395,#11394,#5667,.T.);
#14200=EDGE_CURVE('',#11395,#11396,#516,.T.);
#14201=EDGE_CURVE('',#11396,#11397,#10446,.T.);
#14202=EDGE_CURVE('',#11398,#11397,#517,.T.);
#14203=EDGE_CURVE('',#11399,#11398,#5668,.T.);
#14204=EDGE_CURVE('',#11400,#11399,#10447,.T.);
#14205=EDGE_CURVE('',#11401,#11400,#5669,.T.);
#14206=EDGE_CURVE('',#11401,#11402,#518,.T.);
#14207=EDGE_CURVE('',#11402,#11403,#10448,.T.);
#14208=EDGE_CURVE('',#11404,#11403,#519,.T.);
#14209=EDGE_CURVE('',#11405,#11404,#5670,.T.);
#14210=EDGE_CURVE('',#11406,#11405,#10449,.T.);
#14211=EDGE_CURVE('',#11407,#11406,#5671,.T.);
#14212=EDGE_CURVE('',#11407,#11408,#520,.T.);
#14213=EDGE_CURVE('',#11408,#11409,#10450,.T.);
#14214=EDGE_CURVE('',#11410,#11409,#521,.T.);
#14215=EDGE_CURVE('',#11411,#11410,#5672,.T.);
#14216=EDGE_CURVE('',#11412,#11411,#10451,.T.);
#14217=EDGE_CURVE('',#11413,#11412,#5673,.T.);
#14218=EDGE_CURVE('',#11413,#11414,#522,.T.);
#14219=EDGE_CURVE('',#11414,#11415,#10452,.T.);
#14220=EDGE_CURVE('',#11416,#11415,#523,.T.);
#14221=EDGE_CURVE('',#11417,#11416,#5674,.T.);
#14222=EDGE_CURVE('',#11418,#11417,#10453,.T.);
#14223=EDGE_CURVE('',#11419,#11418,#5675,.T.);
#14224=EDGE_CURVE('',#11419,#11420,#524,.T.);
#14225=EDGE_CURVE('',#11420,#11421,#10454,.T.);
#14226=EDGE_CURVE('',#11422,#11421,#525,.T.);
#14227=EDGE_CURVE('',#11423,#11422,#5676,.T.);
#14228=EDGE_CURVE('',#11424,#11423,#10455,.T.);
#14229=EDGE_CURVE('',#11425,#11424,#5677,.T.);
#14230=EDGE_CURVE('',#11425,#11426,#526,.T.);
#14231=EDGE_CURVE('',#11426,#11427,#10456,.T.);
#14232=EDGE_CURVE('',#11428,#11427,#527,.T.);
#14233=EDGE_CURVE('',#11429,#11428,#5678,.T.);
#14234=EDGE_CURVE('',#11430,#11429,#10457,.T.);
#14235=EDGE_CURVE('',#11431,#11430,#5679,.T.);
#14236=EDGE_CURVE('',#11431,#11432,#528,.T.);
#14237=EDGE_CURVE('',#11432,#11433,#10458,.T.);
#14238=EDGE_CURVE('',#11434,#11433,#529,.T.);
#14239=EDGE_CURVE('',#11435,#11434,#5680,.T.);
#14240=EDGE_CURVE('',#11436,#11435,#10459,.T.);
#14241=EDGE_CURVE('',#11437,#11436,#5681,.T.);
#14242=EDGE_CURVE('',#11437,#11438,#530,.T.);
#14243=EDGE_CURVE('',#11438,#11439,#10460,.T.);
#14244=EDGE_CURVE('',#11440,#11439,#531,.T.);
#14245=EDGE_CURVE('',#11441,#11440,#5682,.T.);
#14246=EDGE_CURVE('',#11442,#11441,#10461,.T.);
#14247=EDGE_CURVE('',#11443,#11442,#5683,.T.);
#14248=EDGE_CURVE('',#11443,#11444,#532,.T.);
#14249=EDGE_CURVE('',#11444,#11445,#10462,.T.);
#14250=EDGE_CURVE('',#11446,#11445,#533,.T.);
#14251=EDGE_CURVE('',#11447,#11446,#5684,.T.);
#14252=EDGE_CURVE('',#11448,#11447,#10463,.T.);
#14253=EDGE_CURVE('',#11449,#11448,#5685,.T.);
#14254=EDGE_CURVE('',#11449,#11450,#534,.T.);
#14255=EDGE_CURVE('',#11450,#11451,#10464,.T.);
#14256=EDGE_CURVE('',#11452,#11451,#535,.T.);
#14257=EDGE_CURVE('',#11453,#11452,#5686,.T.);
#14258=EDGE_CURVE('',#11454,#11453,#10465,.T.);
#14259=EDGE_CURVE('',#11455,#11454,#5687,.T.);
#14260=EDGE_CURVE('',#11455,#11456,#536,.T.);
#14261=EDGE_CURVE('',#11456,#11457,#10466,.T.);
#14262=EDGE_CURVE('',#11458,#11457,#537,.T.);
#14263=EDGE_CURVE('',#11459,#11458,#5688,.T.);
#14264=EDGE_CURVE('',#11460,#11459,#10467,.T.);
#14265=EDGE_CURVE('',#11461,#11460,#5689,.T.);
#14266=EDGE_CURVE('',#11461,#11462,#538,.T.);
#14267=EDGE_CURVE('',#11462,#11463,#10468,.T.);
#14268=EDGE_CURVE('',#11464,#11463,#539,.T.);
#14269=EDGE_CURVE('',#11465,#11464,#5690,.T.);
#14270=EDGE_CURVE('',#11466,#11465,#10469,.T.);
#14271=EDGE_CURVE('',#11467,#11466,#5691,.T.);
#14272=EDGE_CURVE('',#11467,#11468,#540,.T.);
#14273=EDGE_CURVE('',#11468,#11469,#10470,.T.);
#14274=EDGE_CURVE('',#11470,#11469,#541,.T.);
#14275=EDGE_CURVE('',#11471,#11470,#5692,.T.);
#14276=EDGE_CURVE('',#11371,#11471,#10471,.T.);
#14277=EDGE_CURVE('',#11472,#11472,#10472,.T.);
#14278=EDGE_CURVE('',#11473,#11381,#10473,.T.);
#14279=EDGE_CURVE('',#11473,#11382,#5693,.T.);
#14280=EDGE_CURVE('',#11474,#11473,#5694,.T.);
#14281=EDGE_CURVE('',#11383,#11474,#5695,.T.);
#14282=EDGE_CURVE('',#11384,#11475,#5696,.T.);
#14283=EDGE_CURVE('',#11476,#11475,#10474,.T.);
#14284=EDGE_CURVE('',#11385,#11476,#5697,.T.);
#14285=EDGE_CURVE('',#11477,#11476,#542,.T.);
#14286=EDGE_CURVE('',#11386,#11477,#5698,.T.);
#14287=EDGE_CURVE('',#11387,#11478,#5699,.T.);
#14288=EDGE_CURVE('',#11478,#11477,#5700,.T.);
#14289=EDGE_CURVE('',#11475,#11474,#543,.T.);
#14290=EDGE_CURVE('',#11479,#11478,#10475,.T.);
#14291=EDGE_CURVE('',#11479,#11388,#5701,.T.);
#14292=EDGE_CURVE('',#11480,#11479,#5702,.T.);
#14293=EDGE_CURVE('',#11389,#11480,#5703,.T.);
#14294=EDGE_CURVE('',#11390,#11481,#5704,.T.);
#14295=EDGE_CURVE('',#11482,#11481,#10476,.T.);
#14296=EDGE_CURVE('',#11391,#11482,#5705,.T.);
#14297=EDGE_CURVE('',#11483,#11482,#544,.T.);
#14298=EDGE_CURVE('',#11392,#11483,#5706,.T.);
#14299=EDGE_CURVE('',#11393,#11484,#5707,.T.);
#14300=EDGE_CURVE('',#11484,#11483,#5708,.T.);
#14301=EDGE_CURVE('',#11481,#11480,#545,.T.);
#14302=EDGE_CURVE('',#11485,#11484,#10477,.T.);
#14303=EDGE_CURVE('',#11485,#11394,#5709,.T.);
#14304=EDGE_CURVE('',#11486,#11485,#5710,.T.);
#14305=EDGE_CURVE('',#11395,#11486,#5711,.T.);
#14306=EDGE_CURVE('',#11396,#11487,#5712,.T.);
#14307=EDGE_CURVE('',#11488,#11487,#10478,.T.);
#14308=EDGE_CURVE('',#11397,#11488,#5713,.T.);
#14309=EDGE_CURVE('',#11489,#11488,#546,.T.);
#14310=EDGE_CURVE('',#11398,#11489,#5714,.T.);
#14311=EDGE_CURVE('',#11399,#11490,#5715,.T.);
#14312=EDGE_CURVE('',#11490,#11489,#5716,.T.);
#14313=EDGE_CURVE('',#11487,#11486,#547,.T.);
#14314=EDGE_CURVE('',#11491,#11490,#10479,.T.);
#14315=EDGE_CURVE('',#11491,#11400,#5717,.T.);
#14316=EDGE_CURVE('',#11492,#11491,#5718,.T.);
#14317=EDGE_CURVE('',#11401,#11492,#5719,.T.);
#14318=EDGE_CURVE('',#11402,#11493,#5720,.T.);
#14319=EDGE_CURVE('',#11494,#11493,#10480,.T.);
#14320=EDGE_CURVE('',#11403,#11494,#5721,.T.);
#14321=EDGE_CURVE('',#11495,#11494,#548,.T.);
#14322=EDGE_CURVE('',#11404,#11495,#5722,.T.);
#14323=EDGE_CURVE('',#11405,#11496,#5723,.T.);
#14324=EDGE_CURVE('',#11496,#11495,#5724,.T.);
#14325=EDGE_CURVE('',#11493,#11492,#549,.T.);
#14326=EDGE_CURVE('',#11497,#11496,#10481,.T.);
#14327=EDGE_CURVE('',#11497,#11406,#5725,.T.);
#14328=EDGE_CURVE('',#11498,#11497,#5726,.T.);
#14329=EDGE_CURVE('',#11407,#11498,#5727,.T.);
#14330=EDGE_CURVE('',#11408,#11499,#5728,.T.);
#14331=EDGE_CURVE('',#11500,#11499,#10482,.T.);
#14332=EDGE_CURVE('',#11409,#11500,#5729,.T.);
#14333=EDGE_CURVE('',#11501,#11500,#550,.T.);
#14334=EDGE_CURVE('',#11410,#11501,#5730,.T.);
#14335=EDGE_CURVE('',#11411,#11502,#5731,.T.);
#14336=EDGE_CURVE('',#11502,#11501,#5732,.T.);
#14337=EDGE_CURVE('',#11499,#11498,#551,.T.);
#14338=EDGE_CURVE('',#11503,#11502,#10483,.T.);
#14339=EDGE_CURVE('',#11503,#11412,#5733,.T.);
#14340=EDGE_CURVE('',#11504,#11503,#5734,.T.);
#14341=EDGE_CURVE('',#11413,#11504,#5735,.T.);
#14342=EDGE_CURVE('',#11414,#11505,#5736,.T.);
#14343=EDGE_CURVE('',#11506,#11505,#10484,.T.);
#14344=EDGE_CURVE('',#11415,#11506,#5737,.T.);
#14345=EDGE_CURVE('',#11507,#11506,#552,.T.);
#14346=EDGE_CURVE('',#11416,#11507,#5738,.T.);
#14347=EDGE_CURVE('',#11417,#11508,#5739,.T.);
#14348=EDGE_CURVE('',#11508,#11507,#5740,.T.);
#14349=EDGE_CURVE('',#11505,#11504,#553,.T.);
#14350=EDGE_CURVE('',#11509,#11508,#10485,.T.);
#14351=EDGE_CURVE('',#11509,#11418,#5741,.T.);
#14352=EDGE_CURVE('',#11510,#11509,#5742,.T.);
#14353=EDGE_CURVE('',#11419,#11510,#5743,.T.);
#14354=EDGE_CURVE('',#11420,#11511,#5744,.T.);
#14355=EDGE_CURVE('',#11512,#11511,#10486,.T.);
#14356=EDGE_CURVE('',#11421,#11512,#5745,.T.);
#14357=EDGE_CURVE('',#11513,#11512,#554,.T.);
#14358=EDGE_CURVE('',#11422,#11513,#5746,.T.);
#14359=EDGE_CURVE('',#11423,#11514,#5747,.T.);
#14360=EDGE_CURVE('',#11514,#11513,#5748,.T.);
#14361=EDGE_CURVE('',#11511,#11510,#555,.T.);
#14362=EDGE_CURVE('',#11515,#11514,#10487,.T.);
#14363=EDGE_CURVE('',#11515,#11424,#5749,.T.);
#14364=EDGE_CURVE('',#11516,#11515,#5750,.T.);
#14365=EDGE_CURVE('',#11425,#11516,#5751,.T.);
#14366=EDGE_CURVE('',#11426,#11517,#5752,.T.);
#14367=EDGE_CURVE('',#11518,#11517,#10488,.T.);
#14368=EDGE_CURVE('',#11427,#11518,#5753,.T.);
#14369=EDGE_CURVE('',#11519,#11518,#556,.T.);
#14370=EDGE_CURVE('',#11428,#11519,#5754,.T.);
#14371=EDGE_CURVE('',#11429,#11520,#5755,.T.);
#14372=EDGE_CURVE('',#11520,#11519,#5756,.T.);
#14373=EDGE_CURVE('',#11517,#11516,#557,.T.);
#14374=EDGE_CURVE('',#11521,#11520,#10489,.T.);
#14375=EDGE_CURVE('',#11521,#11430,#5757,.T.);
#14376=EDGE_CURVE('',#11522,#11521,#5758,.T.);
#14377=EDGE_CURVE('',#11431,#11522,#5759,.T.);
#14378=EDGE_CURVE('',#11432,#11523,#5760,.T.);
#14379=EDGE_CURVE('',#11524,#11523,#10490,.T.);
#14380=EDGE_CURVE('',#11433,#11524,#5761,.T.);
#14381=EDGE_CURVE('',#11525,#11524,#558,.T.);
#14382=EDGE_CURVE('',#11434,#11525,#5762,.T.);
#14383=EDGE_CURVE('',#11435,#11526,#5763,.T.);
#14384=EDGE_CURVE('',#11526,#11525,#5764,.T.);
#14385=EDGE_CURVE('',#11523,#11522,#559,.T.);
#14386=EDGE_CURVE('',#11527,#11526,#10491,.T.);
#14387=EDGE_CURVE('',#11527,#11436,#5765,.T.);
#14388=EDGE_CURVE('',#11528,#11527,#5766,.T.);
#14389=EDGE_CURVE('',#11437,#11528,#5767,.T.);
#14390=EDGE_CURVE('',#11438,#11529,#5768,.T.);
#14391=EDGE_CURVE('',#11530,#11529,#10492,.T.);
#14392=EDGE_CURVE('',#11439,#11530,#5769,.T.);
#14393=EDGE_CURVE('',#11531,#11530,#560,.T.);
#14394=EDGE_CURVE('',#11440,#11531,#5770,.T.);
#14395=EDGE_CURVE('',#11441,#11532,#5771,.T.);
#14396=EDGE_CURVE('',#11532,#11531,#5772,.T.);
#14397=EDGE_CURVE('',#11529,#11528,#561,.T.);
#14398=EDGE_CURVE('',#11533,#11532,#10493,.T.);
#14399=EDGE_CURVE('',#11533,#11442,#5773,.T.);
#14400=EDGE_CURVE('',#11534,#11533,#5774,.T.);
#14401=EDGE_CURVE('',#11443,#11534,#5775,.T.);
#14402=EDGE_CURVE('',#11444,#11535,#5776,.T.);
#14403=EDGE_CURVE('',#11536,#11535,#10494,.T.);
#14404=EDGE_CURVE('',#11445,#11536,#5777,.T.);
#14405=EDGE_CURVE('',#11537,#11536,#562,.T.);
#14406=EDGE_CURVE('',#11446,#11537,#5778,.T.);
#14407=EDGE_CURVE('',#11447,#11538,#5779,.T.);
#14408=EDGE_CURVE('',#11538,#11537,#5780,.T.);
#14409=EDGE_CURVE('',#11535,#11534,#563,.T.);
#14410=EDGE_CURVE('',#11539,#11538,#10495,.T.);
#14411=EDGE_CURVE('',#11539,#11448,#5781,.T.);
#14412=EDGE_CURVE('',#11540,#11539,#5782,.T.);
#14413=EDGE_CURVE('',#11449,#11540,#5783,.T.);
#14414=EDGE_CURVE('',#11450,#11541,#5784,.T.);
#14415=EDGE_CURVE('',#11542,#11541,#10496,.T.);
#14416=EDGE_CURVE('',#11451,#11542,#5785,.T.);
#14417=EDGE_CURVE('',#11543,#11542,#564,.T.);
#14418=EDGE_CURVE('',#11452,#11543,#5786,.T.);
#14419=EDGE_CURVE('',#11453,#11544,#5787,.T.);
#14420=EDGE_CURVE('',#11544,#11543,#5788,.T.);
#14421=EDGE_CURVE('',#11541,#11540,#565,.T.);
#14422=EDGE_CURVE('',#11545,#11544,#10497,.T.);
#14423=EDGE_CURVE('',#11545,#11454,#5789,.T.);
#14424=EDGE_CURVE('',#11546,#11545,#5790,.T.);
#14425=EDGE_CURVE('',#11455,#11546,#5791,.T.);
#14426=EDGE_CURVE('',#11456,#11547,#5792,.T.);
#14427=EDGE_CURVE('',#11548,#11547,#10498,.T.);
#14428=EDGE_CURVE('',#11457,#11548,#5793,.T.);
#14429=EDGE_CURVE('',#11549,#11548,#566,.T.);
#14430=EDGE_CURVE('',#11458,#11549,#5794,.T.);
#14431=EDGE_CURVE('',#11459,#11550,#5795,.T.);
#14432=EDGE_CURVE('',#11550,#11549,#5796,.T.);
#14433=EDGE_CURVE('',#11547,#11546,#567,.T.);
#14434=EDGE_CURVE('',#11551,#11550,#10499,.T.);
#14435=EDGE_CURVE('',#11551,#11460,#5797,.T.);
#14436=EDGE_CURVE('',#11465,#11552,#5798,.T.);
#14437=EDGE_CURVE('',#11464,#11553,#5799,.T.);
#14438=EDGE_CURVE('',#11552,#11553,#5800,.T.);
#14439=EDGE_CURVE('',#11554,#11551,#5801,.T.);
#14440=EDGE_CURVE('',#11461,#11554,#5802,.T.);
#14441=EDGE_CURVE('',#11462,#11555,#5803,.T.);
#14442=EDGE_CURVE('',#11556,#11555,#10500,.T.);
#14443=EDGE_CURVE('',#11463,#11556,#5804,.T.);
#14444=EDGE_CURVE('',#11553,#11556,#568,.T.);
#14445=EDGE_CURVE('',#11555,#11554,#569,.T.);
#14446=EDGE_CURVE('',#11370,#11557,#10501,.T.);
#14447=EDGE_CURVE('',#11557,#11558,#5805,.T.);
#14448=EDGE_CURVE('',#11558,#11559,#570,.T.);
#14449=EDGE_CURVE('',#11559,#11560,#10502,.T.);
#14450=EDGE_CURVE('',#11560,#11561,#571,.T.);
#14451=EDGE_CURVE('',#11561,#11562,#5806,.T.);
#14452=EDGE_CURVE('',#11562,#11552,#10503,.T.);
#14453=EDGE_CURVE('',#11563,#11563,#10504,.T.);
#14454=EDGE_CURVE('',#11471,#11557,#5807,.T.);
#14455=EDGE_CURVE('',#11470,#11558,#5808,.T.);
#14456=EDGE_CURVE('',#11468,#11560,#5809,.T.);
#14457=EDGE_CURVE('',#11469,#11559,#5810,.T.);
#14458=EDGE_CURVE('',#11562,#11466,#5811,.T.);
#14459=EDGE_CURVE('',#11467,#11561,#5812,.T.);
#14460=EDGE_CURVE('',#11564,#11564,#10505,.T.);
#14461=EDGE_CURVE('',#11565,#11565,#10506,.T.);
#14462=EDGE_CURVE('',#11566,#11566,#10507,.T.);
#14463=EDGE_CURVE('',#11566,#11565,#5813,.T.);
#14464=EDGE_CURVE('',#11567,#11567,#10508,.T.);
#14465=EDGE_CURVE('',#11472,#11567,#5814,.T.);
#14466=EDGE_CURVE('',#11564,#11563,#5815,.T.);
#18618=ORIENTED_EDGE('',*,*,#14170,.F.);
#18619=ORIENTED_EDGE('',*,*,#14171,.F.);
#18620=ORIENTED_EDGE('',*,*,#14172,.F.);
#18621=ORIENTED_EDGE('',*,*,#14173,.T.);
#18622=ORIENTED_EDGE('',*,*,#14174,.F.);
#18623=ORIENTED_EDGE('',*,*,#14175,.T.);
#18624=ORIENTED_EDGE('',*,*,#14176,.F.);
#18625=ORIENTED_EDGE('',*,*,#14177,.F.);
#18626=ORIENTED_EDGE('',*,*,#14178,.T.);
#18627=ORIENTED_EDGE('',*,*,#14177,.T.);
#18628=ORIENTED_EDGE('',*,*,#14179,.F.);
#18629=ORIENTED_EDGE('',*,*,#14180,.F.);
#18630=ORIENTED_EDGE('',*,*,#14181,.F.);
#18631=ORIENTED_EDGE('',*,*,#14182,.T.);
#18632=ORIENTED_EDGE('',*,*,#14180,.T.);
#18633=ORIENTED_EDGE('',*,*,#14183,.F.);
#18634=ORIENTED_EDGE('',*,*,#14184,.F.);
#18635=ORIENTED_EDGE('',*,*,#14172,.T.);
#18636=ORIENTED_EDGE('',*,*,#14185,.F.);
#18637=ORIENTED_EDGE('',*,*,#14175,.F.);
#18638=ORIENTED_EDGE('',*,*,#14186,.F.);
#18639=ORIENTED_EDGE('',*,*,#14187,.F.);
#18640=ORIENTED_EDGE('',*,*,#14188,.T.);
#18641=ORIENTED_EDGE('',*,*,#14189,.T.);
#18642=ORIENTED_EDGE('',*,*,#14190,.F.);
#18643=ORIENTED_EDGE('',*,*,#14191,.F.);
#18644=ORIENTED_EDGE('',*,*,#14192,.F.);
#18645=ORIENTED_EDGE('',*,*,#14193,.F.);
#18646=ORIENTED_EDGE('',*,*,#14194,.T.);
#18647=ORIENTED_EDGE('',*,*,#14195,.T.);
#18648=ORIENTED_EDGE('',*,*,#14196,.F.);
#18649=ORIENTED_EDGE('',*,*,#14197,.F.);
#18650=ORIENTED_EDGE('',*,*,#14198,.F.);
#18651=ORIENTED_EDGE('',*,*,#14199,.F.);
#18652=ORIENTED_EDGE('',*,*,#14200,.T.);
#18653=ORIENTED_EDGE('',*,*,#14201,.T.);
#18654=ORIENTED_EDGE('',*,*,#14202,.F.);
#18655=ORIENTED_EDGE('',*,*,#14203,.F.);
#18656=ORIENTED_EDGE('',*,*,#14204,.F.);
#18657=ORIENTED_EDGE('',*,*,#14205,.F.);
#18658=ORIENTED_EDGE('',*,*,#14206,.T.);
#18659=ORIENTED_EDGE('',*,*,#14207,.T.);
#18660=ORIENTED_EDGE('',*,*,#14208,.F.);
#18661=ORIENTED_EDGE('',*,*,#14209,.F.);
#18662=ORIENTED_EDGE('',*,*,#14210,.F.);
#18663=ORIENTED_EDGE('',*,*,#14211,.F.);
#18664=ORIENTED_EDGE('',*,*,#14212,.T.);
#18665=ORIENTED_EDGE('',*,*,#14213,.T.);
#18666=ORIENTED_EDGE('',*,*,#14214,.F.);
#18667=ORIENTED_EDGE('',*,*,#14215,.F.);
#18668=ORIENTED_EDGE('',*,*,#14216,.F.);
#18669=ORIENTED_EDGE('',*,*,#14217,.F.);
#18670=ORIENTED_EDGE('',*,*,#14218,.T.);
#18671=ORIENTED_EDGE('',*,*,#14219,.T.);
#18672=ORIENTED_EDGE('',*,*,#14220,.F.);
#18673=ORIENTED_EDGE('',*,*,#14221,.F.);
#18674=ORIENTED_EDGE('',*,*,#14222,.F.);
#18675=ORIENTED_EDGE('',*,*,#14223,.F.);
#18676=ORIENTED_EDGE('',*,*,#14224,.T.);
#18677=ORIENTED_EDGE('',*,*,#14225,.T.);
#18678=ORIENTED_EDGE('',*,*,#14226,.F.);
#18679=ORIENTED_EDGE('',*,*,#14227,.F.);
#18680=ORIENTED_EDGE('',*,*,#14228,.F.);
#18681=ORIENTED_EDGE('',*,*,#14229,.F.);
#18682=ORIENTED_EDGE('',*,*,#14230,.T.);
#18683=ORIENTED_EDGE('',*,*,#14231,.T.);
#18684=ORIENTED_EDGE('',*,*,#14232,.F.);
#18685=ORIENTED_EDGE('',*,*,#14233,.F.);
#18686=ORIENTED_EDGE('',*,*,#14234,.F.);
#18687=ORIENTED_EDGE('',*,*,#14235,.F.);
#18688=ORIENTED_EDGE('',*,*,#14236,.T.);
#18689=ORIENTED_EDGE('',*,*,#14237,.T.);
#18690=ORIENTED_EDGE('',*,*,#14238,.F.);
#18691=ORIENTED_EDGE('',*,*,#14239,.F.);
#18692=ORIENTED_EDGE('',*,*,#14240,.F.);
#18693=ORIENTED_EDGE('',*,*,#14241,.F.);
#18694=ORIENTED_EDGE('',*,*,#14242,.T.);
#18695=ORIENTED_EDGE('',*,*,#14243,.T.);
#18696=ORIENTED_EDGE('',*,*,#14244,.F.);
#18697=ORIENTED_EDGE('',*,*,#14245,.F.);
#18698=ORIENTED_EDGE('',*,*,#14246,.F.);
#18699=ORIENTED_EDGE('',*,*,#14247,.F.);
#18700=ORIENTED_EDGE('',*,*,#14248,.T.);
#18701=ORIENTED_EDGE('',*,*,#14249,.T.);
#18702=ORIENTED_EDGE('',*,*,#14250,.F.);
#18703=ORIENTED_EDGE('',*,*,#14251,.F.);
#18704=ORIENTED_EDGE('',*,*,#14252,.F.);
#18705=ORIENTED_EDGE('',*,*,#14253,.F.);
#18706=ORIENTED_EDGE('',*,*,#14254,.T.);
#18707=ORIENTED_EDGE('',*,*,#14255,.T.);
#18708=ORIENTED_EDGE('',*,*,#14256,.F.);
#18709=ORIENTED_EDGE('',*,*,#14257,.F.);
#18710=ORIENTED_EDGE('',*,*,#14258,.F.);
#18711=ORIENTED_EDGE('',*,*,#14259,.F.);
#18712=ORIENTED_EDGE('',*,*,#14260,.T.);
#18713=ORIENTED_EDGE('',*,*,#14261,.T.);
#18714=ORIENTED_EDGE('',*,*,#14262,.F.);
#18715=ORIENTED_EDGE('',*,*,#14263,.F.);
#18716=ORIENTED_EDGE('',*,*,#14264,.F.);
#18717=ORIENTED_EDGE('',*,*,#14265,.F.);
#18718=ORIENTED_EDGE('',*,*,#14266,.T.);
#18719=ORIENTED_EDGE('',*,*,#14267,.T.);
#18720=ORIENTED_EDGE('',*,*,#14268,.F.);
#18721=ORIENTED_EDGE('',*,*,#14269,.F.);
#18722=ORIENTED_EDGE('',*,*,#14270,.F.);
#18723=ORIENTED_EDGE('',*,*,#14271,.F.);
#18724=ORIENTED_EDGE('',*,*,#14272,.T.);
#18725=ORIENTED_EDGE('',*,*,#14273,.T.);
#18726=ORIENTED_EDGE('',*,*,#14274,.F.);
#18727=ORIENTED_EDGE('',*,*,#14275,.F.);
#18728=ORIENTED_EDGE('',*,*,#14276,.F.);
#18729=ORIENTED_EDGE('',*,*,#14173,.F.);
#18730=ORIENTED_EDGE('',*,*,#14184,.T.);
#18731=ORIENTED_EDGE('',*,*,#14174,.T.);
#18732=ORIENTED_EDGE('',*,*,#14178,.F.);
#18733=ORIENTED_EDGE('',*,*,#14182,.F.);
#18734=ORIENTED_EDGE('',*,*,#14277,.T.);
#18735=ORIENTED_EDGE('',*,*,#14181,.T.);
#18736=ORIENTED_EDGE('',*,*,#14278,.F.);
#18737=ORIENTED_EDGE('',*,*,#14279,.T.);
#18738=ORIENTED_EDGE('',*,*,#14186,.T.);
#18739=ORIENTED_EDGE('',*,*,#14279,.F.);
#18740=ORIENTED_EDGE('',*,*,#14280,.F.);
#18741=ORIENTED_EDGE('',*,*,#14281,.F.);
#18742=ORIENTED_EDGE('',*,*,#14187,.T.);
#18743=ORIENTED_EDGE('',*,*,#14189,.F.);
#18744=ORIENTED_EDGE('',*,*,#14282,.T.);
#18745=ORIENTED_EDGE('',*,*,#14283,.F.);
#18746=ORIENTED_EDGE('',*,*,#14284,.F.);
#18747=ORIENTED_EDGE('',*,*,#14190,.T.);
#18748=ORIENTED_EDGE('',*,*,#14284,.T.);
#18749=ORIENTED_EDGE('',*,*,#14285,.F.);
#18750=ORIENTED_EDGE('',*,*,#14286,.F.);
#18751=ORIENTED_EDGE('',*,*,#14287,.F.);
#18752=ORIENTED_EDGE('',*,*,#14191,.T.);
#18753=ORIENTED_EDGE('',*,*,#14286,.T.);
#18754=ORIENTED_EDGE('',*,*,#14288,.F.);
#18755=ORIENTED_EDGE('',*,*,#14188,.F.);
#18756=ORIENTED_EDGE('',*,*,#14281,.T.);
#18757=ORIENTED_EDGE('',*,*,#14289,.F.);
#18758=ORIENTED_EDGE('',*,*,#14282,.F.);
#18759=ORIENTED_EDGE('',*,*,#14287,.T.);
#18760=ORIENTED_EDGE('',*,*,#14290,.F.);
#18761=ORIENTED_EDGE('',*,*,#14291,.T.);
#18762=ORIENTED_EDGE('',*,*,#14192,.T.);
#18763=ORIENTED_EDGE('',*,*,#14291,.F.);
#18764=ORIENTED_EDGE('',*,*,#14292,.F.);
#18765=ORIENTED_EDGE('',*,*,#14293,.F.);
#18766=ORIENTED_EDGE('',*,*,#14193,.T.);
#18767=ORIENTED_EDGE('',*,*,#14195,.F.);
#18768=ORIENTED_EDGE('',*,*,#14294,.T.);
#18769=ORIENTED_EDGE('',*,*,#14295,.F.);
#18770=ORIENTED_EDGE('',*,*,#14296,.F.);
#18771=ORIENTED_EDGE('',*,*,#14196,.T.);
#18772=ORIENTED_EDGE('',*,*,#14296,.T.);
#18773=ORIENTED_EDGE('',*,*,#14297,.F.);
#18774=ORIENTED_EDGE('',*,*,#14298,.F.);
#18775=ORIENTED_EDGE('',*,*,#14299,.F.);
#18776=ORIENTED_EDGE('',*,*,#14197,.T.);
#18777=ORIENTED_EDGE('',*,*,#14298,.T.);
#18778=ORIENTED_EDGE('',*,*,#14300,.F.);
#18779=ORIENTED_EDGE('',*,*,#14194,.F.);
#18780=ORIENTED_EDGE('',*,*,#14293,.T.);
#18781=ORIENTED_EDGE('',*,*,#14301,.F.);
#18782=ORIENTED_EDGE('',*,*,#14294,.F.);
#18783=ORIENTED_EDGE('',*,*,#14299,.T.);
#18784=ORIENTED_EDGE('',*,*,#14302,.F.);
#18785=ORIENTED_EDGE('',*,*,#14303,.T.);
#18786=ORIENTED_EDGE('',*,*,#14198,.T.);
#18787=ORIENTED_EDGE('',*,*,#14303,.F.);
#18788=ORIENTED_EDGE('',*,*,#14304,.F.);
#18789=ORIENTED_EDGE('',*,*,#14305,.F.);
#18790=ORIENTED_EDGE('',*,*,#14199,.T.);
#18791=ORIENTED_EDGE('',*,*,#14201,.F.);
#18792=ORIENTED_EDGE('',*,*,#14306,.T.);
#18793=ORIENTED_EDGE('',*,*,#14307,.F.);
#18794=ORIENTED_EDGE('',*,*,#14308,.F.);
#18795=ORIENTED_EDGE('',*,*,#14202,.T.);
#18796=ORIENTED_EDGE('',*,*,#14308,.T.);
#18797=ORIENTED_EDGE('',*,*,#14309,.F.);
#18798=ORIENTED_EDGE('',*,*,#14310,.F.);
#18799=ORIENTED_EDGE('',*,*,#14311,.F.);
#18800=ORIENTED_EDGE('',*,*,#14203,.T.);
#18801=ORIENTED_EDGE('',*,*,#14310,.T.);
#18802=ORIENTED_EDGE('',*,*,#14312,.F.);
#18803=ORIENTED_EDGE('',*,*,#14200,.F.);
#18804=ORIENTED_EDGE('',*,*,#14305,.T.);
#18805=ORIENTED_EDGE('',*,*,#14313,.F.);
#18806=ORIENTED_EDGE('',*,*,#14306,.F.);
#18807=ORIENTED_EDGE('',*,*,#14311,.T.);
#18808=ORIENTED_EDGE('',*,*,#14314,.F.);
#18809=ORIENTED_EDGE('',*,*,#14315,.T.);
#18810=ORIENTED_EDGE('',*,*,#14204,.T.);
#18811=ORIENTED_EDGE('',*,*,#14315,.F.);
#18812=ORIENTED_EDGE('',*,*,#14316,.F.);
#18813=ORIENTED_EDGE('',*,*,#14317,.F.);
#18814=ORIENTED_EDGE('',*,*,#14205,.T.);
#18815=ORIENTED_EDGE('',*,*,#14207,.F.);
#18816=ORIENTED_EDGE('',*,*,#14318,.T.);
#18817=ORIENTED_EDGE('',*,*,#14319,.F.);
#18818=ORIENTED_EDGE('',*,*,#14320,.F.);
#18819=ORIENTED_EDGE('',*,*,#14208,.T.);
#18820=ORIENTED_EDGE('',*,*,#14320,.T.);
#18821=ORIENTED_EDGE('',*,*,#14321,.F.);
#18822=ORIENTED_EDGE('',*,*,#14322,.F.);
#18823=ORIENTED_EDGE('',*,*,#14323,.F.);
#18824=ORIENTED_EDGE('',*,*,#14209,.T.);
#18825=ORIENTED_EDGE('',*,*,#14322,.T.);
#18826=ORIENTED_EDGE('',*,*,#14324,.F.);
#18827=ORIENTED_EDGE('',*,*,#14206,.F.);
#18828=ORIENTED_EDGE('',*,*,#14317,.T.);
#18829=ORIENTED_EDGE('',*,*,#14325,.F.);
#18830=ORIENTED_EDGE('',*,*,#14318,.F.);
#18831=ORIENTED_EDGE('',*,*,#14323,.T.);
#18832=ORIENTED_EDGE('',*,*,#14326,.F.);
#18833=ORIENTED_EDGE('',*,*,#14327,.T.);
#18834=ORIENTED_EDGE('',*,*,#14210,.T.);
#18835=ORIENTED_EDGE('',*,*,#14327,.F.);
#18836=ORIENTED_EDGE('',*,*,#14328,.F.);
#18837=ORIENTED_EDGE('',*,*,#14329,.F.);
#18838=ORIENTED_EDGE('',*,*,#14211,.T.);
#18839=ORIENTED_EDGE('',*,*,#14213,.F.);
#18840=ORIENTED_EDGE('',*,*,#14330,.T.);
#18841=ORIENTED_EDGE('',*,*,#14331,.F.);
#18842=ORIENTED_EDGE('',*,*,#14332,.F.);
#18843=ORIENTED_EDGE('',*,*,#14214,.T.);
#18844=ORIENTED_EDGE('',*,*,#14332,.T.);
#18845=ORIENTED_EDGE('',*,*,#14333,.F.);
#18846=ORIENTED_EDGE('',*,*,#14334,.F.);
#18847=ORIENTED_EDGE('',*,*,#14335,.F.);
#18848=ORIENTED_EDGE('',*,*,#14215,.T.);
#18849=ORIENTED_EDGE('',*,*,#14334,.T.);
#18850=ORIENTED_EDGE('',*,*,#14336,.F.);
#18851=ORIENTED_EDGE('',*,*,#14212,.F.);
#18852=ORIENTED_EDGE('',*,*,#14329,.T.);
#18853=ORIENTED_EDGE('',*,*,#14337,.F.);
#18854=ORIENTED_EDGE('',*,*,#14330,.F.);
#18855=ORIENTED_EDGE('',*,*,#14335,.T.);
#18856=ORIENTED_EDGE('',*,*,#14338,.F.);
#18857=ORIENTED_EDGE('',*,*,#14339,.T.);
#18858=ORIENTED_EDGE('',*,*,#14216,.T.);
#18859=ORIENTED_EDGE('',*,*,#14339,.F.);
#18860=ORIENTED_EDGE('',*,*,#14340,.F.);
#18861=ORIENTED_EDGE('',*,*,#14341,.F.);
#18862=ORIENTED_EDGE('',*,*,#14217,.T.);
#18863=ORIENTED_EDGE('',*,*,#14219,.F.);
#18864=ORIENTED_EDGE('',*,*,#14342,.T.);
#18865=ORIENTED_EDGE('',*,*,#14343,.F.);
#18866=ORIENTED_EDGE('',*,*,#14344,.F.);
#18867=ORIENTED_EDGE('',*,*,#14220,.T.);
#18868=ORIENTED_EDGE('',*,*,#14344,.T.);
#18869=ORIENTED_EDGE('',*,*,#14345,.F.);
#18870=ORIENTED_EDGE('',*,*,#14346,.F.);
#18871=ORIENTED_EDGE('',*,*,#14347,.F.);
#18872=ORIENTED_EDGE('',*,*,#14221,.T.);
#18873=ORIENTED_EDGE('',*,*,#14346,.T.);
#18874=ORIENTED_EDGE('',*,*,#14348,.F.);
#18875=ORIENTED_EDGE('',*,*,#14218,.F.);
#18876=ORIENTED_EDGE('',*,*,#14341,.T.);
#18877=ORIENTED_EDGE('',*,*,#14349,.F.);
#18878=ORIENTED_EDGE('',*,*,#14342,.F.);
#18879=ORIENTED_EDGE('',*,*,#14347,.T.);
#18880=ORIENTED_EDGE('',*,*,#14350,.F.);
#18881=ORIENTED_EDGE('',*,*,#14351,.T.);
#18882=ORIENTED_EDGE('',*,*,#14222,.T.);
#18883=ORIENTED_EDGE('',*,*,#14351,.F.);
#18884=ORIENTED_EDGE('',*,*,#14352,.F.);
#18885=ORIENTED_EDGE('',*,*,#14353,.F.);
#18886=ORIENTED_EDGE('',*,*,#14223,.T.);
#18887=ORIENTED_EDGE('',*,*,#14225,.F.);
#18888=ORIENTED_EDGE('',*,*,#14354,.T.);
#18889=ORIENTED_EDGE('',*,*,#14355,.F.);
#18890=ORIENTED_EDGE('',*,*,#14356,.F.);
#18891=ORIENTED_EDGE('',*,*,#14226,.T.);
#18892=ORIENTED_EDGE('',*,*,#14356,.T.);
#18893=ORIENTED_EDGE('',*,*,#14357,.F.);
#18894=ORIENTED_EDGE('',*,*,#14358,.F.);
#18895=ORIENTED_EDGE('',*,*,#14359,.F.);
#18896=ORIENTED_EDGE('',*,*,#14227,.T.);
#18897=ORIENTED_EDGE('',*,*,#14358,.T.);
#18898=ORIENTED_EDGE('',*,*,#14360,.F.);
#18899=ORIENTED_EDGE('',*,*,#14224,.F.);
#18900=ORIENTED_EDGE('',*,*,#14353,.T.);
#18901=ORIENTED_EDGE('',*,*,#14361,.F.);
#18902=ORIENTED_EDGE('',*,*,#14354,.F.);
#18903=ORIENTED_EDGE('',*,*,#14359,.T.);
#18904=ORIENTED_EDGE('',*,*,#14362,.F.);
#18905=ORIENTED_EDGE('',*,*,#14363,.T.);
#18906=ORIENTED_EDGE('',*,*,#14228,.T.);
#18907=ORIENTED_EDGE('',*,*,#14363,.F.);
#18908=ORIENTED_EDGE('',*,*,#14364,.F.);
#18909=ORIENTED_EDGE('',*,*,#14365,.F.);
#18910=ORIENTED_EDGE('',*,*,#14229,.T.);
#18911=ORIENTED_EDGE('',*,*,#14231,.F.);
#18912=ORIENTED_EDGE('',*,*,#14366,.T.);
#18913=ORIENTED_EDGE('',*,*,#14367,.F.);
#18914=ORIENTED_EDGE('',*,*,#14368,.F.);
#18915=ORIENTED_EDGE('',*,*,#14232,.T.);
#18916=ORIENTED_EDGE('',*,*,#14368,.T.);
#18917=ORIENTED_EDGE('',*,*,#14369,.F.);
#18918=ORIENTED_EDGE('',*,*,#14370,.F.);
#18919=ORIENTED_EDGE('',*,*,#14371,.F.);
#18920=ORIENTED_EDGE('',*,*,#14233,.T.);
#18921=ORIENTED_EDGE('',*,*,#14370,.T.);
#18922=ORIENTED_EDGE('',*,*,#14372,.F.);
#18923=ORIENTED_EDGE('',*,*,#14230,.F.);
#18924=ORIENTED_EDGE('',*,*,#14365,.T.);
#18925=ORIENTED_EDGE('',*,*,#14373,.F.);
#18926=ORIENTED_EDGE('',*,*,#14366,.F.);
#18927=ORIENTED_EDGE('',*,*,#14371,.T.);
#18928=ORIENTED_EDGE('',*,*,#14374,.F.);
#18929=ORIENTED_EDGE('',*,*,#14375,.T.);
#18930=ORIENTED_EDGE('',*,*,#14234,.T.);
#18931=ORIENTED_EDGE('',*,*,#14375,.F.);
#18932=ORIENTED_EDGE('',*,*,#14376,.F.);
#18933=ORIENTED_EDGE('',*,*,#14377,.F.);
#18934=ORIENTED_EDGE('',*,*,#14235,.T.);
#18935=ORIENTED_EDGE('',*,*,#14237,.F.);
#18936=ORIENTED_EDGE('',*,*,#14378,.T.);
#18937=ORIENTED_EDGE('',*,*,#14379,.F.);
#18938=ORIENTED_EDGE('',*,*,#14380,.F.);
#18939=ORIENTED_EDGE('',*,*,#14238,.T.);
#18940=ORIENTED_EDGE('',*,*,#14380,.T.);
#18941=ORIENTED_EDGE('',*,*,#14381,.F.);
#18942=ORIENTED_EDGE('',*,*,#14382,.F.);
#18943=ORIENTED_EDGE('',*,*,#14383,.F.);
#18944=ORIENTED_EDGE('',*,*,#14239,.T.);
#18945=ORIENTED_EDGE('',*,*,#14382,.T.);
#18946=ORIENTED_EDGE('',*,*,#14384,.F.);
#18947=ORIENTED_EDGE('',*,*,#14236,.F.);
#18948=ORIENTED_EDGE('',*,*,#14377,.T.);
#18949=ORIENTED_EDGE('',*,*,#14385,.F.);
#18950=ORIENTED_EDGE('',*,*,#14378,.F.);
#18951=ORIENTED_EDGE('',*,*,#14383,.T.);
#18952=ORIENTED_EDGE('',*,*,#14386,.F.);
#18953=ORIENTED_EDGE('',*,*,#14387,.T.);
#18954=ORIENTED_EDGE('',*,*,#14240,.T.);
#18955=ORIENTED_EDGE('',*,*,#14387,.F.);
#18956=ORIENTED_EDGE('',*,*,#14388,.F.);
#18957=ORIENTED_EDGE('',*,*,#14389,.F.);
#18958=ORIENTED_EDGE('',*,*,#14241,.T.);
#18959=ORIENTED_EDGE('',*,*,#14243,.F.);
#18960=ORIENTED_EDGE('',*,*,#14390,.T.);
#18961=ORIENTED_EDGE('',*,*,#14391,.F.);
#18962=ORIENTED_EDGE('',*,*,#14392,.F.);
#18963=ORIENTED_EDGE('',*,*,#14244,.T.);
#18964=ORIENTED_EDGE('',*,*,#14392,.T.);
#18965=ORIENTED_EDGE('',*,*,#14393,.F.);
#18966=ORIENTED_EDGE('',*,*,#14394,.F.);
#18967=ORIENTED_EDGE('',*,*,#14395,.F.);
#18968=ORIENTED_EDGE('',*,*,#14245,.T.);
#18969=ORIENTED_EDGE('',*,*,#14394,.T.);
#18970=ORIENTED_EDGE('',*,*,#14396,.F.);
#18971=ORIENTED_EDGE('',*,*,#14242,.F.);
#18972=ORIENTED_EDGE('',*,*,#14389,.T.);
#18973=ORIENTED_EDGE('',*,*,#14397,.F.);
#18974=ORIENTED_EDGE('',*,*,#14390,.F.);
#18975=ORIENTED_EDGE('',*,*,#14395,.T.);
#18976=ORIENTED_EDGE('',*,*,#14398,.F.);
#18977=ORIENTED_EDGE('',*,*,#14399,.T.);
#18978=ORIENTED_EDGE('',*,*,#14246,.T.);
#18979=ORIENTED_EDGE('',*,*,#14399,.F.);
#18980=ORIENTED_EDGE('',*,*,#14400,.F.);
#18981=ORIENTED_EDGE('',*,*,#14401,.F.);
#18982=ORIENTED_EDGE('',*,*,#14247,.T.);
#18983=ORIENTED_EDGE('',*,*,#14249,.F.);
#18984=ORIENTED_EDGE('',*,*,#14402,.T.);
#18985=ORIENTED_EDGE('',*,*,#14403,.F.);
#18986=ORIENTED_EDGE('',*,*,#14404,.F.);
#18987=ORIENTED_EDGE('',*,*,#14250,.T.);
#18988=ORIENTED_EDGE('',*,*,#14404,.T.);
#18989=ORIENTED_EDGE('',*,*,#14405,.F.);
#18990=ORIENTED_EDGE('',*,*,#14406,.F.);
#18991=ORIENTED_EDGE('',*,*,#14407,.F.);
#18992=ORIENTED_EDGE('',*,*,#14251,.T.);
#18993=ORIENTED_EDGE('',*,*,#14406,.T.);
#18994=ORIENTED_EDGE('',*,*,#14408,.F.);
#18995=ORIENTED_EDGE('',*,*,#14248,.F.);
#18996=ORIENTED_EDGE('',*,*,#14401,.T.);
#18997=ORIENTED_EDGE('',*,*,#14409,.F.);
#18998=ORIENTED_EDGE('',*,*,#14402,.F.);
#18999=ORIENTED_EDGE('',*,*,#14407,.T.);
#19000=ORIENTED_EDGE('',*,*,#14410,.F.);
#19001=ORIENTED_EDGE('',*,*,#14411,.T.);
#19002=ORIENTED_EDGE('',*,*,#14252,.T.);
#19003=ORIENTED_EDGE('',*,*,#14411,.F.);
#19004=ORIENTED_EDGE('',*,*,#14412,.F.);
#19005=ORIENTED_EDGE('',*,*,#14413,.F.);
#19006=ORIENTED_EDGE('',*,*,#14253,.T.);
#19007=ORIENTED_EDGE('',*,*,#14255,.F.);
#19008=ORIENTED_EDGE('',*,*,#14414,.T.);
#19009=ORIENTED_EDGE('',*,*,#14415,.F.);
#19010=ORIENTED_EDGE('',*,*,#14416,.F.);
#19011=ORIENTED_EDGE('',*,*,#14256,.T.);
#19012=ORIENTED_EDGE('',*,*,#14416,.T.);
#19013=ORIENTED_EDGE('',*,*,#14417,.F.);
#19014=ORIENTED_EDGE('',*,*,#14418,.F.);
#19015=ORIENTED_EDGE('',*,*,#14419,.F.);
#19016=ORIENTED_EDGE('',*,*,#14257,.T.);
#19017=ORIENTED_EDGE('',*,*,#14418,.T.);
#19018=ORIENTED_EDGE('',*,*,#14420,.F.);
#19019=ORIENTED_EDGE('',*,*,#14254,.F.);
#19020=ORIENTED_EDGE('',*,*,#14413,.T.);
#19021=ORIENTED_EDGE('',*,*,#14421,.F.);
#19022=ORIENTED_EDGE('',*,*,#14414,.F.);
#19023=ORIENTED_EDGE('',*,*,#14419,.T.);
#19024=ORIENTED_EDGE('',*,*,#14422,.F.);
#19025=ORIENTED_EDGE('',*,*,#14423,.T.);
#19026=ORIENTED_EDGE('',*,*,#14258,.T.);
#19027=ORIENTED_EDGE('',*,*,#14423,.F.);
#19028=ORIENTED_EDGE('',*,*,#14424,.F.);
#19029=ORIENTED_EDGE('',*,*,#14425,.F.);
#19030=ORIENTED_EDGE('',*,*,#14259,.T.);
#19031=ORIENTED_EDGE('',*,*,#14261,.F.);
#19032=ORIENTED_EDGE('',*,*,#14426,.T.);
#19033=ORIENTED_EDGE('',*,*,#14427,.F.);
#19034=ORIENTED_EDGE('',*,*,#14428,.F.);
#19035=ORIENTED_EDGE('',*,*,#14262,.T.);
#19036=ORIENTED_EDGE('',*,*,#14428,.T.);
#19037=ORIENTED_EDGE('',*,*,#14429,.F.);
#19038=ORIENTED_EDGE('',*,*,#14430,.F.);
#19039=ORIENTED_EDGE('',*,*,#14431,.F.);
#19040=ORIENTED_EDGE('',*,*,#14263,.T.);
#19041=ORIENTED_EDGE('',*,*,#14430,.T.);
#19042=ORIENTED_EDGE('',*,*,#14432,.F.);
#19043=ORIENTED_EDGE('',*,*,#14260,.F.);
#19044=ORIENTED_EDGE('',*,*,#14425,.T.);
#19045=ORIENTED_EDGE('',*,*,#14433,.F.);
#19046=ORIENTED_EDGE('',*,*,#14426,.F.);
#19047=ORIENTED_EDGE('',*,*,#14431,.T.);
#19048=ORIENTED_EDGE('',*,*,#14434,.F.);
#19049=ORIENTED_EDGE('',*,*,#14435,.T.);
#19050=ORIENTED_EDGE('',*,*,#14264,.T.);
#19051=ORIENTED_EDGE('',*,*,#14436,.F.);
#19052=ORIENTED_EDGE('',*,*,#14269,.T.);
#19053=ORIENTED_EDGE('',*,*,#14437,.T.);
#19054=ORIENTED_EDGE('',*,*,#14438,.F.);
#19055=ORIENTED_EDGE('',*,*,#14435,.F.);
#19056=ORIENTED_EDGE('',*,*,#14439,.F.);
#19057=ORIENTED_EDGE('',*,*,#14440,.F.);
#19058=ORIENTED_EDGE('',*,*,#14265,.T.);
#19059=ORIENTED_EDGE('',*,*,#14267,.F.);
#19060=ORIENTED_EDGE('',*,*,#14441,.T.);
#19061=ORIENTED_EDGE('',*,*,#14442,.F.);
#19062=ORIENTED_EDGE('',*,*,#14443,.F.);
#19063=ORIENTED_EDGE('',*,*,#14268,.T.);
#19064=ORIENTED_EDGE('',*,*,#14443,.T.);
#19065=ORIENTED_EDGE('',*,*,#14444,.F.);
#19066=ORIENTED_EDGE('',*,*,#14437,.F.);
#19067=ORIENTED_EDGE('',*,*,#14266,.F.);
#19068=ORIENTED_EDGE('',*,*,#14440,.T.);
#19069=ORIENTED_EDGE('',*,*,#14445,.F.);
#19070=ORIENTED_EDGE('',*,*,#14441,.F.);
#19071=ORIENTED_EDGE('',*,*,#14446,.T.);
#19072=ORIENTED_EDGE('',*,*,#14447,.T.);
#19073=ORIENTED_EDGE('',*,*,#14448,.T.);
#19074=ORIENTED_EDGE('',*,*,#14449,.T.);
#19075=ORIENTED_EDGE('',*,*,#14450,.T.);
#19076=ORIENTED_EDGE('',*,*,#14451,.T.);
#19077=ORIENTED_EDGE('',*,*,#14452,.T.);
#19078=ORIENTED_EDGE('',*,*,#14438,.T.);
#19079=ORIENTED_EDGE('',*,*,#14444,.T.);
#19080=ORIENTED_EDGE('',*,*,#14442,.T.);
#19081=ORIENTED_EDGE('',*,*,#14445,.T.);
#19082=ORIENTED_EDGE('',*,*,#14439,.T.);
#19083=ORIENTED_EDGE('',*,*,#14434,.T.);
#19084=ORIENTED_EDGE('',*,*,#14432,.T.);
#19085=ORIENTED_EDGE('',*,*,#14429,.T.);
#19086=ORIENTED_EDGE('',*,*,#14427,.T.);
#19087=ORIENTED_EDGE('',*,*,#14433,.T.);
#19088=ORIENTED_EDGE('',*,*,#14424,.T.);
#19089=ORIENTED_EDGE('',*,*,#14422,.T.);
#19090=ORIENTED_EDGE('',*,*,#14420,.T.);
#19091=ORIENTED_EDGE('',*,*,#14417,.T.);
#19092=ORIENTED_EDGE('',*,*,#14415,.T.);
#19093=ORIENTED_EDGE('',*,*,#14421,.T.);
#19094=ORIENTED_EDGE('',*,*,#14412,.T.);
#19095=ORIENTED_EDGE('',*,*,#14410,.T.);
#19096=ORIENTED_EDGE('',*,*,#14408,.T.);
#19097=ORIENTED_EDGE('',*,*,#14405,.T.);
#19098=ORIENTED_EDGE('',*,*,#14403,.T.);
#19099=ORIENTED_EDGE('',*,*,#14409,.T.);
#19100=ORIENTED_EDGE('',*,*,#14400,.T.);
#19101=ORIENTED_EDGE('',*,*,#14398,.T.);
#19102=ORIENTED_EDGE('',*,*,#14396,.T.);
#19103=ORIENTED_EDGE('',*,*,#14393,.T.);
#19104=ORIENTED_EDGE('',*,*,#14391,.T.);
#19105=ORIENTED_EDGE('',*,*,#14397,.T.);
#19106=ORIENTED_EDGE('',*,*,#14388,.T.);
#19107=ORIENTED_EDGE('',*,*,#14386,.T.);
#19108=ORIENTED_EDGE('',*,*,#14384,.T.);
#19109=ORIENTED_EDGE('',*,*,#14381,.T.);
#19110=ORIENTED_EDGE('',*,*,#14379,.T.);
#19111=ORIENTED_EDGE('',*,*,#14385,.T.);
#19112=ORIENTED_EDGE('',*,*,#14376,.T.);
#19113=ORIENTED_EDGE('',*,*,#14374,.T.);
#19114=ORIENTED_EDGE('',*,*,#14372,.T.);
#19115=ORIENTED_EDGE('',*,*,#14369,.T.);
#19116=ORIENTED_EDGE('',*,*,#14367,.T.);
#19117=ORIENTED_EDGE('',*,*,#14373,.T.);
#19118=ORIENTED_EDGE('',*,*,#14364,.T.);
#19119=ORIENTED_EDGE('',*,*,#14362,.T.);
#19120=ORIENTED_EDGE('',*,*,#14360,.T.);
#19121=ORIENTED_EDGE('',*,*,#14357,.T.);
#19122=ORIENTED_EDGE('',*,*,#14355,.T.);
#19123=ORIENTED_EDGE('',*,*,#14361,.T.);
#19124=ORIENTED_EDGE('',*,*,#14352,.T.);
#19125=ORIENTED_EDGE('',*,*,#14350,.T.);
#19126=ORIENTED_EDGE('',*,*,#14348,.T.);
#19127=ORIENTED_EDGE('',*,*,#14345,.T.);
#19128=ORIENTED_EDGE('',*,*,#14343,.T.);
#19129=ORIENTED_EDGE('',*,*,#14349,.T.);
#19130=ORIENTED_EDGE('',*,*,#14340,.T.);
#19131=ORIENTED_EDGE('',*,*,#14338,.T.);
#19132=ORIENTED_EDGE('',*,*,#14336,.T.);
#19133=ORIENTED_EDGE('',*,*,#14333,.T.);
#19134=ORIENTED_EDGE('',*,*,#14331,.T.);
#19135=ORIENTED_EDGE('',*,*,#14337,.T.);
#19136=ORIENTED_EDGE('',*,*,#14328,.T.);
#19137=ORIENTED_EDGE('',*,*,#14326,.T.);
#19138=ORIENTED_EDGE('',*,*,#14324,.T.);
#19139=ORIENTED_EDGE('',*,*,#14321,.T.);
#19140=ORIENTED_EDGE('',*,*,#14319,.T.);
#19141=ORIENTED_EDGE('',*,*,#14325,.T.);
#19142=ORIENTED_EDGE('',*,*,#14316,.T.);
#19143=ORIENTED_EDGE('',*,*,#14314,.T.);
#19144=ORIENTED_EDGE('',*,*,#14312,.T.);
#19145=ORIENTED_EDGE('',*,*,#14309,.T.);
#19146=ORIENTED_EDGE('',*,*,#14307,.T.);
#19147=ORIENTED_EDGE('',*,*,#14313,.T.);
#19148=ORIENTED_EDGE('',*,*,#14304,.T.);
#19149=ORIENTED_EDGE('',*,*,#14302,.T.);
#19150=ORIENTED_EDGE('',*,*,#14300,.T.);
#19151=ORIENTED_EDGE('',*,*,#14297,.T.);
#19152=ORIENTED_EDGE('',*,*,#14295,.T.);
#19153=ORIENTED_EDGE('',*,*,#14301,.T.);
#19154=ORIENTED_EDGE('',*,*,#14292,.T.);
#19155=ORIENTED_EDGE('',*,*,#14290,.T.);
#19156=ORIENTED_EDGE('',*,*,#14288,.T.);
#19157=ORIENTED_EDGE('',*,*,#14285,.T.);
#19158=ORIENTED_EDGE('',*,*,#14283,.T.);
#19159=ORIENTED_EDGE('',*,*,#14289,.T.);
#19160=ORIENTED_EDGE('',*,*,#14280,.T.);
#19161=ORIENTED_EDGE('',*,*,#14278,.T.);
#19162=ORIENTED_EDGE('',*,*,#14183,.T.);
#19163=ORIENTED_EDGE('',*,*,#14179,.T.);
#19164=ORIENTED_EDGE('',*,*,#14176,.T.);
#19165=ORIENTED_EDGE('',*,*,#14185,.T.);
#19166=ORIENTED_EDGE('',*,*,#14171,.T.);
#19167=ORIENTED_EDGE('',*,*,#14453,.F.);
#19168=ORIENTED_EDGE('',*,*,#14170,.T.);
#19169=ORIENTED_EDGE('',*,*,#14276,.T.);
#19170=ORIENTED_EDGE('',*,*,#14454,.T.);
#19171=ORIENTED_EDGE('',*,*,#14446,.F.);
#19172=ORIENTED_EDGE('',*,*,#14454,.F.);
#19173=ORIENTED_EDGE('',*,*,#14275,.T.);
#19174=ORIENTED_EDGE('',*,*,#14455,.T.);
#19175=ORIENTED_EDGE('',*,*,#14447,.F.);
#19176=ORIENTED_EDGE('',*,*,#14273,.F.);
#19177=ORIENTED_EDGE('',*,*,#14456,.T.);
#19178=ORIENTED_EDGE('',*,*,#14449,.F.);
#19179=ORIENTED_EDGE('',*,*,#14457,.F.);
#19180=ORIENTED_EDGE('',*,*,#14274,.T.);
#19181=ORIENTED_EDGE('',*,*,#14457,.T.);
#19182=ORIENTED_EDGE('',*,*,#14448,.F.);
#19183=ORIENTED_EDGE('',*,*,#14455,.F.);
#19184=ORIENTED_EDGE('',*,*,#14458,.F.);
#19185=ORIENTED_EDGE('',*,*,#14451,.F.);
#19186=ORIENTED_EDGE('',*,*,#14459,.F.);
#19187=ORIENTED_EDGE('',*,*,#14271,.T.);
#19188=ORIENTED_EDGE('',*,*,#14272,.F.);
#19189=ORIENTED_EDGE('',*,*,#14459,.T.);
#19190=ORIENTED_EDGE('',*,*,#14450,.F.);
#19191=ORIENTED_EDGE('',*,*,#14456,.F.);
#19192=ORIENTED_EDGE('',*,*,#14436,.T.);
#19193=ORIENTED_EDGE('',*,*,#14452,.F.);
#19194=ORIENTED_EDGE('',*,*,#14458,.T.);
#19195=ORIENTED_EDGE('',*,*,#14270,.T.);
#19196=ORIENTED_EDGE('',*,*,#14460,.T.);
#19197=ORIENTED_EDGE('',*,*,#14461,.F.);
#19198=ORIENTED_EDGE('',*,*,#14462,.F.);
#19199=ORIENTED_EDGE('',*,*,#14463,.T.);
#19200=ORIENTED_EDGE('',*,*,#14461,.T.);
#19201=ORIENTED_EDGE('',*,*,#14463,.F.);
#19202=ORIENTED_EDGE('',*,*,#14464,.F.);
#19203=ORIENTED_EDGE('',*,*,#14462,.T.);
#19204=ORIENTED_EDGE('',*,*,#14277,.F.);
#19205=ORIENTED_EDGE('',*,*,#14465,.T.);
#19206=ORIENTED_EDGE('',*,*,#14464,.T.);
#19207=ORIENTED_EDGE('',*,*,#14465,.F.);
#19208=ORIENTED_EDGE('',*,*,#14460,.F.);
#19209=ORIENTED_EDGE('',*,*,#14466,.T.);
#19210=ORIENTED_EDGE('',*,*,#14453,.T.);
#19211=ORIENTED_EDGE('',*,*,#14466,.F.);
#25761=ADVANCED_FACE('',(#2568),#1248,.T.);
#25762=ADVANCED_FACE('',(#2569),#2193,.T.);
#25763=ADVANCED_FACE('',(#2570),#865,.T.);
#25764=ADVANCED_FACE('',(#2571),#1249,.T.);
#25765=ADVANCED_FACE('',(#2572),#866,.T.);
#25766=ADVANCED_FACE('',(#2573,#1013),#1250,.T.);
#25767=ADVANCED_FACE('',(#2574),#2194,.T.);
#25768=ADVANCED_FACE('',(#2575),#1251,.T.);
#25769=ADVANCED_FACE('',(#2576),#2195,.T.);
#25770=ADVANCED_FACE('',(#2577),#867,.T.);
#25771=ADVANCED_FACE('',(#2578),#1252,.T.);
#25772=ADVANCED_FACE('',(#2579),#868,.T.);
#25773=ADVANCED_FACE('',(#2580),#2196,.T.);
#25774=ADVANCED_FACE('',(#2581),#1253,.T.);
#25775=ADVANCED_FACE('',(#2582),#2197,.T.);
#25776=ADVANCED_FACE('',(#2583),#869,.T.);
#25777=ADVANCED_FACE('',(#2584),#1254,.T.);
#25778=ADVANCED_FACE('',(#2585),#870,.T.);
#25779=ADVANCED_FACE('',(#2586),#2198,.T.);
#25780=ADVANCED_FACE('',(#2587),#1255,.T.);
#25781=ADVANCED_FACE('',(#2588),#2199,.T.);
#25782=ADVANCED_FACE('',(#2589),#871,.T.);
#25783=ADVANCED_FACE('',(#2590),#1256,.T.);
#25784=ADVANCED_FACE('',(#2591),#872,.T.);
#25785=ADVANCED_FACE('',(#2592),#2200,.T.);
#25786=ADVANCED_FACE('',(#2593),#1257,.T.);
#25787=ADVANCED_FACE('',(#2594),#2201,.T.);
#25788=ADVANCED_FACE('',(#2595),#873,.T.);
#25789=ADVANCED_FACE('',(#2596),#1258,.T.);
#25790=ADVANCED_FACE('',(#2597),#874,.T.);
#25791=ADVANCED_FACE('',(#2598),#2202,.T.);
#25792=ADVANCED_FACE('',(#2599),#1259,.T.);
#25793=ADVANCED_FACE('',(#2600),#2203,.T.);
#25794=ADVANCED_FACE('',(#2601),#875,.T.);
#25795=ADVANCED_FACE('',(#2602),#1260,.T.);
#25796=ADVANCED_FACE('',(#2603),#876,.T.);
#25797=ADVANCED_FACE('',(#2604),#2204,.T.);
#25798=ADVANCED_FACE('',(#2605),#1261,.T.);
#25799=ADVANCED_FACE('',(#2606),#2205,.T.);
#25800=ADVANCED_FACE('',(#2607),#877,.T.);
#25801=ADVANCED_FACE('',(#2608),#1262,.T.);
#25802=ADVANCED_FACE('',(#2609),#878,.T.);
#25803=ADVANCED_FACE('',(#2610),#2206,.T.);
#25804=ADVANCED_FACE('',(#2611),#1263,.T.);
#25805=ADVANCED_FACE('',(#2612),#2207,.T.);
#25806=ADVANCED_FACE('',(#2613),#879,.T.);
#25807=ADVANCED_FACE('',(#2614),#1264,.T.);
#25808=ADVANCED_FACE('',(#2615),#880,.T.);
#25809=ADVANCED_FACE('',(#2616),#2208,.T.);
#25810=ADVANCED_FACE('',(#2617),#1265,.T.);
#25811=ADVANCED_FACE('',(#2618),#2209,.T.);
#25812=ADVANCED_FACE('',(#2619),#881,.T.);
#25813=ADVANCED_FACE('',(#2620),#1266,.T.);
#25814=ADVANCED_FACE('',(#2621),#882,.T.);
#25815=ADVANCED_FACE('',(#2622),#2210,.T.);
#25816=ADVANCED_FACE('',(#2623),#1267,.T.);
#25817=ADVANCED_FACE('',(#2624),#2211,.T.);
#25818=ADVANCED_FACE('',(#2625),#883,.T.);
#25819=ADVANCED_FACE('',(#2626),#1268,.T.);
#25820=ADVANCED_FACE('',(#2627),#884,.T.);
#25821=ADVANCED_FACE('',(#2628),#2212,.T.);
#25822=ADVANCED_FACE('',(#2629),#1269,.T.);
#25823=ADVANCED_FACE('',(#2630),#2213,.T.);
#25824=ADVANCED_FACE('',(#2631),#885,.T.);
#25825=ADVANCED_FACE('',(#2632),#1270,.T.);
#25826=ADVANCED_FACE('',(#2633),#886,.T.);
#25827=ADVANCED_FACE('',(#2634),#2214,.T.);
#25828=ADVANCED_FACE('',(#2635),#1271,.T.);
#25829=ADVANCED_FACE('',(#2636),#2215,.T.);
#25830=ADVANCED_FACE('',(#2637),#887,.T.);
#25831=ADVANCED_FACE('',(#2638),#1272,.T.);
#25832=ADVANCED_FACE('',(#2639),#888,.T.);
#25833=ADVANCED_FACE('',(#2640),#2216,.T.);
#25834=ADVANCED_FACE('',(#2641),#1273,.T.);
#25835=ADVANCED_FACE('',(#2642),#2217,.T.);
#25836=ADVANCED_FACE('',(#2643),#889,.T.);
#25837=ADVANCED_FACE('',(#2644),#1274,.T.);
#25838=ADVANCED_FACE('',(#2645),#890,.T.);
#25839=ADVANCED_FACE('',(#2646),#2218,.T.);
#25840=ADVANCED_FACE('',(#2647),#1275,.T.);
#25841=ADVANCED_FACE('',(#2648),#2219,.T.);
#25842=ADVANCED_FACE('',(#2649),#891,.T.);
#25843=ADVANCED_FACE('',(#2650),#1276,.T.);
#25844=ADVANCED_FACE('',(#2651),#892,.T.);
#25845=ADVANCED_FACE('',(#2652),#2220,.T.);
#25846=ADVANCED_FACE('',(#2653),#1277,.T.);
#25847=ADVANCED_FACE('',(#2654),#1278,.T.);
#25848=ADVANCED_FACE('',(#2655),#2221,.T.);
#25849=ADVANCED_FACE('',(#2656),#893,.T.);
#25850=ADVANCED_FACE('',(#2657),#894,.T.);
#25851=ADVANCED_FACE('',(#2658,#1014),#1279,.T.);
#25852=ADVANCED_FACE('',(#2659),#2222,.T.);
#25853=ADVANCED_FACE('',(#2660),#1280,.T.);
#25854=ADVANCED_FACE('',(#2661),#2223,.T.);
#25855=ADVANCED_FACE('',(#2662),#895,.T.);
#25856=ADVANCED_FACE('',(#2663),#1281,.T.);
#25857=ADVANCED_FACE('',(#2664),#896,.T.);
#25858=ADVANCED_FACE('',(#2665),#2224,.T.);
#25859=ADVANCED_FACE('',(#2666,#1015),#1282,.T.);
#25860=ADVANCED_FACE('',(#2667),#2225,.F.);
#25861=ADVANCED_FACE('',(#2668,#1016),#1283,.T.);
#25862=ADVANCED_FACE('',(#2669),#2226,.F.);
#25863=ADVANCED_FACE('',(#2670),#2227,.F.);
#26932=CLOSED_SHELL('',(#25761,#25762,#25763,#25764,#25765,#25766,#25767,
#25768,#25769,#25770,#25771,#25772,#25773,#25774,#25775,#25776,#25777,#25778,
#25779,#25780,#25781,#25782,#25783,#25784,#25785,#25786,#25787,#25788,#25789,
#25790,#25791,#25792,#25793,#25794,#25795,#25796,#25797,#25798,#25799,#25800,
#25801,#25802,#25803,#25804,#25805,#25806,#25807,#25808,#25809,#25810,#25811,
#25812,#25813,#25814,#25815,#25816,#25817,#25818,#25819,#25820,#25821,#25822,
#25823,#25824,#25825,#25826,#25827,#25828,#25829,#25830,#25831,#25832,#25833,
#25834,#25835,#25836,#25837,#25838,#25839,#25840,#25841,#25842,#25843,#25844,
#25845,#25846,#25847,#25848,#25849,#25850,#25851,#25852,#25853,#25854,#25855,
#25856,#25857,#25858,#25859,#25860,#25861,#25862,#25863));
#27453=AXIS2_PLACEMENT_3D('',#37130,#30341,#30342);
#27454=AXIS2_PLACEMENT_3D('',#37131,#30343,#30344);
#27455=AXIS2_PLACEMENT_3D('',#37140,#30349,#30350);
#27456=AXIS2_PLACEMENT_3D('',#37143,#30351,#30352);
#27457=AXIS2_PLACEMENT_3D('',#37147,#30354,#30355);
#27458=AXIS2_PLACEMENT_3D('',#37292,#30358,#30359);
#27459=AXIS2_PLACEMENT_3D('',#37438,#30363,#30364);
#27460=AXIS2_PLACEMENT_3D('',#37440,#30365,#30366);
#27461=AXIS2_PLACEMENT_3D('',#37480,#30368,#30369);
#27462=AXIS2_PLACEMENT_3D('',#37520,#30371,#30372);
#27463=AXIS2_PLACEMENT_3D('',#37560,#30374,#30375);
#27464=AXIS2_PLACEMENT_3D('',#37600,#30377,#30378);
#27465=AXIS2_PLACEMENT_3D('',#37640,#30380,#30381);
#27466=AXIS2_PLACEMENT_3D('',#37680,#30383,#30384);
#27467=AXIS2_PLACEMENT_3D('',#37720,#30386,#30387);
#27468=AXIS2_PLACEMENT_3D('',#37760,#30389,#30390);
#27469=AXIS2_PLACEMENT_3D('',#37800,#30392,#30393);
#27470=AXIS2_PLACEMENT_3D('',#37840,#30395,#30396);
#27471=AXIS2_PLACEMENT_3D('',#37880,#30398,#30399);
#27472=AXIS2_PLACEMENT_3D('',#37920,#30401,#30402);
#27473=AXIS2_PLACEMENT_3D('',#37960,#30404,#30405);
#27474=AXIS2_PLACEMENT_3D('',#38000,#30407,#30408);
#27475=AXIS2_PLACEMENT_3D('',#38040,#30410,#30411);
#27476=AXIS2_PLACEMENT_3D('',#38080,#30413,#30414);
#27477=AXIS2_PLACEMENT_3D('',#38120,#30416,#30417);
#27478=AXIS2_PLACEMENT_3D('',#38160,#30419,#30420);
#27479=AXIS2_PLACEMENT_3D('',#38200,#30422,#30423);
#27480=AXIS2_PLACEMENT_3D('',#38240,#30425,#30426);
#27481=AXIS2_PLACEMENT_3D('',#38280,#30428,#30429);
#27482=AXIS2_PLACEMENT_3D('',#38320,#30431,#30432);
#27483=AXIS2_PLACEMENT_3D('',#38360,#30434,#30435);
#27484=AXIS2_PLACEMENT_3D('',#38400,#30437,#30438);
#27485=AXIS2_PLACEMENT_3D('',#38440,#30440,#30441);
#27486=AXIS2_PLACEMENT_3D('',#38480,#30443,#30444);
#27487=AXIS2_PLACEMENT_3D('',#38520,#30446,#30447);
#27488=AXIS2_PLACEMENT_3D('',#38560,#30449,#30450);
#27489=AXIS2_PLACEMENT_3D('',#38600,#30452,#30453);
#27490=AXIS2_PLACEMENT_3D('',#38639,#30455,#30456);
#27491=AXIS2_PLACEMENT_3D('',#38641,#30457,#30458);
#27492=AXIS2_PLACEMENT_3D('',#38642,#30459,#30460);
#27493=AXIS2_PLACEMENT_3D('',#38644,#30461,#30462);
#27494=AXIS2_PLACEMENT_3D('',#38646,#30464,#30465);
#27495=AXIS2_PLACEMENT_3D('',#38650,#30468,#30469);
#27496=AXIS2_PLACEMENT_3D('',#38654,#30471,#30472);
#27497=AXIS2_PLACEMENT_3D('',#38763,#30475,#30476);
#27498=AXIS2_PLACEMENT_3D('',#38872,#30479,#30480);
#27499=AXIS2_PLACEMENT_3D('',#38874,#30481,#30482);
#27500=AXIS2_PLACEMENT_3D('',#38876,#30484,#30485);
#27501=AXIS2_PLACEMENT_3D('',#38880,#30488,#30489);
#27502=AXIS2_PLACEMENT_3D('',#38884,#30491,#30492);
#27503=AXIS2_PLACEMENT_3D('',#38993,#30495,#30496);
#27504=AXIS2_PLACEMENT_3D('',#39102,#30499,#30500);
#27505=AXIS2_PLACEMENT_3D('',#39104,#30501,#30502);
#27506=AXIS2_PLACEMENT_3D('',#39106,#30504,#30505);
#27507=AXIS2_PLACEMENT_3D('',#39110,#30508,#30509);
#27508=AXIS2_PLACEMENT_3D('',#39114,#30511,#30512);
#27509=AXIS2_PLACEMENT_3D('',#39223,#30515,#30516);
#27510=AXIS2_PLACEMENT_3D('',#39332,#30519,#30520);
#27511=AXIS2_PLACEMENT_3D('',#39334,#30521,#30522);
#27512=AXIS2_PLACEMENT_3D('',#39336,#30524,#30525);
#27513=AXIS2_PLACEMENT_3D('',#39340,#30528,#30529);
#27514=AXIS2_PLACEMENT_3D('',#39344,#30531,#30532);
#27515=AXIS2_PLACEMENT_3D('',#39453,#30535,#30536);
#27516=AXIS2_PLACEMENT_3D('',#39562,#30539,#30540);
#27517=AXIS2_PLACEMENT_3D('',#39564,#30541,#30542);
#27518=AXIS2_PLACEMENT_3D('',#39566,#30544,#30545);
#27519=AXIS2_PLACEMENT_3D('',#39570,#30548,#30549);
#27520=AXIS2_PLACEMENT_3D('',#39574,#30551,#30552);
#27521=AXIS2_PLACEMENT_3D('',#39683,#30555,#30556);
#27522=AXIS2_PLACEMENT_3D('',#39792,#30559,#30560);
#27523=AXIS2_PLACEMENT_3D('',#39794,#30561,#30562);
#27524=AXIS2_PLACEMENT_3D('',#39796,#30564,#30565);
#27525=AXIS2_PLACEMENT_3D('',#39800,#30568,#30569);
#27526=AXIS2_PLACEMENT_3D('',#39804,#30571,#30572);
#27527=AXIS2_PLACEMENT_3D('',#39913,#30575,#30576);
#27528=AXIS2_PLACEMENT_3D('',#40022,#30579,#30580);
#27529=AXIS2_PLACEMENT_3D('',#40024,#30581,#30582);
#27530=AXIS2_PLACEMENT_3D('',#40026,#30584,#30585);
#27531=AXIS2_PLACEMENT_3D('',#40030,#30588,#30589);
#27532=AXIS2_PLACEMENT_3D('',#40034,#30591,#30592);
#27533=AXIS2_PLACEMENT_3D('',#40143,#30595,#30596);
#27534=AXIS2_PLACEMENT_3D('',#40252,#30599,#30600);
#27535=AXIS2_PLACEMENT_3D('',#40254,#30601,#30602);
#27536=AXIS2_PLACEMENT_3D('',#40256,#30604,#30605);
#27537=AXIS2_PLACEMENT_3D('',#40260,#30608,#30609);
#27538=AXIS2_PLACEMENT_3D('',#40264,#30611,#30612);
#27539=AXIS2_PLACEMENT_3D('',#40373,#30615,#30616);
#27540=AXIS2_PLACEMENT_3D('',#40482,#30619,#30620);
#27541=AXIS2_PLACEMENT_3D('',#40484,#30621,#30622);
#27542=AXIS2_PLACEMENT_3D('',#40486,#30624,#30625);
#27543=AXIS2_PLACEMENT_3D('',#40490,#30628,#30629);
#27544=AXIS2_PLACEMENT_3D('',#40494,#30631,#30632);
#27545=AXIS2_PLACEMENT_3D('',#40603,#30635,#30636);
#27546=AXIS2_PLACEMENT_3D('',#40712,#30639,#30640);
#27547=AXIS2_PLACEMENT_3D('',#40714,#30641,#30642);
#27548=AXIS2_PLACEMENT_3D('',#40716,#30644,#30645);
#27549=AXIS2_PLACEMENT_3D('',#40720,#30648,#30649);
#27550=AXIS2_PLACEMENT_3D('',#40724,#30651,#30652);
#27551=AXIS2_PLACEMENT_3D('',#40833,#30655,#30656);
#27552=AXIS2_PLACEMENT_3D('',#40942,#30659,#30660);
#27553=AXIS2_PLACEMENT_3D('',#40944,#30661,#30662);
#27554=AXIS2_PLACEMENT_3D('',#40946,#30664,#30665);
#27555=AXIS2_PLACEMENT_3D('',#40950,#30668,#30669);
#27556=AXIS2_PLACEMENT_3D('',#40954,#30671,#30672);
#27557=AXIS2_PLACEMENT_3D('',#41063,#30675,#30676);
#27558=AXIS2_PLACEMENT_3D('',#41172,#30679,#30680);
#27559=AXIS2_PLACEMENT_3D('',#41174,#30681,#30682);
#27560=AXIS2_PLACEMENT_3D('',#41176,#30684,#30685);
#27561=AXIS2_PLACEMENT_3D('',#41180,#30688,#30689);
#27562=AXIS2_PLACEMENT_3D('',#41184,#30691,#30692);
#27563=AXIS2_PLACEMENT_3D('',#41293,#30695,#30696);
#27564=AXIS2_PLACEMENT_3D('',#41402,#30699,#30700);
#27565=AXIS2_PLACEMENT_3D('',#41404,#30701,#30702);
#27566=AXIS2_PLACEMENT_3D('',#41406,#30704,#30705);
#27567=AXIS2_PLACEMENT_3D('',#41410,#30708,#30709);
#27568=AXIS2_PLACEMENT_3D('',#41414,#30711,#30712);
#27569=AXIS2_PLACEMENT_3D('',#41523,#30715,#30716);
#27570=AXIS2_PLACEMENT_3D('',#41632,#30719,#30720);
#27571=AXIS2_PLACEMENT_3D('',#41634,#30721,#30722);
#27572=AXIS2_PLACEMENT_3D('',#41636,#30724,#30725);
#27573=AXIS2_PLACEMENT_3D('',#41642,#30729,#30730);
#27574=AXIS2_PLACEMENT_3D('',#41646,#30733,#30734);
#27575=AXIS2_PLACEMENT_3D('',#41650,#30736,#30737);
#27576=AXIS2_PLACEMENT_3D('',#41862,#30739,#30740);
#27577=AXIS2_PLACEMENT_3D('',#41864,#30741,#30742);
#27578=AXIS2_PLACEMENT_3D('',#41904,#30744,#30745);
#27579=AXIS2_PLACEMENT_3D('',#41943,#30747,#30748);
#27580=AXIS2_PLACEMENT_3D('',#41945,#30749,#30750);
#27581=AXIS2_PLACEMENT_3D('',#41946,#30751,#30752);
#27582=AXIS2_PLACEMENT_3D('',#41948,#30754,#30755);
#27583=AXIS2_PLACEMENT_3D('',#41950,#30757,#30758);
#27584=AXIS2_PLACEMENT_3D('',#42023,#30761,#30762);
#27585=AXIS2_PLACEMENT_3D('',#42096,#30765,#30766);
#27586=AXIS2_PLACEMENT_3D('',#42097,#30767,#30768);
#27587=AXIS2_PLACEMENT_3D('',#42099,#30769,#30770);
#27588=AXIS2_PLACEMENT_3D('',#42101,#30771,#30772);
#27589=AXIS2_PLACEMENT_3D('',#42102,#30773,#30774);
#27590=AXIS2_PLACEMENT_3D('',#42104,#30775,#30776);
#27591=AXIS2_PLACEMENT_3D('',#42106,#30778,#30779);
#27592=AXIS2_PLACEMENT_3D('',#42108,#30780,#30781);
#27593=AXIS2_PLACEMENT_3D('',#42109,#30782,#30783);
#27594=AXIS2_PLACEMENT_3D('',#42111,#30785,#30786);
#30341=DIRECTION('axis',(0.,0.,1.));
#30342=DIRECTION('refdir',(1.,0.,0.));
#30343=DIRECTION('center_axis',(-0.960505777339176,0.,0.278260043301344));
#30344=DIRECTION('ref_axis',(-0.278260043301344,0.,-0.960505777339176));
#30345=DIRECTION('',(0.,1.,0.));
#30346=DIRECTION('',(-0.278260043301344,0.,-0.960505777339176));
#30347=DIRECTION('',(0.,-1.,0.));
#30348=DIRECTION('',(-0.278260043301344,0.,-0.960505777339176));
#30349=DIRECTION('center_axis',(0.,-1.,0.));
#30350=DIRECTION('ref_axis',(0.350496277439372,0.,0.936564124607142));
#30351=DIRECTION('center_axis',(0.,1.,0.));
#30352=DIRECTION('ref_axis',(0.350496277439372,0.,0.936564124607142));
#30353=DIRECTION('',(0.,-1.,0.));
#30354=DIRECTION('center_axis',(0.,-1.,0.));
#30355=DIRECTION('ref_axis',(0.350496277439372,0.,0.936564124607142));
#30356=DIRECTION('',(0.,-1.,0.));
#30357=DIRECTION('',(0.,-1.,0.));
#30358=DIRECTION('center_axis',(0.875939712077029,0.,-0.482420584973746));
#30359=DIRECTION('ref_axis',(0.482420584973746,0.,0.875939712077029));
#30360=DIRECTION('',(0.,-1.,0.));
#30361=DIRECTION('',(0.482420584973746,0.,0.875939712077029));
#30362=DIRECTION('',(0.482420584973746,0.,0.875939712077029));
#30363=DIRECTION('center_axis',(0.,1.,0.));
#30364=DIRECTION('ref_axis',(0.,0.,1.));
#30365=DIRECTION('center_axis',(0.,-1.,0.));
#30366=DIRECTION('ref_axis',(1.,0.,0.));
#30367=DIRECTION('',(-0.62464840640047,0.,-0.780906120081891));
#30368=DIRECTION('center_axis',(0.,1.,0.));
#30369=DIRECTION('ref_axis',(0.6822239107823,0.,0.731143307127204));
#30370=DIRECTION('',(0.780906120081892,0.,0.624648406400469));
#30371=DIRECTION('center_axis',(0.,-1.,0.));
#30372=DIRECTION('ref_axis',(1.,0.,0.));
#30373=DIRECTION('',(-0.87593971207703,0.,-0.482420584973745));
#30374=DIRECTION('center_axis',(0.,1.,0.));
#30375=DIRECTION('ref_axis',(0.910089138083774,0.,0.414412548967732));
#30376=DIRECTION('',(0.960505777339176,0.,0.278260043301343));
#30377=DIRECTION('center_axis',(0.,-1.,0.));
#30378=DIRECTION('ref_axis',(1.,0.,0.));
#30379=DIRECTION('',(-0.993877137003125,0.,-0.110490888956839));
#30380=DIRECTION('center_axis',(0.,1.,0.));
#30381=DIRECTION('ref_axis',(0.999401544090575,0.,0.0345912368870341));
#30382=DIRECTION('',(0.993877137003124,0.,-0.11049088895684));
#30383=DIRECTION('center_axis',(0.,-1.,0.));
#30384=DIRECTION('ref_axis',(1.,0.,0.));
#30385=DIRECTION('',(-0.960505777339176,0.,0.278260043301344));
#30386=DIRECTION('center_axis',(0.,1.,0.));
#30387=DIRECTION('ref_axis',(0.936564124607142,0.,-0.350496277439372));
#30388=DIRECTION('',(0.875939712077029,0.,-0.482420584973746));
#30389=DIRECTION('center_axis',(0.,-1.,0.));
#30390=DIRECTION('ref_axis',(1.,0.,0.));
#30391=DIRECTION('',(-0.780906120081891,0.,0.62464840640047));
#30392=DIRECTION('center_axis',(0.,1.,0.));
#30393=DIRECTION('ref_axis',(0.731143307127204,0.,-0.6822239107823));
#30394=DIRECTION('',(0.624648406400469,0.,-0.780906120081892));
#30395=DIRECTION('center_axis',(0.,-1.,0.));
#30396=DIRECTION('ref_axis',(1.,0.,0.));
#30397=DIRECTION('',(-0.482420584973745,0.,0.87593971207703));
#30398=DIRECTION('center_axis',(0.,1.,0.));
#30399=DIRECTION('ref_axis',(0.414412548967732,0.,-0.910089138083774));
#30400=DIRECTION('',(0.278260043301343,0.,-0.960505777339176));
#30401=DIRECTION('center_axis',(0.,-1.,0.));
#30402=DIRECTION('ref_axis',(1.,0.,0.));
#30403=DIRECTION('',(-0.110490888956839,0.,0.993877137003125));
#30404=DIRECTION('center_axis',(0.,1.,0.));
#30405=DIRECTION('ref_axis',(0.0345912368870341,0.,-0.999401544090575));
#30406=DIRECTION('',(-0.11049088895684,0.,-0.993877137003124));
#30407=DIRECTION('center_axis',(0.,-1.,0.));
#30408=DIRECTION('ref_axis',(1.,0.,0.));
#30409=DIRECTION('',(0.278260043301344,0.,0.960505777339176));
#30410=DIRECTION('center_axis',(0.,1.,0.));
#30411=DIRECTION('ref_axis',(-0.350496277439372,0.,-0.936564124607142));
#30412=DIRECTION('',(-0.482420584973746,0.,-0.875939712077029));
#30413=DIRECTION('center_axis',(0.,-1.,0.));
#30414=DIRECTION('ref_axis',(1.,0.,0.));
#30415=DIRECTION('',(0.62464840640047,0.,0.780906120081891));
#30416=DIRECTION('center_axis',(0.,1.,0.));
#30417=DIRECTION('ref_axis',(-0.6822239107823,0.,-0.731143307127204));
#30418=DIRECTION('',(-0.780906120081892,0.,-0.62464840640047));
#30419=DIRECTION('center_axis',(0.,-1.,0.));
#30420=DIRECTION('ref_axis',(1.,0.,0.));
#30421=DIRECTION('',(0.87593971207703,0.,0.482420584973745));
#30422=DIRECTION('center_axis',(0.,1.,0.));
#30423=DIRECTION('ref_axis',(-0.910089138083774,0.,-0.414412548967732));
#30424=DIRECTION('',(-0.960505777339176,0.,-0.278260043301343));
#30425=DIRECTION('center_axis',(0.,-1.,0.));
#30426=DIRECTION('ref_axis',(1.,0.,0.));
#30427=DIRECTION('',(0.993877137003125,0.,0.110490888956839));
#30428=DIRECTION('center_axis',(0.,1.,0.));
#30429=DIRECTION('ref_axis',(-0.999401544090575,0.,-0.0345912368870342));
#30430=DIRECTION('',(-0.993877137003124,0.,0.110490888956839));
#30431=DIRECTION('center_axis',(0.,-1.,0.));
#30432=DIRECTION('ref_axis',(1.,0.,0.));
#30433=DIRECTION('',(0.960505777339176,0.,-0.278260043301343));
#30434=DIRECTION('center_axis',(0.,1.,0.));
#30435=DIRECTION('ref_axis',(-0.936564124607143,0.,0.350496277439371));
#30436=DIRECTION('',(-0.875939712077029,0.,0.482420584973746));
#30437=DIRECTION('center_axis',(0.,-1.,0.));
#30438=DIRECTION('ref_axis',(1.,0.,0.));
#30439=DIRECTION('',(0.780906120081891,0.,-0.62464840640047));
#30440=DIRECTION('center_axis',(0.,1.,0.));
#30441=DIRECTION('ref_axis',(-0.731143307127204,0.,0.6822239107823));
#30442=DIRECTION('',(-0.62464840640047,0.,0.780906120081892));
#30443=DIRECTION('center_axis',(0.,-1.,0.));
#30444=DIRECTION('ref_axis',(1.,0.,0.));
#30445=DIRECTION('',(0.482420584973745,0.,-0.87593971207703));
#30446=DIRECTION('center_axis',(0.,1.,0.));
#30447=DIRECTION('ref_axis',(-0.414412548967732,0.,0.910089138083774));
#30448=DIRECTION('',(-0.278260043301343,0.,0.960505777339176));
#30449=DIRECTION('center_axis',(0.,-1.,0.));
#30450=DIRECTION('ref_axis',(1.,0.,0.));
#30451=DIRECTION('',(0.110490888956839,0.,-0.993877137003125));
#30452=DIRECTION('center_axis',(0.,1.,0.));
#30453=DIRECTION('ref_axis',(-0.0345912368870343,0.,0.999401544090575));
#30454=DIRECTION('',(0.110490888956839,0.,0.993877137003124));
#30455=DIRECTION('center_axis',(0.,-1.,0.));
#30456=DIRECTION('ref_axis',(1.,0.,0.));
#30457=DIRECTION('center_axis',(0.,-1.,0.));
#30458=DIRECTION('ref_axis',(1.,0.,0.));
#30459=DIRECTION('center_axis',(0.,-1.,0.));
#30460=DIRECTION('ref_axis',(1.,0.,0.));
#30461=DIRECTION('center_axis',(0.,-1.,0.));
#30462=DIRECTION('ref_axis',(1.,0.,0.));
#30463=DIRECTION('',(0.,1.,0.));
#30464=DIRECTION('center_axis',(-0.780906120081891,0.,0.62464840640047));
#30465=DIRECTION('ref_axis',(-0.62464840640047,0.,-0.780906120081891));
#30466=DIRECTION('',(-0.62464840640047,0.,-0.780906120081891));
#30467=DIRECTION('',(0.,-1.,0.));
#30468=DIRECTION('center_axis',(0.,-1.,0.));
#30469=DIRECTION('ref_axis',(0.6822239107823,0.,0.731143307127204));
#30470=DIRECTION('',(0.,-1.,0.));
#30471=DIRECTION('center_axis',(0.,-1.,0.));
#30472=DIRECTION('ref_axis',(0.6822239107823,0.,0.731143307127204));
#30473=DIRECTION('',(0.,-1.,0.));
#30474=DIRECTION('',(0.,-1.,0.));
#30475=DIRECTION('center_axis',(0.624648406400469,0.,-0.780906120081892));
#30476=DIRECTION('ref_axis',(0.780906120081892,0.,0.624648406400469));
#30477=DIRECTION('',(0.,-1.,0.));
#30478=DIRECTION('',(0.780906120081892,0.,0.624648406400469));
#30479=DIRECTION('center_axis',(0.,-1.,0.));
#30480=DIRECTION('ref_axis',(1.,0.,0.));
#30481=DIRECTION('center_axis',(0.,-1.,0.));
#30482=DIRECTION('ref_axis',(1.,0.,0.));
#30483=DIRECTION('',(0.,1.,0.));
#30484=DIRECTION('center_axis',(-0.482420584973745,0.,0.87593971207703));
#30485=DIRECTION('ref_axis',(-0.87593971207703,0.,-0.482420584973745));
#30486=DIRECTION('',(-0.87593971207703,0.,-0.482420584973745));
#30487=DIRECTION('',(0.,-1.,0.));
#30488=DIRECTION('center_axis',(0.,-1.,0.));
#30489=DIRECTION('ref_axis',(0.910089138083774,0.,0.414412548967732));
#30490=DIRECTION('',(0.,-1.,0.));
#30491=DIRECTION('center_axis',(0.,-1.,0.));
#30492=DIRECTION('ref_axis',(0.910089138083774,0.,0.414412548967732));
#30493=DIRECTION('',(0.,-1.,0.));
#30494=DIRECTION('',(0.,-1.,0.));
#30495=DIRECTION('center_axis',(0.278260043301343,0.,-0.960505777339176));
#30496=DIRECTION('ref_axis',(0.960505777339176,0.,0.278260043301343));
#30497=DIRECTION('',(0.,-1.,0.));
#30498=DIRECTION('',(0.960505777339176,0.,0.278260043301343));
#30499=DIRECTION('center_axis',(0.,-1.,0.));
#30500=DIRECTION('ref_axis',(1.,0.,0.));
#30501=DIRECTION('center_axis',(0.,-1.,0.));
#30502=DIRECTION('ref_axis',(1.,0.,0.));
#30503=DIRECTION('',(0.,1.,0.));
#30504=DIRECTION('center_axis',(-0.110490888956839,0.,0.993877137003125));
#30505=DIRECTION('ref_axis',(-0.993877137003125,0.,-0.110490888956839));
#30506=DIRECTION('',(-0.993877137003125,0.,-0.110490888956839));
#30507=DIRECTION('',(0.,-1.,0.));
#30508=DIRECTION('center_axis',(0.,-1.,0.));
#30509=DIRECTION('ref_axis',(0.999401544090575,0.,0.0345912368870341));
#30510=DIRECTION('',(0.,-1.,0.));
#30511=DIRECTION('center_axis',(0.,-1.,0.));
#30512=DIRECTION('ref_axis',(0.999401544090575,0.,0.0345912368870341));
#30513=DIRECTION('',(0.,-1.,0.));
#30514=DIRECTION('',(0.,-1.,0.));
#30515=DIRECTION('center_axis',(-0.11049088895684,0.,-0.993877137003125));
#30516=DIRECTION('ref_axis',(0.993877137003125,0.,-0.11049088895684));
#30517=DIRECTION('',(0.,-1.,0.));
#30518=DIRECTION('',(0.993877137003124,0.,-0.11049088895684));
#30519=DIRECTION('center_axis',(0.,-1.,0.));
#30520=DIRECTION('ref_axis',(1.,0.,0.));
#30521=DIRECTION('center_axis',(0.,-1.,0.));
#30522=DIRECTION('ref_axis',(1.,0.,0.));
#30523=DIRECTION('',(0.,1.,0.));
#30524=DIRECTION('center_axis',(0.278260043301344,0.,0.960505777339176));
#30525=DIRECTION('ref_axis',(-0.960505777339176,0.,0.278260043301344));
#30526=DIRECTION('',(-0.960505777339176,0.,0.278260043301344));
#30527=DIRECTION('',(0.,-1.,0.));
#30528=DIRECTION('center_axis',(0.,-1.,0.));
#30529=DIRECTION('ref_axis',(0.936564124607142,0.,-0.350496277439372));
#30530=DIRECTION('',(0.,-1.,0.));
#30531=DIRECTION('center_axis',(0.,-1.,0.));
#30532=DIRECTION('ref_axis',(0.936564124607142,0.,-0.350496277439372));
#30533=DIRECTION('',(0.,-1.,0.));
#30534=DIRECTION('',(0.,-1.,0.));
#30535=DIRECTION('center_axis',(-0.482420584973746,0.,-0.875939712077029));
#30536=DIRECTION('ref_axis',(0.875939712077029,0.,-0.482420584973746));
#30537=DIRECTION('',(0.,-1.,0.));
#30538=DIRECTION('',(0.875939712077029,0.,-0.482420584973746));
#30539=DIRECTION('center_axis',(0.,-1.,0.));
#30540=DIRECTION('ref_axis',(1.,0.,0.));
#30541=DIRECTION('center_axis',(0.,-1.,0.));
#30542=DIRECTION('ref_axis',(1.,0.,0.));
#30543=DIRECTION('',(0.,1.,0.));
#30544=DIRECTION('center_axis',(0.62464840640047,0.,0.780906120081891));
#30545=DIRECTION('ref_axis',(-0.780906120081891,0.,0.62464840640047));
#30546=DIRECTION('',(-0.780906120081891,0.,0.62464840640047));
#30547=DIRECTION('',(0.,-1.,0.));
#30548=DIRECTION('center_axis',(0.,-1.,0.));
#30549=DIRECTION('ref_axis',(0.731143307127204,0.,-0.6822239107823));
#30550=DIRECTION('',(0.,-1.,0.));
#30551=DIRECTION('center_axis',(0.,-1.,0.));
#30552=DIRECTION('ref_axis',(0.731143307127204,0.,-0.6822239107823));
#30553=DIRECTION('',(0.,-1.,0.));
#30554=DIRECTION('',(0.,-1.,0.));
#30555=DIRECTION('center_axis',(-0.780906120081892,0.,-0.624648406400469));
#30556=DIRECTION('ref_axis',(0.624648406400469,0.,-0.780906120081892));
#30557=DIRECTION('',(0.,-1.,0.));
#30558=DIRECTION('',(0.624648406400469,0.,-0.780906120081892));
#30559=DIRECTION('center_axis',(0.,-1.,0.));
#30560=DIRECTION('ref_axis',(1.,0.,0.));
#30561=DIRECTION('center_axis',(0.,-1.,0.));
#30562=DIRECTION('ref_axis',(1.,0.,0.));
#30563=DIRECTION('',(0.,1.,0.));
#30564=DIRECTION('center_axis',(0.87593971207703,0.,0.482420584973745));
#30565=DIRECTION('ref_axis',(-0.482420584973745,0.,0.87593971207703));
#30566=DIRECTION('',(-0.482420584973745,0.,0.87593971207703));
#30567=DIRECTION('',(0.,-1.,0.));
#30568=DIRECTION('center_axis',(0.,-1.,0.));
#30569=DIRECTION('ref_axis',(0.414412548967732,0.,-0.910089138083774));
#30570=DIRECTION('',(0.,-1.,0.));
#30571=DIRECTION('center_axis',(0.,-1.,0.));
#30572=DIRECTION('ref_axis',(0.414412548967732,0.,-0.910089138083774));
#30573=DIRECTION('',(0.,-1.,0.));
#30574=DIRECTION('',(0.,-1.,0.));
#30575=DIRECTION('center_axis',(-0.960505777339176,0.,-0.278260043301343));
#30576=DIRECTION('ref_axis',(0.278260043301343,0.,-0.960505777339176));
#30577=DIRECTION('',(0.,-1.,0.));
#30578=DIRECTION('',(0.278260043301343,0.,-0.960505777339176));
#30579=DIRECTION('center_axis',(0.,-1.,0.));
#30580=DIRECTION('ref_axis',(1.,0.,0.));
#30581=DIRECTION('center_axis',(0.,-1.,0.));
#30582=DIRECTION('ref_axis',(1.,0.,0.));
#30583=DIRECTION('',(0.,1.,0.));
#30584=DIRECTION('center_axis',(0.993877137003125,0.,0.110490888956839));
#30585=DIRECTION('ref_axis',(-0.110490888956839,0.,0.993877137003125));
#30586=DIRECTION('',(-0.110490888956839,0.,0.993877137003125));
#30587=DIRECTION('',(0.,-1.,0.));
#30588=DIRECTION('center_axis',(0.,-1.,0.));
#30589=DIRECTION('ref_axis',(0.0345912368870341,0.,-0.999401544090575));
#30590=DIRECTION('',(0.,-1.,0.));
#30591=DIRECTION('center_axis',(0.,-1.,0.));
#30592=DIRECTION('ref_axis',(0.0345912368870341,0.,-0.999401544090575));
#30593=DIRECTION('',(0.,-1.,0.));
#30594=DIRECTION('',(0.,-1.,0.));
#30595=DIRECTION('center_axis',(-0.993877137003125,0.,0.11049088895684));
#30596=DIRECTION('ref_axis',(-0.11049088895684,0.,-0.993877137003125));
#30597=DIRECTION('',(0.,-1.,0.));
#30598=DIRECTION('',(-0.11049088895684,0.,-0.993877137003124));
#30599=DIRECTION('center_axis',(0.,-1.,0.));
#30600=DIRECTION('ref_axis',(1.,0.,0.));
#30601=DIRECTION('center_axis',(0.,-1.,0.));
#30602=DIRECTION('ref_axis',(1.,0.,0.));
#30603=DIRECTION('',(0.,1.,0.));
#30604=DIRECTION('center_axis',(0.960505777339176,0.,-0.278260043301344));
#30605=DIRECTION('ref_axis',(0.278260043301344,0.,0.960505777339176));
#30606=DIRECTION('',(0.278260043301344,0.,0.960505777339176));
#30607=DIRECTION('',(0.,-1.,0.));
#30608=DIRECTION('center_axis',(0.,-1.,0.));
#30609=DIRECTION('ref_axis',(-0.350496277439372,0.,-0.936564124607142));
#30610=DIRECTION('',(0.,-1.,0.));
#30611=DIRECTION('center_axis',(0.,-1.,0.));
#30612=DIRECTION('ref_axis',(-0.350496277439372,0.,-0.936564124607142));
#30613=DIRECTION('',(0.,-1.,0.));
#30614=DIRECTION('',(0.,-1.,0.));
#30615=DIRECTION('center_axis',(-0.875939712077029,0.,0.482420584973746));
#30616=DIRECTION('ref_axis',(-0.482420584973746,0.,-0.875939712077029));
#30617=DIRECTION('',(0.,-1.,0.));
#30618=DIRECTION('',(-0.482420584973746,0.,-0.875939712077029));
#30619=DIRECTION('center_axis',(0.,-1.,0.));
#30620=DIRECTION('ref_axis',(1.,0.,0.));
#30621=DIRECTION('center_axis',(0.,-1.,0.));
#30622=DIRECTION('ref_axis',(1.,0.,0.));
#30623=DIRECTION('',(0.,1.,0.));
#30624=DIRECTION('center_axis',(0.780906120081891,0.,-0.62464840640047));
#30625=DIRECTION('ref_axis',(0.62464840640047,0.,0.780906120081891));
#30626=DIRECTION('',(0.62464840640047,0.,0.780906120081891));
#30627=DIRECTION('',(0.,-1.,0.));
#30628=DIRECTION('center_axis',(0.,-1.,0.));
#30629=DIRECTION('ref_axis',(-0.6822239107823,0.,-0.731143307127204));
#30630=DIRECTION('',(0.,-1.,0.));
#30631=DIRECTION('center_axis',(0.,-1.,0.));
#30632=DIRECTION('ref_axis',(-0.6822239107823,0.,-0.731143307127204));
#30633=DIRECTION('',(0.,-1.,0.));
#30634=DIRECTION('',(0.,-1.,0.));
#30635=DIRECTION('center_axis',(-0.62464840640047,0.,0.780906120081892));
#30636=DIRECTION('ref_axis',(-0.780906120081892,0.,-0.62464840640047));
#30637=DIRECTION('',(0.,-1.,0.));
#30638=DIRECTION('',(-0.780906120081892,0.,-0.62464840640047));
#30639=DIRECTION('center_axis',(0.,-1.,0.));
#30640=DIRECTION('ref_axis',(1.,0.,0.));
#30641=DIRECTION('center_axis',(0.,-1.,0.));
#30642=DIRECTION('ref_axis',(1.,0.,0.));
#30643=DIRECTION('',(0.,1.,0.));
#30644=DIRECTION('center_axis',(0.482420584973745,0.,-0.87593971207703));
#30645=DIRECTION('ref_axis',(0.87593971207703,0.,0.482420584973745));
#30646=DIRECTION('',(0.87593971207703,0.,0.482420584973745));
#30647=DIRECTION('',(0.,-1.,0.));
#30648=DIRECTION('center_axis',(0.,-1.,0.));
#30649=DIRECTION('ref_axis',(-0.910089138083774,0.,-0.414412548967732));
#30650=DIRECTION('',(0.,-1.,0.));
#30651=DIRECTION('center_axis',(0.,-1.,0.));
#30652=DIRECTION('ref_axis',(-0.910089138083774,0.,-0.414412548967732));
#30653=DIRECTION('',(0.,-1.,0.));
#30654=DIRECTION('',(0.,-1.,0.));
#30655=DIRECTION('center_axis',(-0.278260043301343,0.,0.960505777339176));
#30656=DIRECTION('ref_axis',(-0.960505777339176,0.,-0.278260043301343));
#30657=DIRECTION('',(0.,-1.,0.));
#30658=DIRECTION('',(-0.960505777339176,0.,-0.278260043301343));
#30659=DIRECTION('center_axis',(0.,-1.,0.));
#30660=DIRECTION('ref_axis',(1.,0.,0.));
#30661=DIRECTION('center_axis',(0.,-1.,0.));
#30662=DIRECTION('ref_axis',(1.,0.,0.));
#30663=DIRECTION('',(0.,1.,0.));
#30664=DIRECTION('center_axis',(0.110490888956839,0.,-0.993877137003125));
#30665=DIRECTION('ref_axis',(0.993877137003125,0.,0.110490888956839));
#30666=DIRECTION('',(0.993877137003125,0.,0.110490888956839));
#30667=DIRECTION('',(0.,-1.,0.));
#30668=DIRECTION('center_axis',(0.,-1.,0.));
#30669=DIRECTION('ref_axis',(-0.999401544090575,0.,-0.0345912368870342));
#30670=DIRECTION('',(0.,-1.,0.));
#30671=DIRECTION('center_axis',(0.,-1.,0.));
#30672=DIRECTION('ref_axis',(-0.999401544090575,0.,-0.0345912368870342));
#30673=DIRECTION('',(0.,-1.,0.));
#30674=DIRECTION('',(0.,-1.,0.));
#30675=DIRECTION('center_axis',(0.110490888956839,0.,0.993877137003125));
#30676=DIRECTION('ref_axis',(-0.993877137003125,0.,0.110490888956839));
#30677=DIRECTION('',(0.,-1.,0.));
#30678=DIRECTION('',(-0.993877137003124,0.,0.110490888956839));
#30679=DIRECTION('center_axis',(0.,-1.,0.));
#30680=DIRECTION('ref_axis',(1.,0.,0.));
#30681=DIRECTION('center_axis',(0.,-1.,0.));
#30682=DIRECTION('ref_axis',(1.,0.,0.));
#30683=DIRECTION('',(0.,1.,0.));
#30684=DIRECTION('center_axis',(-0.278260043301344,0.,-0.960505777339176));
#30685=DIRECTION('ref_axis',(0.960505777339176,0.,-0.278260043301344));
#30686=DIRECTION('',(0.960505777339176,0.,-0.278260043301343));
#30687=DIRECTION('',(0.,-1.,0.));
#30688=DIRECTION('center_axis',(0.,-1.,0.));
#30689=DIRECTION('ref_axis',(-0.936564124607143,0.,0.350496277439371));
#30690=DIRECTION('',(0.,-1.,0.));
#30691=DIRECTION('center_axis',(0.,-1.,0.));
#30692=DIRECTION('ref_axis',(-0.936564124607143,0.,0.350496277439371));
#30693=DIRECTION('',(0.,-1.,0.));
#30694=DIRECTION('',(0.,-1.,0.));
#30695=DIRECTION('center_axis',(0.482420584973746,0.,0.875939712077029));
#30696=DIRECTION('ref_axis',(-0.875939712077029,0.,0.482420584973746));
#30697=DIRECTION('',(0.,-1.,0.));
#30698=DIRECTION('',(-0.875939712077029,0.,0.482420584973746));
#30699=DIRECTION('center_axis',(0.,-1.,0.));
#30700=DIRECTION('ref_axis',(1.,0.,0.));
#30701=DIRECTION('center_axis',(0.,-1.,0.));
#30702=DIRECTION('ref_axis',(1.,0.,0.));
#30703=DIRECTION('',(0.,1.,0.));
#30704=DIRECTION('center_axis',(-0.62464840640047,0.,-0.780906120081891));
#30705=DIRECTION('ref_axis',(0.780906120081891,0.,-0.62464840640047));
#30706=DIRECTION('',(0.780906120081891,0.,-0.62464840640047));
#30707=DIRECTION('',(0.,-1.,0.));
#30708=DIRECTION('center_axis',(0.,-1.,0.));
#30709=DIRECTION('ref_axis',(-0.731143307127204,0.,0.6822239107823));
#30710=DIRECTION('',(0.,-1.,0.));
#30711=DIRECTION('center_axis',(0.,-1.,0.));
#30712=DIRECTION('ref_axis',(-0.731143307127204,0.,0.6822239107823));
#30713=DIRECTION('',(0.,-1.,0.));
#30714=DIRECTION('',(0.,-1.,0.));
#30715=DIRECTION('center_axis',(0.780906120081892,0.,0.62464840640047));
#30716=DIRECTION('ref_axis',(-0.62464840640047,0.,0.780906120081892));
#30717=DIRECTION('',(0.,-1.,0.));
#30718=DIRECTION('',(-0.62464840640047,0.,0.780906120081892));
#30719=DIRECTION('center_axis',(0.,-1.,0.));
#30720=DIRECTION('ref_axis',(1.,0.,0.));
#30721=DIRECTION('center_axis',(0.,-1.,0.));
#30722=DIRECTION('ref_axis',(1.,0.,0.));
#30723=DIRECTION('',(0.,1.,0.));
#30724=DIRECTION('center_axis',(0.960505777339176,0.,0.278260043301343));
#30725=DIRECTION('ref_axis',(-0.278260043301343,0.,0.960505777339176));
#30726=DIRECTION('',(0.,-1.,0.));
#30727=DIRECTION('',(0.,-1.,0.));
#30728=DIRECTION('',(-0.278260043301343,0.,0.960505777339176));
#30729=DIRECTION('center_axis',(-0.87593971207703,0.,-0.482420584973745));
#30730=DIRECTION('ref_axis',(0.482420584973745,0.,-0.87593971207703));
#30731=DIRECTION('',(0.482420584973745,0.,-0.87593971207703));
#30732=DIRECTION('',(0.,-1.,0.));
#30733=DIRECTION('center_axis',(0.,-1.,0.));
#30734=DIRECTION('ref_axis',(-0.414412548967732,0.,0.910089138083774));
#30735=DIRECTION('',(0.,-1.,0.));
#30736=DIRECTION('center_axis',(0.,-1.,0.));
#30737=DIRECTION('ref_axis',(-0.414412548967732,0.,0.910089138083774));
#30738=DIRECTION('',(0.,-1.,0.));
#30739=DIRECTION('center_axis',(0.,-1.,0.));
#30740=DIRECTION('ref_axis',(0.,0.,-1.));
#30741=DIRECTION('center_axis',(0.,-1.,0.));
#30742=DIRECTION('ref_axis',(1.,0.,0.));
#30743=DIRECTION('',(0.110490888956839,0.,0.993877137003124));
#30744=DIRECTION('center_axis',(0.,-1.,0.));
#30745=DIRECTION('ref_axis',(-0.0345912368870343,0.,0.999401544090575));
#30746=DIRECTION('',(0.110490888956839,0.,-0.993877137003125));
#30747=DIRECTION('center_axis',(0.,-1.,0.));
#30748=DIRECTION('ref_axis',(1.,0.,0.));
#30749=DIRECTION('center_axis',(0.,-1.,0.));
#30750=DIRECTION('ref_axis',(1.,0.,0.));
#30751=DIRECTION('center_axis',(0.,-1.,0.));
#30752=DIRECTION('ref_axis',(1.,0.,0.));
#30753=DIRECTION('',(0.,-1.,0.));
#30754=DIRECTION('center_axis',(0.993877137003125,0.,-0.110490888956839));
#30755=DIRECTION('ref_axis',(0.110490888956839,0.,0.993877137003125));
#30756=DIRECTION('',(0.,-1.,0.));
#30757=DIRECTION('center_axis',(0.,-1.,0.));
#30758=DIRECTION('ref_axis',(-0.0345912368870343,0.,0.999401544090575));
#30759=DIRECTION('',(0.,-1.,0.));
#30760=DIRECTION('',(0.,-1.,0.));
#30761=DIRECTION('center_axis',(-0.993877137003125,0.,-0.110490888956839));
#30762=DIRECTION('ref_axis',(0.110490888956839,0.,-0.993877137003125));
#30763=DIRECTION('',(0.,1.,0.));
#30764=DIRECTION('',(0.,-1.,0.));
#30765=DIRECTION('center_axis',(0.,-1.,0.));
#30766=DIRECTION('ref_axis',(1.,0.,0.));
#30767=DIRECTION('center_axis',(0.,-1.,0.));
#30768=DIRECTION('ref_axis',(0.,0.,-1.));
#30769=DIRECTION('center_axis',(0.,-1.,0.));
#30770=DIRECTION('ref_axis',(1.,0.,0.));
#30771=DIRECTION('center_axis',(0.,-1.,0.));
#30772=DIRECTION('ref_axis',(1.,0.,0.));
#30773=DIRECTION('center_axis',(0.,-1.,0.));
#30774=DIRECTION('ref_axis',(1.,0.,0.));
#30775=DIRECTION('center_axis',(0.,-1.,0.));
#30776=DIRECTION('ref_axis',(1.,0.,0.));
#30777=DIRECTION('',(0.,-1.,0.));
#30778=DIRECTION('center_axis',(0.,1.,0.));
#30779=DIRECTION('ref_axis',(0.,0.,1.));
#30780=DIRECTION('center_axis',(0.,-1.,0.));
#30781=DIRECTION('ref_axis',(1.,0.,0.));
#30782=DIRECTION('center_axis',(0.,-1.,0.));
#30783=DIRECTION('ref_axis',(1.,0.,0.));
#30784=DIRECTION('',(0.,-1.,0.));
#30785=DIRECTION('center_axis',(0.,-1.,0.));
#30786=DIRECTION('ref_axis',(1.,0.,0.));
#30787=DIRECTION('',(0.,-1.,0.));
#37130=CARTESIAN_POINT('',(0.,0.,0.));
#37131=CARTESIAN_POINT('Origin',(1.66039107437149,57.495,5.73138421404289));
#37132=CARTESIAN_POINT('',(1.4909173120086,51.145,5.1463899549833));
#37133=CARTESIAN_POINT('',(1.4909173120086,57.495,5.1463899549833));
#37134=CARTESIAN_POINT('',(1.4909173120086,54.32,5.1463899549833));
#37135=CARTESIAN_POINT('',(1.66039107437149,51.145,5.73138421404289));
#37136=CARTESIAN_POINT('',(1.66039107437149,51.145,5.73138421404289));
#37137=CARTESIAN_POINT('',(1.66039107437149,57.495,5.73138421404289));
#37138=CARTESIAN_POINT('',(1.66039107437149,57.495,5.73138421404289));
#37139=CARTESIAN_POINT('',(1.66039107437149,57.495,5.73138421404289));
#37140=CARTESIAN_POINT('Origin',(6.23660068148934E-13,57.495,1.50456066262064E-12));
#37141=CARTESIAN_POINT('',(2.50394540602693,57.495,6.6908141061934));
#37142=CARTESIAN_POINT('',(2.96056324982543,57.495,6.5016768024705));
#37143=CARTESIAN_POINT('Origin',(6.23660068148934E-13,57.495,1.50456066262064E-12));
#37144=CARTESIAN_POINT('',(2.50394540602693,51.145,6.6908141061934));
#37145=CARTESIAN_POINT('',(2.50394540602693,57.495,6.6908141061934));
#37146=CARTESIAN_POINT('',(2.96056324982543,51.145,6.5016768024705));
#37147=CARTESIAN_POINT('Origin',(6.23660068148934E-13,51.145,1.50456066262064E-12));
#37148=CARTESIAN_POINT('',(2.96056324982543,57.495,6.5016768024705));
#37149=CARTESIAN_POINT('Ctrl Pts',(2.87862685522557,57.495,5.22677443144495));
#37150=CARTESIAN_POINT('Ctrl Pts',(2.87862685522557,49.875,5.22677443144495));
#37151=CARTESIAN_POINT('Ctrl Pts',(2.88043681055508,57.495,5.23024117954544));
#37152=CARTESIAN_POINT('Ctrl Pts',(2.88043681055508,49.875,5.23024117954544));
#37153=CARTESIAN_POINT('Ctrl Pts',(2.88406558980908,57.495,5.2374521593957));
#37154=CARTESIAN_POINT('Ctrl Pts',(2.88406558980908,49.875,5.2374521593957));
#37155=CARTESIAN_POINT('Ctrl Pts',(2.88953536864324,57.495,5.24910109063627));
#37156=CARTESIAN_POINT('Ctrl Pts',(2.88953536864324,49.875,5.24910109063627));
#37157=CARTESIAN_POINT('Ctrl Pts',(2.8968816873652,57.495,5.26630084561717));
#37158=CARTESIAN_POINT('Ctrl Pts',(2.8968816873652,49.875,5.26630084561717));
#37159=CARTESIAN_POINT('Ctrl Pts',(2.90614521320845,57.495,5.29057828960674));
#37160=CARTESIAN_POINT('Ctrl Pts',(2.90614521320845,49.875,5.29057828960674));
#37161=CARTESIAN_POINT('Ctrl Pts',(2.91546314862894,57.495,5.31759510370885));
#37162=CARTESIAN_POINT('Ctrl Pts',(2.91546314862894,49.875,5.31759510370885));
#37163=CARTESIAN_POINT('Ctrl Pts',(2.92478335875772,57.495,5.34725389048201));
#37164=CARTESIAN_POINT('Ctrl Pts',(2.92478335875772,49.875,5.34725389048201));
#37165=CARTESIAN_POINT('Ctrl Pts',(2.93401523982667,57.495,5.37936310952306));
#37166=CARTESIAN_POINT('Ctrl Pts',(2.93401523982667,49.875,5.37936310952306));
#37167=CARTESIAN_POINT('Ctrl Pts',(2.94303247002252,57.495,5.41364129622042));
#37168=CARTESIAN_POINT('Ctrl Pts',(2.94303247002252,49.875,5.41364129622042));
#37169=CARTESIAN_POINT('Ctrl Pts',(2.95169462080126,57.495,5.44977003302479));
#37170=CARTESIAN_POINT('Ctrl Pts',(2.95169462080126,49.875,5.44977003302479));
#37171=CARTESIAN_POINT('Ctrl Pts',(2.95986479289849,57.495,5.48743586913294));
#37172=CARTESIAN_POINT('Ctrl Pts',(2.95986479289849,49.875,5.48743586913294));
#37173=CARTESIAN_POINT('Ctrl Pts',(2.96742703426686,57.495,5.52637191504897));
#37174=CARTESIAN_POINT('Ctrl Pts',(2.96742703426686,49.875,5.52637191504897));
#37175=CARTESIAN_POINT('Ctrl Pts',(2.97430877025614,57.495,5.56641026634754));
#37176=CARTESIAN_POINT('Ctrl Pts',(2.97430877025614,49.875,5.56641026634754));
#37177=CARTESIAN_POINT('Ctrl Pts',(2.98047914221006,57.495,5.60747882861056));
#37178=CARTESIAN_POINT('Ctrl Pts',(2.98047914221006,49.875,5.60747882861056));
#37179=CARTESIAN_POINT('Ctrl Pts',(2.98593308820276,57.495,5.64956501668965));
#37180=CARTESIAN_POINT('Ctrl Pts',(2.98593308820276,49.875,5.64956501668965));
#37181=CARTESIAN_POINT('Ctrl Pts',(2.99067972442542,57.495,5.6926888242775));
#37182=CARTESIAN_POINT('Ctrl Pts',(2.99067972442542,49.875,5.6926888242775));
#37183=CARTESIAN_POINT('Ctrl Pts',(2.99473015701059,57.495,5.73687442119609));
#37184=CARTESIAN_POINT('Ctrl Pts',(2.99473015701059,49.875,5.73687442119609));
#37185=CARTESIAN_POINT('Ctrl Pts',(2.99808342690941,57.495,5.78211642456377));
#37186=CARTESIAN_POINT('Ctrl Pts',(2.99808342690941,49.875,5.78211642456377));
#37187=CARTESIAN_POINT('Ctrl Pts',(3.00072490941926,57.495,5.82837721216371));
#37188=CARTESIAN_POINT('Ctrl Pts',(3.00072490941926,49.875,5.82837721216371));
#37189=CARTESIAN_POINT('Ctrl Pts',(3.00263159433907,57.495,5.87560110342618));
#37190=CARTESIAN_POINT('Ctrl Pts',(3.00263159433907,49.875,5.87560110342618));
#37191=CARTESIAN_POINT('Ctrl Pts',(3.00377540211876,57.495,5.92372322806235));
#37192=CARTESIAN_POINT('Ctrl Pts',(3.00377540211876,49.875,5.92372322806235));
#37193=CARTESIAN_POINT('Ctrl Pts',(3.00412716938112,57.495,5.97267956506957));
#37194=CARTESIAN_POINT('Ctrl Pts',(3.00412716938112,49.875,5.97267956506957));
#37195=CARTESIAN_POINT('Ctrl Pts',(3.0036611362189,57.495,6.02241806591682));
#37196=CARTESIAN_POINT('Ctrl Pts',(3.0036611362189,49.875,6.02241806591682));
#37197=CARTESIAN_POINT('Ctrl Pts',(3.00235671375976,57.495,6.07290162599645));
#37198=CARTESIAN_POINT('Ctrl Pts',(3.00235671375976,49.875,6.07290162599645));
#37199=CARTESIAN_POINT('Ctrl Pts',(3.00019778316116,57.495,6.12410381716763));
#37200=CARTESIAN_POINT('Ctrl Pts',(3.00019778316116,49.875,6.12410381716763));
#37201=CARTESIAN_POINT('Ctrl Pts',(2.99717295692923,57.495,6.17600655789219));
#37202=CARTESIAN_POINT('Ctrl Pts',(2.99717295692923,49.875,6.17600655789219));
#37203=CARTESIAN_POINT('Ctrl Pts',(2.9932755486881,57.495,6.22859706400143));
#37204=CARTESIAN_POINT('Ctrl Pts',(2.9932755486881,49.875,6.22859706400143));
#37205=CARTESIAN_POINT('Ctrl Pts',(2.98850417352762,57.495,6.28186459845025));
#37206=CARTESIAN_POINT('Ctrl Pts',(2.98850417352762,49.875,6.28186459845025));
#37207=CARTESIAN_POINT('Ctrl Pts',(2.98286238364848,57.495,6.33579850967655));
#37208=CARTESIAN_POINT('Ctrl Pts',(2.98286238364848,49.875,6.33579850967655));
#37209=CARTESIAN_POINT('Ctrl Pts',(2.97635619664327,57.495,6.39038953466525));
#37210=CARTESIAN_POINT('Ctrl Pts',(2.97635619664327,49.875,6.39038953466525));
#37211=CARTESIAN_POINT('Ctrl Pts',(2.97046502832938,57.495,6.43458214159119));
#37212=CARTESIAN_POINT('Ctrl Pts',(2.97046502832938,49.875,6.43458214159119));
#37213=CARTESIAN_POINT('Ctrl Pts',(2.96566304810545,57.495,6.4680168144459));
#37214=CARTESIAN_POINT('Ctrl Pts',(2.96566304810545,49.875,6.4680168144459));
#37215=CARTESIAN_POINT('Ctrl Pts',(2.96229154623624,57.495,6.49043534784125));
#37216=CARTESIAN_POINT('Ctrl Pts',(2.96229154623624,49.875,6.49043534784125));
#37217=CARTESIAN_POINT('Ctrl Pts',(2.96056324982543,57.495,6.5016768024705));
#37218=CARTESIAN_POINT('Ctrl Pts',(2.96056324982543,49.875,6.5016768024705));
#37219=CARTESIAN_POINT('',(2.87862685522557,57.495,5.22677443144495));
#37220=CARTESIAN_POINT('Ctrl Pts',(2.87862685522557,57.495,5.22677443144495));
#37221=CARTESIAN_POINT('Ctrl Pts',(2.88043681055508,57.495,5.23024117954544));
#37222=CARTESIAN_POINT('Ctrl Pts',(2.88406558980908,57.495,5.2374521593957));
#37223=CARTESIAN_POINT('Ctrl Pts',(2.88953536864324,57.495,5.24910109063627));
#37224=CARTESIAN_POINT('Ctrl Pts',(2.8968816873652,57.495,5.26630084561717));
#37225=CARTESIAN_POINT('Ctrl Pts',(2.90614521320845,57.495,5.29057828960674));
#37226=CARTESIAN_POINT('Ctrl Pts',(2.91546314862894,57.495,5.31759510370885));
#37227=CARTESIAN_POINT('Ctrl Pts',(2.92478335875772,57.495,5.34725389048201));
#37228=CARTESIAN_POINT('Ctrl Pts',(2.93401523982667,57.495,5.37936310952306));
#37229=CARTESIAN_POINT('Ctrl Pts',(2.94303247002252,57.495,5.41364129622042));
#37230=CARTESIAN_POINT('Ctrl Pts',(2.95169462080126,57.495,5.44977003302479));
#37231=CARTESIAN_POINT('Ctrl Pts',(2.95986479289849,57.495,5.48743586913294));
#37232=CARTESIAN_POINT('Ctrl Pts',(2.96742703426686,57.495,5.52637191504897));
#37233=CARTESIAN_POINT('Ctrl Pts',(2.97430877025614,57.495,5.56641026634754));
#37234=CARTESIAN_POINT('Ctrl Pts',(2.98047914221006,57.495,5.60747882861056));
#37235=CARTESIAN_POINT('Ctrl Pts',(2.98593308820276,57.495,5.64956501668965));
#37236=CARTESIAN_POINT('Ctrl Pts',(2.99067972442542,57.495,5.6926888242775));
#37237=CARTESIAN_POINT('Ctrl Pts',(2.99473015701059,57.495,5.73687442119609));
#37238=CARTESIAN_POINT('Ctrl Pts',(2.99808342690941,57.495,5.78211642456377));
#37239=CARTESIAN_POINT('Ctrl Pts',(3.00072490941926,57.495,5.82837721216371));
#37240=CARTESIAN_POINT('Ctrl Pts',(3.00263159433907,57.495,5.87560110342618));
#37241=CARTESIAN_POINT('Ctrl Pts',(3.00377540211876,57.495,5.92372322806235));
#37242=CARTESIAN_POINT('Ctrl Pts',(3.00412716938112,57.495,5.97267956506957));
#37243=CARTESIAN_POINT('Ctrl Pts',(3.0036611362189,57.495,6.02241806591682));
#37244=CARTESIAN_POINT('Ctrl Pts',(3.00235671375976,57.495,6.07290162599645));
#37245=CARTESIAN_POINT('Ctrl Pts',(3.00019778316116,57.495,6.12410381716763));
#37246=CARTESIAN_POINT('Ctrl Pts',(2.99717295692923,57.495,6.17600655789219));
#37247=CARTESIAN_POINT('Ctrl Pts',(2.9932755486881,57.495,6.22859706400143));
#37248=CARTESIAN_POINT('Ctrl Pts',(2.98850417352762,57.495,6.28186459845025));
#37249=CARTESIAN_POINT('Ctrl Pts',(2.98286238364848,57.495,6.33579850967655));
#37250=CARTESIAN_POINT('Ctrl Pts',(2.97635619664327,57.495,6.39038953466525));
#37251=CARTESIAN_POINT('Ctrl Pts',(2.97046502832938,57.495,6.43458214159119));
#37252=CARTESIAN_POINT('Ctrl Pts',(2.96566304810545,57.495,6.4680168144459));
#37253=CARTESIAN_POINT('Ctrl Pts',(2.96229154623624,57.495,6.49043534784125));
#37254=CARTESIAN_POINT('Ctrl Pts',(2.96056324982543,57.495,6.5016768024705));
#37255=CARTESIAN_POINT('',(2.87862685522557,51.145,5.22677443144495));
#37256=CARTESIAN_POINT('Ctrl Pts',(2.87862685522557,51.145,5.22677443144495));
#37257=CARTESIAN_POINT('Ctrl Pts',(2.88043681055508,51.145,5.23024117954544));
#37258=CARTESIAN_POINT('Ctrl Pts',(2.88406558980908,51.145,5.2374521593957));
#37259=CARTESIAN_POINT('Ctrl Pts',(2.88953536864324,51.145,5.24910109063627));
#37260=CARTESIAN_POINT('Ctrl Pts',(2.8968816873652,51.145,5.26630084561717));
#37261=CARTESIAN_POINT('Ctrl Pts',(2.90614521320845,51.145,5.29057828960674));
#37262=CARTESIAN_POINT('Ctrl Pts',(2.91546314862894,51.145,5.31759510370885));
#37263=CARTESIAN_POINT('Ctrl Pts',(2.92478335875772,51.145,5.34725389048201));
#37264=CARTESIAN_POINT('Ctrl Pts',(2.93401523982667,51.145,5.37936310952306));
#37265=CARTESIAN_POINT('Ctrl Pts',(2.94303247002252,51.145,5.41364129622042));
#37266=CARTESIAN_POINT('Ctrl Pts',(2.95169462080126,51.145,5.44977003302479));
#37267=CARTESIAN_POINT('Ctrl Pts',(2.95986479289849,51.145,5.48743586913294));
#37268=CARTESIAN_POINT('Ctrl Pts',(2.96742703426686,51.145,5.52637191504897));
#37269=CARTESIAN_POINT('Ctrl Pts',(2.97430877025614,51.145,5.56641026634754));
#37270=CARTESIAN_POINT('Ctrl Pts',(2.98047914221006,51.145,5.60747882861056));
#37271=CARTESIAN_POINT('Ctrl Pts',(2.98593308820276,51.145,5.64956501668965));
#37272=CARTESIAN_POINT('Ctrl Pts',(2.99067972442542,51.145,5.6926888242775));
#37273=CARTESIAN_POINT('Ctrl Pts',(2.99473015701059,51.145,5.73687442119609));
#37274=CARTESIAN_POINT('Ctrl Pts',(2.99808342690941,51.145,5.78211642456377));
#37275=CARTESIAN_POINT('Ctrl Pts',(3.00072490941926,51.145,5.82837721216371));
#37276=CARTESIAN_POINT('Ctrl Pts',(3.00263159433907,51.145,5.87560110342618));
#37277=CARTESIAN_POINT('Ctrl Pts',(3.00377540211876,51.145,5.92372322806235));
#37278=CARTESIAN_POINT('Ctrl Pts',(3.00412716938112,51.145,5.97267956506957));
#37279=CARTESIAN_POINT('Ctrl Pts',(3.0036611362189,51.145,6.02241806591682));
#37280=CARTESIAN_POINT('Ctrl Pts',(3.00235671375976,51.145,6.07290162599645));
#37281=CARTESIAN_POINT('Ctrl Pts',(3.00019778316116,51.145,6.12410381716763));
#37282=CARTESIAN_POINT('Ctrl Pts',(2.99717295692923,51.145,6.17600655789219));
#37283=CARTESIAN_POINT('Ctrl Pts',(2.9932755486881,51.145,6.22859706400143));
#37284=CARTESIAN_POINT('Ctrl Pts',(2.98850417352762,51.145,6.28186459845025));
#37285=CARTESIAN_POINT('Ctrl Pts',(2.98286238364848,51.145,6.33579850967655));
#37286=CARTESIAN_POINT('Ctrl Pts',(2.97635619664327,51.145,6.39038953466525));
#37287=CARTESIAN_POINT('Ctrl Pts',(2.97046502832938,51.145,6.43458214159119));
#37288=CARTESIAN_POINT('Ctrl Pts',(2.96566304810545,51.145,6.4680168144459));
#37289=CARTESIAN_POINT('Ctrl Pts',(2.96229154623624,51.145,6.49043534784125));
#37290=CARTESIAN_POINT('Ctrl Pts',(2.96056324982543,51.145,6.5016768024705));
#37291=CARTESIAN_POINT('',(2.87862685522557,57.495,5.22677443144495));
#37292=CARTESIAN_POINT('Origin',(2.51244640654327,57.495,4.56189402049717));
#37293=CARTESIAN_POINT('',(2.58480949428933,57.495,4.69328497730872));
#37294=CARTESIAN_POINT('',(2.58480949428933,51.145,4.69328497730872));
#37295=CARTESIAN_POINT('',(2.58480949428933,54.32,4.69328497730872));
#37296=CARTESIAN_POINT('',(2.51244640654327,57.495,4.56189402049717));
#37297=CARTESIAN_POINT('',(2.51244640654327,51.145,4.56189402049717));
#37298=CARTESIAN_POINT('Ctrl Pts',(2.50394540602693,57.495,6.6908141061934));
#37299=CARTESIAN_POINT('Ctrl Pts',(2.50394540602693,49.875,6.6908141061934));
#37300=CARTESIAN_POINT('Ctrl Pts',(2.49477440711623,57.495,6.6840872875067));
#37301=CARTESIAN_POINT('Ctrl Pts',(2.49477440711623,49.875,6.6840872875067));
#37302=CARTESIAN_POINT('Ctrl Pts',(2.47653809829367,57.495,6.67061900235319));
#37303=CARTESIAN_POINT('Ctrl Pts',(2.47653809829367,49.875,6.67061900235319));
#37304=CARTESIAN_POINT('Ctrl Pts',(2.44950070161195,57.495,6.65037263123044));
#37305=CARTESIAN_POINT('Ctrl Pts',(2.44950070161195,49.875,6.65037263123044));
#37306=CARTESIAN_POINT('Ctrl Pts',(2.41408612451248,57.495,6.62328942425873));
#37307=CARTESIAN_POINT('Ctrl Pts',(2.41408612451248,49.875,6.62328942425873));
#37308=CARTESIAN_POINT('Ctrl Pts',(2.37088387159998,57.495,6.58928830924832));
#37309=CARTESIAN_POINT('Ctrl Pts',(2.37088387159998,49.875,6.58928830924832));
#37310=CARTESIAN_POINT('Ctrl Pts',(2.32875748935431,57.495,6.55514062276576));
#37311=CARTESIAN_POINT('Ctrl Pts',(2.32875748935431,49.875,6.55514062276576));
#37312=CARTESIAN_POINT('Ctrl Pts',(2.28771778279682,57.495,6.52084865967131));
#37313=CARTESIAN_POINT('Ctrl Pts',(2.28771778279682,49.875,6.52084865967131));
#37314=CARTESIAN_POINT('Ctrl Pts',(2.24777479550452,57.495,6.48641743997165));
#37315=CARTESIAN_POINT('Ctrl Pts',(2.24777479550452,49.875,6.48641743997165));
#37316=CARTESIAN_POINT('Ctrl Pts',(2.20893514043546,57.495,6.45185553518355));
#37317=CARTESIAN_POINT('Ctrl Pts',(2.20893514043546,49.875,6.45185553518355));
#37318=CARTESIAN_POINT('Ctrl Pts',(2.17120312938033,57.495,6.41717671306116));
#37319=CARTESIAN_POINT('Ctrl Pts',(2.17120312938033,49.875,6.41717671306116));
#37320=CARTESIAN_POINT('Ctrl Pts',(2.13458349574322,57.495,6.38240181135686));
#37321=CARTESIAN_POINT('Ctrl Pts',(2.13458349574322,49.875,6.38240181135686));
#37322=CARTESIAN_POINT('Ctrl Pts',(2.09908352929886,57.495,6.34756091533109));
#37323=CARTESIAN_POINT('Ctrl Pts',(2.09908352929886,49.875,6.34756091533109));
#37324=CARTESIAN_POINT('Ctrl Pts',(2.06471490843566,57.495,6.31269482043472));
#37325=CARTESIAN_POINT('Ctrl Pts',(2.06471490843566,49.875,6.31269482043472));
#37326=CARTESIAN_POINT('Ctrl Pts',(2.03149622201774,57.495,6.27785854554207));
#37327=CARTESIAN_POINT('Ctrl Pts',(2.03149622201774,49.875,6.27785854554207));
#37328=CARTESIAN_POINT('Ctrl Pts',(1.99945211810842,57.495,6.24311798195999));
#37329=CARTESIAN_POINT('Ctrl Pts',(1.99945211810842,49.875,6.24311798195999));
#37330=CARTESIAN_POINT('Ctrl Pts',(1.96860861168855,57.495,6.20853885514991));
#37331=CARTESIAN_POINT('Ctrl Pts',(1.96860861168855,49.875,6.20853885514991));
#37332=CARTESIAN_POINT('Ctrl Pts',(1.93898880419739,57.495,6.17417680788948));
#37333=CARTESIAN_POINT('Ctrl Pts',(1.93898880419739,49.875,6.17417680788948));
#37334=CARTESIAN_POINT('Ctrl Pts',(1.91060895733316,57.495,6.14006878432979));
#37335=CARTESIAN_POINT('Ctrl Pts',(1.91060895733316,49.875,6.14006878432979));
#37336=CARTESIAN_POINT('Ctrl Pts',(1.88347219921808,57.495,6.10621926889293));
#37337=CARTESIAN_POINT('Ctrl Pts',(1.88347219921808,49.875,6.10621926889293));
#37338=CARTESIAN_POINT('Ctrl Pts',(1.85756929242873,57.495,6.07260331771223));
#37339=CARTESIAN_POINT('Ctrl Pts',(1.85756929242873,49.875,6.07260331771223));
#37340=CARTESIAN_POINT('Ctrl Pts',(1.83289254541003,57.495,6.03920034699142));
#37341=CARTESIAN_POINT('Ctrl Pts',(1.83289254541003,49.875,6.03920034699142));
#37342=CARTESIAN_POINT('Ctrl Pts',(1.80944727788364,57.495,6.00602283509636));
#37343=CARTESIAN_POINT('Ctrl Pts',(1.80944727788364,49.875,6.00602283509636));
#37344=CARTESIAN_POINT('Ctrl Pts',(1.78726264793637,57.495,5.97314358084405));
#37345=CARTESIAN_POINT('Ctrl Pts',(1.78726264793637,49.875,5.97314358084405));
#37346=CARTESIAN_POINT('Ctrl Pts',(1.76640606389863,57.495,5.94073262861954));
#37347=CARTESIAN_POINT('Ctrl Pts',(1.76640606389863,49.875,5.94073262861954));
#37348=CARTESIAN_POINT('Ctrl Pts',(1.74698425466385,57.495,5.90906068827417));
#37349=CARTESIAN_POINT('Ctrl Pts',(1.74698425466385,49.875,5.90906068827417));
#37350=CARTESIAN_POINT('Ctrl Pts',(1.72912206102238,57.495,5.87844620539466));
#37351=CARTESIAN_POINT('Ctrl Pts',(1.72912206102238,49.875,5.87844620539466));
#37352=CARTESIAN_POINT('Ctrl Pts',(1.71294534020682,57.495,5.84921363316514));
#37353=CARTESIAN_POINT('Ctrl Pts',(1.71294534020682,49.875,5.84921363316514));
#37354=CARTESIAN_POINT('Ctrl Pts',(1.69856379474193,57.495,5.8216513201319));
#37355=CARTESIAN_POINT('Ctrl Pts',(1.69856379474193,49.875,5.8216513201319));
#37356=CARTESIAN_POINT('Ctrl Pts',(1.68604879760681,57.495,5.79595877235173));
#37357=CARTESIAN_POINT('Ctrl Pts',(1.68604879760681,49.875,5.79595877235173));
#37358=CARTESIAN_POINT('Ctrl Pts',(1.67543235427339,57.495,5.77224172513534));
#37359=CARTESIAN_POINT('Ctrl Pts',(1.67543235427339,49.875,5.77224172513534));
#37360=CARTESIAN_POINT('Ctrl Pts',(1.6684649226767,57.495,5.75488502996854));
#37361=CARTESIAN_POINT('Ctrl Pts',(1.6684649226767,49.875,5.75488502996854));
#37362=CARTESIAN_POINT('Ctrl Pts',(1.66409560210811,57.495,5.74278027398956));
#37363=CARTESIAN_POINT('Ctrl Pts',(1.66409560210811,49.875,5.74278027398956));
#37364=CARTESIAN_POINT('Ctrl Pts',(1.66156260377489,57.495,5.73511540682054));
#37365=CARTESIAN_POINT('Ctrl Pts',(1.66156260377489,49.875,5.73511540682054));
#37366=CARTESIAN_POINT('Ctrl Pts',(1.66039107437149,57.495,5.73138421404289));
#37367=CARTESIAN_POINT('Ctrl Pts',(1.66039107437149,49.875,5.73138421404289));
#37368=CARTESIAN_POINT('Ctrl Pts',(1.66039107437149,57.495,5.73138421404289));
#37369=CARTESIAN_POINT('Ctrl Pts',(1.66156260377489,57.495,5.73511540682054));
#37370=CARTESIAN_POINT('Ctrl Pts',(1.66409560210811,57.495,5.74278027398956));
#37371=CARTESIAN_POINT('Ctrl Pts',(1.6684649226767,57.495,5.75488502996854));
#37372=CARTESIAN_POINT('Ctrl Pts',(1.67543235427339,57.495,5.77224172513534));
#37373=CARTESIAN_POINT('Ctrl Pts',(1.68604879760681,57.495,5.79595877235173));
#37374=CARTESIAN_POINT('Ctrl Pts',(1.69856379474193,57.495,5.8216513201319));
#37375=CARTESIAN_POINT('Ctrl Pts',(1.71294534020682,57.495,5.84921363316514));
#37376=CARTESIAN_POINT('Ctrl Pts',(1.72912206102238,57.495,5.87844620539466));
#37377=CARTESIAN_POINT('Ctrl Pts',(1.74698425466385,57.495,5.90906068827417));
#37378=CARTESIAN_POINT('Ctrl Pts',(1.76640606389863,57.495,5.94073262861954));
#37379=CARTESIAN_POINT('Ctrl Pts',(1.78726264793637,57.495,5.97314358084405));
#37380=CARTESIAN_POINT('Ctrl Pts',(1.80944727788364,57.495,6.00602283509636));
#37381=CARTESIAN_POINT('Ctrl Pts',(1.83289254541003,57.495,6.03920034699142));
#37382=CARTESIAN_POINT('Ctrl Pts',(1.85756929242873,57.495,6.07260331771223));
#37383=CARTESIAN_POINT('Ctrl Pts',(1.88347219921808,57.495,6.10621926889293));
#37384=CARTESIAN_POINT('Ctrl Pts',(1.91060895733316,57.495,6.14006878432979));
#37385=CARTESIAN_POINT('Ctrl Pts',(1.93898880419739,57.495,6.17417680788948));
#37386=CARTESIAN_POINT('Ctrl Pts',(1.96860861168855,57.495,6.20853885514991));
#37387=CARTESIAN_POINT('Ctrl Pts',(1.99945211810842,57.495,6.24311798195999));
#37388=CARTESIAN_POINT('Ctrl Pts',(2.03149622201774,57.495,6.27785854554207));
#37389=CARTESIAN_POINT('Ctrl Pts',(2.06471490843566,57.495,6.31269482043472));
#37390=CARTESIAN_POINT('Ctrl Pts',(2.09908352929886,57.495,6.34756091533109));
#37391=CARTESIAN_POINT('Ctrl Pts',(2.13458349574322,57.495,6.38240181135686));
#37392=CARTESIAN_POINT('Ctrl Pts',(2.17120312938033,57.495,6.41717671306116));
#37393=CARTESIAN_POINT('Ctrl Pts',(2.20893514043546,57.495,6.45185553518355));
#37394=CARTESIAN_POINT('Ctrl Pts',(2.24777479550452,57.495,6.48641743997165));
#37395=CARTESIAN_POINT('Ctrl Pts',(2.28771778279682,57.495,6.52084865967131));
#37396=CARTESIAN_POINT('Ctrl Pts',(2.32875748935431,57.495,6.55514062276576));
#37397=CARTESIAN_POINT('Ctrl Pts',(2.37088387159998,57.495,6.58928830924832));
#37398=CARTESIAN_POINT('Ctrl Pts',(2.41408612451248,57.495,6.62328942425873));
#37399=CARTESIAN_POINT('Ctrl Pts',(2.44950070161195,57.495,6.65037263123044));
#37400=CARTESIAN_POINT('Ctrl Pts',(2.47653809829367,57.495,6.67061900235319));
#37401=CARTESIAN_POINT('Ctrl Pts',(2.49477440711623,57.495,6.6840872875067));
#37402=CARTESIAN_POINT('Ctrl Pts',(2.50394540602693,57.495,6.6908141061934));
#37403=CARTESIAN_POINT('Ctrl Pts',(2.50394540602693,51.145,6.6908141061934));
#37404=CARTESIAN_POINT('Ctrl Pts',(2.49477440711623,51.145,6.6840872875067));
#37405=CARTESIAN_POINT('Ctrl Pts',(2.47653809829367,51.145,6.67061900235319));
#37406=CARTESIAN_POINT('Ctrl Pts',(2.44950070161195,51.145,6.65037263123044));
#37407=CARTESIAN_POINT('Ctrl Pts',(2.41408612451248,51.145,6.62328942425873));
#37408=CARTESIAN_POINT('Ctrl Pts',(2.37088387159998,51.145,6.58928830924832));
#37409=CARTESIAN_POINT('Ctrl Pts',(2.32875748935431,51.145,6.55514062276576));
#37410=CARTESIAN_POINT('Ctrl Pts',(2.28771778279682,51.145,6.52084865967131));
#37411=CARTESIAN_POINT('Ctrl Pts',(2.24777479550452,51.145,6.48641743997165));
#37412=CARTESIAN_POINT('Ctrl Pts',(2.20893514043546,51.145,6.45185553518355));
#37413=CARTESIAN_POINT('Ctrl Pts',(2.17120312938033,51.145,6.41717671306116));
#37414=CARTESIAN_POINT('Ctrl Pts',(2.13458349574322,51.145,6.38240181135686));
#37415=CARTESIAN_POINT('Ctrl Pts',(2.09908352929886,51.145,6.34756091533109));
#37416=CARTESIAN_POINT('Ctrl Pts',(2.06471490843566,51.145,6.31269482043472));
#37417=CARTESIAN_POINT('Ctrl Pts',(2.03149622201774,51.145,6.27785854554207));
#37418=CARTESIAN_POINT('Ctrl Pts',(1.99945211810842,51.145,6.24311798195999));
#37419=CARTESIAN_POINT('Ctrl Pts',(1.96860861168855,51.145,6.20853885514991));
#37420=CARTESIAN_POINT('Ctrl Pts',(1.93898880419739,51.145,6.17417680788948));
#37421=CARTESIAN_POINT('Ctrl Pts',(1.91060895733316,51.145,6.14006878432979));
#37422=CARTESIAN_POINT('Ctrl Pts',(1.88347219921808,51.145,6.10621926889293));
#37423=CARTESIAN_POINT('Ctrl Pts',(1.85756929242873,51.145,6.07260331771223));
#37424=CARTESIAN_POINT('Ctrl Pts',(1.83289254541003,51.145,6.03920034699142));
#37425=CARTESIAN_POINT('Ctrl Pts',(1.80944727788364,51.145,6.00602283509636));
#37426=CARTESIAN_POINT('Ctrl Pts',(1.78726264793637,51.145,5.97314358084405));
#37427=CARTESIAN_POINT('Ctrl Pts',(1.76640606389863,51.145,5.94073262861954));
#37428=CARTESIAN_POINT('Ctrl Pts',(1.74698425466385,51.145,5.90906068827417));
#37429=CARTESIAN_POINT('Ctrl Pts',(1.72912206102238,51.145,5.87844620539466));
#37430=CARTESIAN_POINT('Ctrl Pts',(1.71294534020682,51.145,5.84921363316514));
#37431=CARTESIAN_POINT('Ctrl Pts',(1.69856379474193,51.145,5.8216513201319));
#37432=CARTESIAN_POINT('Ctrl Pts',(1.68604879760681,51.145,5.79595877235173));
#37433=CARTESIAN_POINT('Ctrl Pts',(1.67543235427339,51.145,5.77224172513534));
#37434=CARTESIAN_POINT('Ctrl Pts',(1.6684649226767,51.145,5.75488502996854));
#37435=CARTESIAN_POINT('Ctrl Pts',(1.66409560210811,51.145,5.74278027398956));
#37436=CARTESIAN_POINT('Ctrl Pts',(1.66156260377489,51.145,5.73511540682054));
#37437=CARTESIAN_POINT('Ctrl Pts',(1.66039107437149,51.145,5.73138421404289));
#37438=CARTESIAN_POINT('Origin',(5.358,57.495,0.));
#37439=CARTESIAN_POINT('',(3.34686616149372,57.495,4.18409499139877));
#37440=CARTESIAN_POINT('Origin',(0.,57.495,0.));
#37441=CARTESIAN_POINT('',(3.72730711280926,57.495,4.65970441290367));
#37442=CARTESIAN_POINT('',(3.72730711280926,57.495,4.65970441290367));
#37443=CARTESIAN_POINT('',(4.87380761862879,57.495,5.22328778611671));
#37444=CARTESIAN_POINT('Ctrl Pts',(3.72730711280926,57.495,4.65970441290367));
#37445=CARTESIAN_POINT('Ctrl Pts',(3.72981733050578,57.495,4.66270326064959));
#37446=CARTESIAN_POINT('Ctrl Pts',(3.73509073349858,57.495,4.66881533805013));
#37447=CARTESIAN_POINT('Ctrl Pts',(3.74375974890886,57.495,4.67832660775287));
#37448=CARTESIAN_POINT('Ctrl Pts',(3.75683893603616,57.495,4.69169578253132));
#37449=CARTESIAN_POINT('Ctrl Pts',(3.77572337177431,57.495,4.7095447400518));
#37450=CARTESIAN_POINT('Ctrl Pts',(3.7971178338476,57.495,4.72849227702426));
#37451=CARTESIAN_POINT('Ctrl Pts',(3.82095228990397,57.495,4.74845295472312));
#37452=CARTESIAN_POINT('Ctrl Pts',(3.84708445224627,57.495,4.76926976684252));
#37453=CARTESIAN_POINT('Ctrl Pts',(3.8753026227458,57.495,4.79071829540103));
#37454=CARTESIAN_POINT('Ctrl Pts',(3.90536636162318,57.495,4.81254694822034));
#37455=CARTESIAN_POINT('Ctrl Pts',(3.93703846717724,57.495,4.83450929444279));
#37456=CARTESIAN_POINT('Ctrl Pts',(3.97011673859274,57.495,4.85639607415676));
#37457=CARTESIAN_POINT('Ctrl Pts',(4.00447382552396,57.495,4.87807598288654));
#37458=CARTESIAN_POINT('Ctrl Pts',(4.04005493051012,57.495,4.89949292161185));
#37459=CARTESIAN_POINT('Ctrl Pts',(4.07685036350539,57.495,4.92063739759521));
#37460=CARTESIAN_POINT('Ctrl Pts',(4.11487510765791,57.495,4.94152548435402));
#37461=CARTESIAN_POINT('Ctrl Pts',(4.15414724283858,57.495,4.96217669200723));
#37462=CARTESIAN_POINT('Ctrl Pts',(4.1946621629253,57.495,4.98258807456961));
#37463=CARTESIAN_POINT('Ctrl Pts',(4.23639070615337,57.495,5.00273172317863));
#37464=CARTESIAN_POINT('Ctrl Pts',(4.27929023600674,57.495,5.02256507114894));
#37465=CARTESIAN_POINT('Ctrl Pts',(4.3233115657319,57.495,5.04203735157412));
#37466=CARTESIAN_POINT('Ctrl Pts',(4.36840670797617,57.495,5.06109712122989));
#37467=CARTESIAN_POINT('Ctrl Pts',(4.41453743405677,57.495,5.07970066295468));
#37468=CARTESIAN_POINT('Ctrl Pts',(4.46167734280651,57.495,5.09781475579217));
#37469=CARTESIAN_POINT('Ctrl Pts',(4.50980818622101,57.495,5.11541439426204));
#37470=CARTESIAN_POINT('Ctrl Pts',(4.5589176169425,57.495,5.13248213818666));
#37471=CARTESIAN_POINT('Ctrl Pts',(4.60899638270439,57.495,5.14900691787064));
#37472=CARTESIAN_POINT('Ctrl Pts',(4.66003509375265,57.495,5.16498334493456));
#37473=CARTESIAN_POINT('Ctrl Pts',(4.71202254995864,57.495,5.18041062500752));
#37474=CARTESIAN_POINT('Ctrl Pts',(4.7649478905793,57.495,5.19529077281773));
#37475=CARTESIAN_POINT('Ctrl Pts',(4.80803098811744,57.495,5.20675982149348));
#37476=CARTESIAN_POINT('Ctrl Pts',(4.84075823631826,57.495,5.21511826561704));
#37477=CARTESIAN_POINT('Ctrl Pts',(4.86276047837859,57.495,5.2205826053545));
#37478=CARTESIAN_POINT('Ctrl Pts',(4.87380761862879,57.495,5.22328778611671));
#37479=CARTESIAN_POINT('',(5.22328778611671,57.495,4.87380761862879));
#37480=CARTESIAN_POINT('Origin',(1.15195721078055E-12,57.495,1.15136842610855E-12));
#37481=CARTESIAN_POINT('',(4.65970441290368,57.495,3.72730711280926));
#37482=CARTESIAN_POINT('Ctrl Pts',(4.65970441290368,57.495,3.72730711280926));
#37483=CARTESIAN_POINT('Ctrl Pts',(4.66270326064961,57.495,3.72981733050576));
#37484=CARTESIAN_POINT('Ctrl Pts',(4.6688153380502,57.495,3.73509073349854));
#37485=CARTESIAN_POINT('Ctrl Pts',(4.67832660775297,57.495,3.7437597489088));
#37486=CARTESIAN_POINT('Ctrl Pts',(4.69169578253142,57.495,3.7568389360361));
#37487=CARTESIAN_POINT('Ctrl Pts',(4.70954474005187,57.495,3.77572337177426));
#37488=CARTESIAN_POINT('Ctrl Pts',(4.72849227702429,57.495,3.79711783384759));
#37489=CARTESIAN_POINT('Ctrl Pts',(4.74845295472311,57.495,3.82095228990398));
#37490=CARTESIAN_POINT('Ctrl Pts',(4.76926976684248,57.495,3.84708445224628));
#37491=CARTESIAN_POINT('Ctrl Pts',(4.79071829540097,57.495,3.87530262274579));
#37492=CARTESIAN_POINT('Ctrl Pts',(4.81254694822028,57.495,3.90536636162316));
#37493=CARTESIAN_POINT('Ctrl Pts',(4.83450929444277,57.495,3.93703846717723));
#37494=CARTESIAN_POINT('Ctrl Pts',(4.85639607415679,57.495,3.97011673859275));
#37495=CARTESIAN_POINT('Ctrl Pts',(4.87807598288661,57.495,4.00447382552398));
#37496=CARTESIAN_POINT('Ctrl Pts',(4.89949292161193,57.495,4.04005493051016));
#37497=CARTESIAN_POINT('Ctrl Pts',(4.92063739759527,57.495,4.07685036350543));
#37498=CARTESIAN_POINT('Ctrl Pts',(4.94152548435404,57.495,4.11487510765792));
#37499=CARTESIAN_POINT('Ctrl Pts',(4.9621766920072,57.495,4.15414724283855));
#37500=CARTESIAN_POINT('Ctrl Pts',(4.98258807456953,57.495,4.19466216292523));
#37501=CARTESIAN_POINT('Ctrl Pts',(5.00273172317852,57.495,4.23639070615327));
#37502=CARTESIAN_POINT('Ctrl Pts',(5.02256507114883,57.495,4.27929023600664));
#37503=CARTESIAN_POINT('Ctrl Pts',(5.04203735157409,57.495,4.32331156573186));
#37504=CARTESIAN_POINT('Ctrl Pts',(5.06109712122993,57.495,4.36840670797621));
#37505=CARTESIAN_POINT('Ctrl Pts',(5.07970066295481,57.495,4.41453743405689));
#37506=CARTESIAN_POINT('Ctrl Pts',(5.09781475579234,57.495,4.46167734280668));
#37507=CARTESIAN_POINT('Ctrl Pts',(5.11541439426219,57.495,4.50980818622117));
#37508=CARTESIAN_POINT('Ctrl Pts',(5.13248213818673,57.495,4.55891761694258));
#37509=CARTESIAN_POINT('Ctrl Pts',(5.14900691787061,57.495,4.60899638270436));
#37510=CARTESIAN_POINT('Ctrl Pts',(5.16498334493441,57.495,4.66003509375248));
#37511=CARTESIAN_POINT('Ctrl Pts',(5.1804106250073,57.495,4.71202254995837));
#37512=CARTESIAN_POINT('Ctrl Pts',(5.1952907728175,57.495,4.764947890579));
#37513=CARTESIAN_POINT('Ctrl Pts',(5.2067598214933,57.495,4.8080309881172));
#37514=CARTESIAN_POINT('Ctrl Pts',(5.21511826561693,57.495,4.84075823631811));
#37515=CARTESIAN_POINT('Ctrl Pts',(5.22058260535447,57.495,4.86276047837853));
#37516=CARTESIAN_POINT('Ctrl Pts',(5.22328778611671,57.495,4.87380761862879));
#37517=CARTESIAN_POINT('',(4.18409499139877,57.495,3.34686616149372));
#37518=CARTESIAN_POINT('',(4.06695907338649,57.495,3.25316890053365));
#37519=CARTESIAN_POINT('',(4.69328497730872,57.495,2.58480949428933));
#37520=CARTESIAN_POINT('Origin',(0.,57.495,0.));
#37521=CARTESIAN_POINT('',(5.22677443144495,57.495,2.87862685522557));
#37522=CARTESIAN_POINT('',(5.22677443144495,57.495,2.87862685522557));
#37523=CARTESIAN_POINT('',(6.50167680247051,57.495,2.96056324982543));
#37524=CARTESIAN_POINT('Ctrl Pts',(5.22677443144495,57.495,2.87862685522557));
#37525=CARTESIAN_POINT('Ctrl Pts',(5.23024117954545,57.495,2.88043681055505));
#37526=CARTESIAN_POINT('Ctrl Pts',(5.23745215939571,57.495,2.88406558980901));
#37527=CARTESIAN_POINT('Ctrl Pts',(5.24910109063628,57.495,2.88953536864313));
#37528=CARTESIAN_POINT('Ctrl Pts',(5.26630084561719,57.495,2.89688168736508));
#37529=CARTESIAN_POINT('Ctrl Pts',(5.29057828960676,57.495,2.90614521320837));
#37530=CARTESIAN_POINT('Ctrl Pts',(5.31759510370885,57.495,2.91546314862892));
#37531=CARTESIAN_POINT('Ctrl Pts',(5.34725389048201,57.495,2.92478335875774));
#37532=CARTESIAN_POINT('Ctrl Pts',(5.37936310952307,57.495,2.93401523982671));
#37533=CARTESIAN_POINT('Ctrl Pts',(5.41364129622045,57.495,2.94303247002258));
#37534=CARTESIAN_POINT('Ctrl Pts',(5.44977003302482,57.495,2.95169462080131));
#37535=CARTESIAN_POINT('Ctrl Pts',(5.48743586913296,57.495,2.9598647928985));
#37536=CARTESIAN_POINT('Ctrl Pts',(5.52637191504895,57.495,2.96742703426683));
#37537=CARTESIAN_POINT('Ctrl Pts',(5.56641026634749,57.495,2.97430877025609));
#37538=CARTESIAN_POINT('Ctrl Pts',(5.60747882861049,57.495,2.98047914221));
#37539=CARTESIAN_POINT('Ctrl Pts',(5.64956501668959,57.495,2.98593308820271));
#37540=CARTESIAN_POINT('Ctrl Pts',(5.69268882427748,57.495,2.9906797244254));
#37541=CARTESIAN_POINT('Ctrl Pts',(5.73687442119613,57.495,2.9947301570106));
#37542=CARTESIAN_POINT('Ctrl Pts',(5.78211642456387,57.495,2.99808342690946));
#37543=CARTESIAN_POINT('Ctrl Pts',(5.82837721216385,57.495,3.00072490941932));
#37544=CARTESIAN_POINT('Ctrl Pts',(5.87560110342631,57.495,3.00263159433912));
#37545=CARTESIAN_POINT('Ctrl Pts',(5.9237232280624,57.495,3.00377540211878));
#37546=CARTESIAN_POINT('Ctrl Pts',(5.97267956506952,57.495,3.00412716938109));
#37547=CARTESIAN_POINT('Ctrl Pts',(6.02241806591666,57.495,3.00366113621883));
#37548=CARTESIAN_POINT('Ctrl Pts',(6.07290162599622,57.495,3.00235671375967));
#37549=CARTESIAN_POINT('Ctrl Pts',(6.12410381716742,57.495,3.00019778316108));
#37550=CARTESIAN_POINT('Ctrl Pts',(6.17600655789209,57.495,2.99717295692919));
#37551=CARTESIAN_POINT('Ctrl Pts',(6.22859706400147,57.495,2.99327554868811));
#37552=CARTESIAN_POINT('Ctrl Pts',(6.28186459845047,57.495,2.98850417352769));
#37553=CARTESIAN_POINT('Ctrl Pts',(6.33579850967689,57.495,2.98286238364858));
#37554=CARTESIAN_POINT('Ctrl Pts',(6.39038953466561,57.495,2.97635619664337));
#37555=CARTESIAN_POINT('Ctrl Pts',(6.43458214159149,57.495,2.97046502832946));
#37556=CARTESIAN_POINT('Ctrl Pts',(6.46801681444607,57.495,2.9656630481055));
#37557=CARTESIAN_POINT('Ctrl Pts',(6.49043534784131,57.495,2.96229154623625));
#37558=CARTESIAN_POINT('Ctrl Pts',(6.50167680247051,57.495,2.96056324982543));
#37559=CARTESIAN_POINT('',(6.69081410619341,57.495,2.50394540602692));
#37560=CARTESIAN_POINT('Origin',(1.50487931058895E-12,57.495,6.22890783902203E-13));
#37561=CARTESIAN_POINT('',(5.73138421404289,57.495,1.66039107437148));
#37562=CARTESIAN_POINT('Ctrl Pts',(5.73138421404289,57.495,1.66039107437148));
#37563=CARTESIAN_POINT('Ctrl Pts',(5.73511540682056,57.495,1.66156260377487));
#37564=CARTESIAN_POINT('Ctrl Pts',(5.7427802739896,57.495,1.66409560210805));
#37565=CARTESIAN_POINT('Ctrl Pts',(5.75488502996861,57.495,1.6684649226766));
#37566=CARTESIAN_POINT('Ctrl Pts',(5.77224172513541,57.495,1.67543235427329));
#37567=CARTESIAN_POINT('Ctrl Pts',(5.79595877235177,57.495,1.68604879760674));
#37568=CARTESIAN_POINT('Ctrl Pts',(5.82165132013192,57.495,1.69856379474191));
#37569=CARTESIAN_POINT('Ctrl Pts',(5.84921363316513,57.495,1.71294534020683));
#37570=CARTESIAN_POINT('Ctrl Pts',(5.87844620539462,57.495,1.72912206102241));
#37571=CARTESIAN_POINT('Ctrl Pts',(5.90906068827411,57.495,1.74698425466387));
#37572=CARTESIAN_POINT('Ctrl Pts',(5.94073262861949,57.495,1.76640606389864));
#37573=CARTESIAN_POINT('Ctrl Pts',(5.97314358084403,57.495,1.78726264793637));
#37574=CARTESIAN_POINT('Ctrl Pts',(6.0060228350964,57.495,1.80944727788364));
#37575=CARTESIAN_POINT('Ctrl Pts',(6.03920034699149,57.495,1.83289254541003));
#37576=CARTESIAN_POINT('Ctrl Pts',(6.07260331771232,57.495,1.85756929242874));
#37577=CARTESIAN_POINT('Ctrl Pts',(6.10621926889299,57.495,1.88347219921809));
#37578=CARTESIAN_POINT('Ctrl Pts',(6.14006878432982,57.495,1.91060895733317));
#37579=CARTESIAN_POINT('Ctrl Pts',(6.17417680788945,57.495,1.93898880419737));
#37580=CARTESIAN_POINT('Ctrl Pts',(6.20853885514981,57.495,1.96860861168851));
#37581=CARTESIAN_POINT('Ctrl Pts',(6.24311798195985,57.495,1.99945211810837));
#37582=CARTESIAN_POINT('Ctrl Pts',(6.27785854554194,57.495,2.03149622201769));
#37583=CARTESIAN_POINT('Ctrl Pts',(6.31269482043467,57.495,2.06471490843563));
#37584=CARTESIAN_POINT('Ctrl Pts',(6.34756091533115,57.495,2.09908352929888));
#37585=CARTESIAN_POINT('Ctrl Pts',(6.38240181135703,57.495,2.13458349574329));
#37586=CARTESIAN_POINT('Ctrl Pts',(6.41717671306138,57.495,2.17120312938042));
#37587=CARTESIAN_POINT('Ctrl Pts',(6.45185553518375,57.495,2.20893514043555));
#37588=CARTESIAN_POINT('Ctrl Pts',(6.48641743997175,57.495,2.24777479550457));
#37589=CARTESIAN_POINT('Ctrl Pts',(6.52084865967127,57.495,2.2877177827968));
#37590=CARTESIAN_POINT('Ctrl Pts',(6.55514062276556,57.495,2.32875748935421));
#37591=CARTESIAN_POINT('Ctrl Pts',(6.58928830924802,57.495,2.37088387159981));
#37592=CARTESIAN_POINT('Ctrl Pts',(6.6232894242584,57.495,2.41408612451229));
#37593=CARTESIAN_POINT('Ctrl Pts',(6.65037263123018,57.495,2.4495007016118));
#37594=CARTESIAN_POINT('Ctrl Pts',(6.67061900235304,57.495,2.47653809829358));
#37595=CARTESIAN_POINT('Ctrl Pts',(6.68408728750664,57.495,2.49477440711619));
#37596=CARTESIAN_POINT('Ctrl Pts',(6.69081410619341,57.495,2.50394540602692));
#37597=CARTESIAN_POINT('',(5.1463899549833,57.495,1.4909173120086));
#37598=CARTESIAN_POINT('',(5.00231408838243,57.495,1.4491783055134));
#37599=CARTESIAN_POINT('',(5.32519370006274,57.495,0.592010183030742));
#37600=CARTESIAN_POINT('Origin',(0.,57.495,0.));
#37601=CARTESIAN_POINT('',(5.93051272372135,57.495,0.659304453656786));
#37602=CARTESIAN_POINT('',(5.93051272372135,57.495,0.659304453656786));
#37603=CARTESIAN_POINT('',(7.13972463098307,57.495,0.247119796320915));
#37604=CARTESIAN_POINT('Ctrl Pts',(5.93051272372135,57.495,0.659304453656786));
#37605=CARTESIAN_POINT('Ctrl Pts',(5.93440822125369,57.495,0.659649967278209));
#37606=CARTESIAN_POINT('Ctrl Pts',(5.94245897164689,57.495,0.66024299963913));
#37607=CARTESIAN_POINT('Ctrl Pts',(5.95531437453421,57.495,0.660838563360811));
#37608=CARTESIAN_POINT('Ctrl Pts',(5.97401619058905,57.495,0.661043615595394));
#37609=CARTESIAN_POINT('Ctrl Pts',(5.99999062205821,57.495,0.660311421925918));
#37610=CARTESIAN_POINT('Ctrl Pts',(6.02851672315009,57.495,0.658581184594064));
#37611=CARTESIAN_POINT('Ctrl Pts',(6.05948455921138,57.495,0.655842009648653));
#37612=CARTESIAN_POINT('Ctrl Pts',(6.092682497423,57.495,0.652083489461662));
#37613=CARTESIAN_POINT('Ctrl Pts',(6.12780215712609,57.495,0.647296629738963));
#37614=CARTESIAN_POINT('Ctrl Pts',(6.16449561918681,57.495,0.641473544543642));
#37615=CARTESIAN_POINT('Ctrl Pts',(6.2024209037432,57.495,0.634607707876569));
#37616=CARTESIAN_POINT('Ctrl Pts',(6.24128706412512,57.495,0.626694128202827));
#37617=CARTESIAN_POINT('Ctrl Pts',(6.28091120375433,57.495,0.617730009530282));
#37618=CARTESIAN_POINT('Ctrl Pts',(6.32121490697708,57.495,0.607714431517377));
#37619=CARTESIAN_POINT('Ctrl Pts',(6.36218460951721,57.495,0.596647533682194));
#37620=CARTESIAN_POINT('Ctrl Pts',(6.40384227175349,57.495,0.584530087032232));
#37621=CARTESIAN_POINT('Ctrl Pts',(6.4462144738227,57.495,0.571363102905584));
#37622=CARTESIAN_POINT('Ctrl Pts',(6.48929587557851,57.495,0.557147755196286));
#37623=CARTESIAN_POINT('Ctrl Pts',(6.53304612199338,57.495,0.541884929839957));
#37624=CARTESIAN_POINT('Ctrl Pts',(6.57740496530586,57.495,0.525574676214359));
#37625=CARTESIAN_POINT('Ctrl Pts',(6.62230172760518,57.495,0.508215876982666));
#37626=CARTESIAN_POINT('Ctrl Pts',(6.66766610085612,57.495,0.489806088474619));
#37627=CARTESIAN_POINT('Ctrl Pts',(6.71344014059646,57.495,0.470341429749655));
#37628=CARTESIAN_POINT('Ctrl Pts',(6.75958168761835,57.495,0.449817078488633));
#37629=CARTESIAN_POINT('Ctrl Pts',(6.80606015708944,57.495,0.42822825643448));
#37630=CARTESIAN_POINT('Ctrl Pts',(6.85285448604147,57.495,0.405571362419761));
#37631=CARTESIAN_POINT('Ctrl Pts',(6.89995030467732,57.495,0.38184511132823));
#37632=CARTESIAN_POINT('Ctrl Pts',(6.94733716327859,57.495,0.357052332559016));
#37633=CARTESIAN_POINT('Ctrl Pts',(6.99500658045334,57.495,0.331200384093974));
#37634=CARTESIAN_POINT('Ctrl Pts',(7.04295230112448,57.495,0.304298370266161));
#37635=CARTESIAN_POINT('Ctrl Pts',(7.0815264936406,57.495,0.281943861934802));
#37636=CARTESIAN_POINT('Ctrl Pts',(7.1105784652929,57.495,0.264712515322363));
#37637=CARTESIAN_POINT('Ctrl Pts',(7.13000027153814,57.495,0.253018452443265));
#37638=CARTESIAN_POINT('Ctrl Pts',(7.13972463098307,57.495,0.247119796320915));
#37639=CARTESIAN_POINT('',(7.13972463098307,57.495,-0.247119796320921));
#37640=CARTESIAN_POINT('Origin',(1.6286971771251E-12,57.495,-4.16333634234733E-16));
#37641=CARTESIAN_POINT('',(5.93051272372135,57.495,-0.659304453656789));
#37642=CARTESIAN_POINT('Ctrl Pts',(5.93051272372135,57.495,-0.659304453656789));
#37643=CARTESIAN_POINT('Ctrl Pts',(5.9344082212537,57.495,-0.659649967278237));
#37644=CARTESIAN_POINT('Ctrl Pts',(5.94245897164691,57.495,-0.660242999639202));
#37645=CARTESIAN_POINT('Ctrl Pts',(5.95531437453424,57.495,-0.660838563360922));
#37646=CARTESIAN_POINT('Ctrl Pts',(5.97401619058907,57.495,-0.661043615595513));
#37647=CARTESIAN_POINT('Ctrl Pts',(5.99999062205823,57.495,-0.660311421925998));
#37648=CARTESIAN_POINT('Ctrl Pts',(6.0285167231501,57.495,-0.658581184594089));
#37649=CARTESIAN_POINT('Ctrl Pts',(6.05948455921138,57.495,-0.655842009648634));
#37650=CARTESIAN_POINT('Ctrl Pts',(6.09268249742298,57.495,-0.652083489461621));
#37651=CARTESIAN_POINT('Ctrl Pts',(6.12780215712604,57.495,-0.647296629738921));
#37652=CARTESIAN_POINT('Ctrl Pts',(6.16449561918676,57.495,-0.641473544543615));
#37653=CARTESIAN_POINT('Ctrl Pts',(6.20242090374318,57.495,-0.634607707876565));
#37654=CARTESIAN_POINT('Ctrl Pts',(6.24128706412515,57.495,-0.626694128202843));
#37655=CARTESIAN_POINT('Ctrl Pts',(6.2809112037544,57.495,-0.617730009530308));
#37656=CARTESIAN_POINT('Ctrl Pts',(6.32121490697716,57.495,-0.607714431517403));
#37657=CARTESIAN_POINT('Ctrl Pts',(6.36218460951727,57.495,-0.596647533682212));
#37658=CARTESIAN_POINT('Ctrl Pts',(6.40384227175352,57.495,-0.584530087032239));
#37659=CARTESIAN_POINT('Ctrl Pts',(6.44621447382266,57.495,-0.57136310290558));
#37660=CARTESIAN_POINT('Ctrl Pts',(6.4892958755784,57.495,-0.557147755196278));
#37661=CARTESIAN_POINT('Ctrl Pts',(6.53304612199323,57.495,-0.541884929839951));
#37662=CARTESIAN_POINT('Ctrl Pts',(6.57740496530571,57.495,-0.525574676214357));
#37663=CARTESIAN_POINT('Ctrl Pts',(6.62230172760513,57.495,-0.508215876982669));
#37664=CARTESIAN_POINT('Ctrl Pts',(6.66766610085618,57.495,-0.489806088474624));
#37665=CARTESIAN_POINT('Ctrl Pts',(6.71344014059664,57.495,-0.470341429749656));
#37666=CARTESIAN_POINT('Ctrl Pts',(6.75958168761858,57.495,-0.44981707848863));
#37667=CARTESIAN_POINT('Ctrl Pts',(6.80606015708966,57.495,-0.428228256434474));
#37668=CARTESIAN_POINT('Ctrl Pts',(6.85285448604159,57.495,-0.405571362419757));
#37669=CARTESIAN_POINT('Ctrl Pts',(6.89995030467727,57.495,-0.381845111328236));
#37670=CARTESIAN_POINT('Ctrl Pts',(6.94733716327837,57.495,-0.357052332559036));
#37671=CARTESIAN_POINT('Ctrl Pts',(6.99500658045299,57.495,-0.33120038409401));
#37672=CARTESIAN_POINT('Ctrl Pts',(7.0429523011241,57.495,-0.304298370266206));
#37673=CARTESIAN_POINT('Ctrl Pts',(7.0815264936403,57.495,-0.281943861934841));
#37674=CARTESIAN_POINT('Ctrl Pts',(7.11057846529273,57.495,-0.264712515322388));
#37675=CARTESIAN_POINT('Ctrl Pts',(7.13000027153808,57.495,-0.253018452443277));
#37676=CARTESIAN_POINT('Ctrl Pts',(7.13972463098307,57.495,-0.247119796320918));
#37677=CARTESIAN_POINT('',(5.32519370006274,57.495,-0.592010183030745));
#37678=CARTESIAN_POINT('',(5.17611212951227,57.495,-0.575436549687219));
#37679=CARTESIAN_POINT('',(5.1463899549833,57.495,-1.4909173120086));
#37680=CARTESIAN_POINT('Origin',(0.,57.495,0.));
#37681=CARTESIAN_POINT('',(5.73138421404289,57.495,-1.66039107437149));
#37682=CARTESIAN_POINT('',(5.73138421404289,57.495,-1.66039107437149));
#37683=CARTESIAN_POINT('',(6.6908141061934,57.495,-2.50394540602693));
#37684=CARTESIAN_POINT('Ctrl Pts',(5.73138421404289,57.495,-1.66039107437149));
#37685=CARTESIAN_POINT('Ctrl Pts',(5.73511540682054,57.495,-1.66156260377489));
#37686=CARTESIAN_POINT('Ctrl Pts',(5.74278027398956,57.495,-1.66409560210811));
#37687=CARTESIAN_POINT('Ctrl Pts',(5.75488502996854,57.495,-1.6684649226767));
#37688=CARTESIAN_POINT('Ctrl Pts',(5.77224172513534,57.495,-1.67543235427339));
#37689=CARTESIAN_POINT('Ctrl Pts',(5.79595877235173,57.495,-1.68604879760681));
#37690=CARTESIAN_POINT('Ctrl Pts',(5.8216513201319,57.495,-1.69856379474193));
#37691=CARTESIAN_POINT('Ctrl Pts',(5.84921363316514,57.495,-1.71294534020682));
#37692=CARTESIAN_POINT('Ctrl Pts',(5.87844620539466,57.495,-1.72912206102238));
#37693=CARTESIAN_POINT('Ctrl Pts',(5.90906068827417,57.495,-1.74698425466385));
#37694=CARTESIAN_POINT('Ctrl Pts',(5.94073262861954,57.495,-1.76640606389863));
#37695=CARTESIAN_POINT('Ctrl Pts',(5.97314358084405,57.495,-1.78726264793637));
#37696=CARTESIAN_POINT('Ctrl Pts',(6.00602283509636,57.495,-1.80944727788364));
#37697=CARTESIAN_POINT('Ctrl Pts',(6.03920034699142,57.495,-1.83289254541003));
#37698=CARTESIAN_POINT('Ctrl Pts',(6.07260331771223,57.495,-1.85756929242873));
#37699=CARTESIAN_POINT('Ctrl Pts',(6.10621926889293,57.495,-1.88347219921808));
#37700=CARTESIAN_POINT('Ctrl Pts',(6.14006878432979,57.495,-1.91060895733316));
#37701=CARTESIAN_POINT('Ctrl Pts',(6.17417680788948,57.495,-1.93898880419739));
#37702=CARTESIAN_POINT('Ctrl Pts',(6.20853885514991,57.495,-1.96860861168855));
#37703=CARTESIAN_POINT('Ctrl Pts',(6.24311798195999,57.495,-1.99945211810842));
#37704=CARTESIAN_POINT('Ctrl Pts',(6.27785854554207,57.495,-2.03149622201774));
#37705=CARTESIAN_POINT('Ctrl Pts',(6.31269482043472,57.495,-2.06471490843566));
#37706=CARTESIAN_POINT('Ctrl Pts',(6.34756091533109,57.495,-2.09908352929886));
#37707=CARTESIAN_POINT('Ctrl Pts',(6.38240181135686,57.495,-2.13458349574322));
#37708=CARTESIAN_POINT('Ctrl Pts',(6.41717671306116,57.495,-2.17120312938033));
#37709=CARTESIAN_POINT('Ctrl Pts',(6.45185553518355,57.495,-2.20893514043546));
#37710=CARTESIAN_POINT('Ctrl Pts',(6.48641743997165,57.495,-2.24777479550452));
#37711=CARTESIAN_POINT('Ctrl Pts',(6.52084865967131,57.495,-2.28771778279682));
#37712=CARTESIAN_POINT('Ctrl Pts',(6.55514062276576,57.495,-2.32875748935431));
#37713=CARTESIAN_POINT('Ctrl Pts',(6.58928830924832,57.495,-2.37088387159998));
#37714=CARTESIAN_POINT('Ctrl Pts',(6.62328942425873,57.495,-2.41408612451248));
#37715=CARTESIAN_POINT('Ctrl Pts',(6.65037263123044,57.495,-2.44950070161195));
#37716=CARTESIAN_POINT('Ctrl Pts',(6.67061900235319,57.495,-2.47653809829367));
#37717=CARTESIAN_POINT('Ctrl Pts',(6.6840872875067,57.495,-2.49477440711623));
#37718=CARTESIAN_POINT('Ctrl Pts',(6.6908141061934,57.495,-2.50394540602693));
#37719=CARTESIAN_POINT('',(6.5016768024705,57.495,-2.96056324982543));
#37720=CARTESIAN_POINT('Origin',(1.50456066262064E-12,57.495,-6.23660068148934E-13));
#37721=CARTESIAN_POINT('',(5.22677443144495,57.495,-2.87862685522557));
#37722=CARTESIAN_POINT('Ctrl Pts',(5.22677443144495,57.495,-2.87862685522557));
#37723=CARTESIAN_POINT('Ctrl Pts',(5.23024117954544,57.495,-2.88043681055508));
#37724=CARTESIAN_POINT('Ctrl Pts',(5.2374521593957,57.495,-2.88406558980908));
#37725=CARTESIAN_POINT('Ctrl Pts',(5.24910109063627,57.495,-2.88953536864324));
#37726=CARTESIAN_POINT('Ctrl Pts',(5.26630084561717,57.495,-2.8968816873652));
#37727=CARTESIAN_POINT('Ctrl Pts',(5.29057828960674,57.495,-2.90614521320845));
#37728=CARTESIAN_POINT('Ctrl Pts',(5.31759510370885,57.495,-2.91546314862894));
#37729=CARTESIAN_POINT('Ctrl Pts',(5.34725389048201,57.495,-2.92478335875772));
#37730=CARTESIAN_POINT('Ctrl Pts',(5.37936310952306,57.495,-2.93401523982667));
#37731=CARTESIAN_POINT('Ctrl Pts',(5.41364129622042,57.495,-2.94303247002252));
#37732=CARTESIAN_POINT('Ctrl Pts',(5.44977003302479,57.495,-2.95169462080126));
#37733=CARTESIAN_POINT('Ctrl Pts',(5.48743586913294,57.495,-2.95986479289849));
#37734=CARTESIAN_POINT('Ctrl Pts',(5.52637191504897,57.495,-2.96742703426686));
#37735=CARTESIAN_POINT('Ctrl Pts',(5.56641026634754,57.495,-2.97430877025614));
#37736=CARTESIAN_POINT('Ctrl Pts',(5.60747882861056,57.495,-2.98047914221006));
#37737=CARTESIAN_POINT('Ctrl Pts',(5.64956501668965,57.495,-2.98593308820275));
#37738=CARTESIAN_POINT('Ctrl Pts',(5.6926888242775,57.495,-2.99067972442542));
#37739=CARTESIAN_POINT('Ctrl Pts',(5.73687442119609,57.495,-2.99473015701059));
#37740=CARTESIAN_POINT('Ctrl Pts',(5.78211642456377,57.495,-2.99808342690941));
#37741=CARTESIAN_POINT('Ctrl Pts',(5.82837721216371,57.495,-3.00072490941926));
#37742=CARTESIAN_POINT('Ctrl Pts',(5.87560110342618,57.495,-3.00263159433907));
#37743=CARTESIAN_POINT('Ctrl Pts',(5.92372322806235,57.495,-3.00377540211876));
#37744=CARTESIAN_POINT('Ctrl Pts',(5.97267956506957,57.495,-3.00412716938112));
#37745=CARTESIAN_POINT('Ctrl Pts',(6.02241806591682,57.495,-3.0036611362189));
#37746=CARTESIAN_POINT('Ctrl Pts',(6.07290162599645,57.495,-3.00235671375976));
#37747=CARTESIAN_POINT('Ctrl Pts',(6.12410381716763,57.495,-3.00019778316116));
#37748=CARTESIAN_POINT('Ctrl Pts',(6.17600655789219,57.495,-2.99717295692923));
#37749=CARTESIAN_POINT('Ctrl Pts',(6.22859706400143,57.495,-2.9932755486881));
#37750=CARTESIAN_POINT('Ctrl Pts',(6.28186459845025,57.495,-2.98850417352762));
#37751=CARTESIAN_POINT('Ctrl Pts',(6.33579850967655,57.495,-2.98286238364848));
#37752=CARTESIAN_POINT('Ctrl Pts',(6.39038953466525,57.495,-2.97635619664327));
#37753=CARTESIAN_POINT('Ctrl Pts',(6.43458214159119,57.495,-2.97046502832938));
#37754=CARTESIAN_POINT('Ctrl Pts',(6.4680168144459,57.495,-2.96566304810545));
#37755=CARTESIAN_POINT('Ctrl Pts',(6.49043534784125,57.495,-2.96229154623624));
#37756=CARTESIAN_POINT('Ctrl Pts',(6.5016768024705,57.495,-2.96056324982543));
#37757=CARTESIAN_POINT('',(4.69328497730872,57.495,-2.58480949428933));
#37758=CARTESIAN_POINT('',(4.56189402049717,57.495,-2.51244640654327));
#37759=CARTESIAN_POINT('',(4.18409499139877,57.495,-3.34686616149372));
#37760=CARTESIAN_POINT('Origin',(0.,57.495,0.));
#37761=CARTESIAN_POINT('',(4.65970441290367,57.495,-3.72730711280926));
#37762=CARTESIAN_POINT('',(4.65970441290367,57.495,-3.72730711280926));
#37763=CARTESIAN_POINT('',(5.22328778611671,57.495,-4.87380761862879));
#37764=CARTESIAN_POINT('Ctrl Pts',(4.65970441290367,57.495,-3.72730711280926));
#37765=CARTESIAN_POINT('Ctrl Pts',(4.66270326064959,57.495,-3.72981733050578));
#37766=CARTESIAN_POINT('Ctrl Pts',(4.66881533805013,57.495,-3.73509073349858));
#37767=CARTESIAN_POINT('Ctrl Pts',(4.67832660775287,57.495,-3.74375974890886));
#37768=CARTESIAN_POINT('Ctrl Pts',(4.69169578253132,57.495,-3.75683893603616));
#37769=CARTESIAN_POINT('Ctrl Pts',(4.7095447400518,57.495,-3.77572337177431));
#37770=CARTESIAN_POINT('Ctrl Pts',(4.72849227702427,57.495,-3.7971178338476));
#37771=CARTESIAN_POINT('Ctrl Pts',(4.74845295472312,57.495,-3.82095228990397));
#37772=CARTESIAN_POINT('Ctrl Pts',(4.76926976684252,57.495,-3.84708445224627));
#37773=CARTESIAN_POINT('Ctrl Pts',(4.79071829540103,57.495,-3.8753026227458));
#37774=CARTESIAN_POINT('Ctrl Pts',(4.81254694822034,57.495,-3.90536636162318));
#37775=CARTESIAN_POINT('Ctrl Pts',(4.83450929444279,57.495,-3.93703846717724));
#37776=CARTESIAN_POINT('Ctrl Pts',(4.85639607415676,57.495,-3.97011673859274));
#37777=CARTESIAN_POINT('Ctrl Pts',(4.87807598288654,57.495,-4.00447382552396));
#37778=CARTESIAN_POINT('Ctrl Pts',(4.89949292161185,57.495,-4.04005493051012));
#37779=CARTESIAN_POINT('Ctrl Pts',(4.92063739759521,57.495,-4.07685036350539));
#37780=CARTESIAN_POINT('Ctrl Pts',(4.94152548435402,57.495,-4.11487510765791));
#37781=CARTESIAN_POINT('Ctrl Pts',(4.96217669200723,57.495,-4.15414724283858));
#37782=CARTESIAN_POINT('Ctrl Pts',(4.98258807456962,57.495,-4.1946621629253));
#37783=CARTESIAN_POINT('Ctrl Pts',(5.00273172317863,57.495,-4.23639070615337));
#37784=CARTESIAN_POINT('Ctrl Pts',(5.02256507114894,57.495,-4.27929023600674));
#37785=CARTESIAN_POINT('Ctrl Pts',(5.04203735157413,57.495,-4.3233115657319));
#37786=CARTESIAN_POINT('Ctrl Pts',(5.06109712122989,57.495,-4.36840670797617));
#37787=CARTESIAN_POINT('Ctrl Pts',(5.07970066295468,57.495,-4.41453743405677));
#37788=CARTESIAN_POINT('Ctrl Pts',(5.09781475579217,57.495,-4.46167734280651));
#37789=CARTESIAN_POINT('Ctrl Pts',(5.11541439426204,57.495,-4.50980818622101));
#37790=CARTESIAN_POINT('Ctrl Pts',(5.13248213818666,57.495,-4.5589176169425));
#37791=CARTESIAN_POINT('Ctrl Pts',(5.14900691787064,57.495,-4.60899638270439));
#37792=CARTESIAN_POINT('Ctrl Pts',(5.16498334493456,57.495,-4.66003509375265));
#37793=CARTESIAN_POINT('Ctrl Pts',(5.18041062500752,57.495,-4.71202254995864));
#37794=CARTESIAN_POINT('Ctrl Pts',(5.19529077281773,57.495,-4.7649478905793));
#37795=CARTESIAN_POINT('Ctrl Pts',(5.20675982149348,57.495,-4.80803098811744));
#37796=CARTESIAN_POINT('Ctrl Pts',(5.21511826561704,57.495,-4.84075823631826));
#37797=CARTESIAN_POINT('Ctrl Pts',(5.2205826053545,57.495,-4.86276047837859));
#37798=CARTESIAN_POINT('Ctrl Pts',(5.22328778611671,57.495,-4.87380761862879));
#37799=CARTESIAN_POINT('',(4.87380761862879,57.495,-5.22328778611671));
#37800=CARTESIAN_POINT('Origin',(1.15136842610855E-12,57.495,-1.15195721078055E-12));
#37801=CARTESIAN_POINT('',(3.72730711280926,57.495,-4.65970441290368));
#37802=CARTESIAN_POINT('Ctrl Pts',(3.72730711280926,57.495,-4.65970441290368));
#37803=CARTESIAN_POINT('Ctrl Pts',(3.72981733050576,57.495,-4.66270326064961));
#37804=CARTESIAN_POINT('Ctrl Pts',(3.73509073349854,57.495,-4.6688153380502));
#37805=CARTESIAN_POINT('Ctrl Pts',(3.7437597489088,57.495,-4.67832660775297));
#37806=CARTESIAN_POINT('Ctrl Pts',(3.7568389360361,57.495,-4.69169578253142));
#37807=CARTESIAN_POINT('Ctrl Pts',(3.77572337177426,57.495,-4.70954474005187));
#37808=CARTESIAN_POINT('Ctrl Pts',(3.79711783384759,57.495,-4.72849227702429));
#37809=CARTESIAN_POINT('Ctrl Pts',(3.82095228990398,57.495,-4.74845295472311));
#37810=CARTESIAN_POINT('Ctrl Pts',(3.84708445224628,57.495,-4.76926976684248));
#37811=CARTESIAN_POINT('Ctrl Pts',(3.87530262274579,57.495,-4.79071829540097));
#37812=CARTESIAN_POINT('Ctrl Pts',(3.90536636162316,57.495,-4.81254694822028));
#37813=CARTESIAN_POINT('Ctrl Pts',(3.93703846717723,57.495,-4.83450929444277));
#37814=CARTESIAN_POINT('Ctrl Pts',(3.97011673859275,57.495,-4.85639607415679));
#37815=CARTESIAN_POINT('Ctrl Pts',(4.00447382552398,57.495,-4.87807598288661));
#37816=CARTESIAN_POINT('Ctrl Pts',(4.04005493051016,57.495,-4.89949292161193));
#37817=CARTESIAN_POINT('Ctrl Pts',(4.07685036350543,57.495,-4.92063739759527));
#37818=CARTESIAN_POINT('Ctrl Pts',(4.11487510765792,57.495,-4.94152548435404));
#37819=CARTESIAN_POINT('Ctrl Pts',(4.15414724283855,57.495,-4.9621766920072));
#37820=CARTESIAN_POINT('Ctrl Pts',(4.19466216292523,57.495,-4.98258807456953));
#37821=CARTESIAN_POINT('Ctrl Pts',(4.23639070615327,57.495,-5.00273172317852));
#37822=CARTESIAN_POINT('Ctrl Pts',(4.27929023600664,57.495,-5.02256507114883));
#37823=CARTESIAN_POINT('Ctrl Pts',(4.32331156573186,57.495,-5.04203735157409));
#37824=CARTESIAN_POINT('Ctrl Pts',(4.36840670797621,57.495,-5.06109712122993));
#37825=CARTESIAN_POINT('Ctrl Pts',(4.41453743405689,57.495,-5.07970066295481));
#37826=CARTESIAN_POINT('Ctrl Pts',(4.46167734280668,57.495,-5.09781475579234));
#37827=CARTESIAN_POINT('Ctrl Pts',(4.50980818622117,57.495,-5.11541439426219));
#37828=CARTESIAN_POINT('Ctrl Pts',(4.55891761694258,57.495,-5.13248213818673));
#37829=CARTESIAN_POINT('Ctrl Pts',(4.60899638270436,57.495,-5.14900691787061));
#37830=CARTESIAN_POINT('Ctrl Pts',(4.66003509375248,57.495,-5.16498334493441));
#37831=CARTESIAN_POINT('Ctrl Pts',(4.71202254995837,57.495,-5.1804106250073));
#37832=CARTESIAN_POINT('Ctrl Pts',(4.764947890579,57.495,-5.1952907728175));
#37833=CARTESIAN_POINT('Ctrl Pts',(4.8080309881172,57.495,-5.2067598214933));
#37834=CARTESIAN_POINT('Ctrl Pts',(4.84075823631811,57.495,-5.21511826561693));
#37835=CARTESIAN_POINT('Ctrl Pts',(4.86276047837853,57.495,-5.22058260535447));
#37836=CARTESIAN_POINT('Ctrl Pts',(4.87380761862879,57.495,-5.22328778611671));
#37837=CARTESIAN_POINT('',(3.34686616149372,57.495,-4.18409499139877));
#37838=CARTESIAN_POINT('',(3.25316890053365,57.495,-4.06695907338649));
#37839=CARTESIAN_POINT('',(2.58480949428932,57.495,-4.69328497730873));
#37840=CARTESIAN_POINT('Origin',(0.,57.495,0.));
#37841=CARTESIAN_POINT('',(2.87862685522556,57.495,-5.22677443144495));
#37842=CARTESIAN_POINT('',(2.87862685522556,57.495,-5.22677443144495));
#37843=CARTESIAN_POINT('',(2.96056324982543,57.495,-6.50167680247051));
#37844=CARTESIAN_POINT('Ctrl Pts',(2.87862685522556,57.495,-5.22677443144495));
#37845=CARTESIAN_POINT('Ctrl Pts',(2.88043681055505,57.495,-5.23024117954545));
#37846=CARTESIAN_POINT('Ctrl Pts',(2.884065589809,57.495,-5.23745215939571));
#37847=CARTESIAN_POINT('Ctrl Pts',(2.88953536864313,57.495,-5.24910109063628));
#37848=CARTESIAN_POINT('Ctrl Pts',(2.89688168736508,57.495,-5.26630084561719));
#37849=CARTESIAN_POINT('Ctrl Pts',(2.90614521320837,57.495,-5.29057828960676));
#37850=CARTESIAN_POINT('Ctrl Pts',(2.91546314862891,57.495,-5.31759510370886));
#37851=CARTESIAN_POINT('Ctrl Pts',(2.92478335875774,57.495,-5.34725389048201));
#37852=CARTESIAN_POINT('Ctrl Pts',(2.93401523982671,57.495,-5.37936310952307));
#37853=CARTESIAN_POINT('Ctrl Pts',(2.94303247002258,57.495,-5.41364129622045));
#37854=CARTESIAN_POINT('Ctrl Pts',(2.95169462080131,57.495,-5.44977003302482));
#37855=CARTESIAN_POINT('Ctrl Pts',(2.95986479289849,57.495,-5.48743586913296));
#37856=CARTESIAN_POINT('Ctrl Pts',(2.96742703426683,57.495,-5.52637191504895));
#37857=CARTESIAN_POINT('Ctrl Pts',(2.97430877025608,57.495,-5.56641026634749));
#37858=CARTESIAN_POINT('Ctrl Pts',(2.98047914221,57.495,-5.6074788286105));
#37859=CARTESIAN_POINT('Ctrl Pts',(2.98593308820271,57.495,-5.64956501668959));
#37860=CARTESIAN_POINT('Ctrl Pts',(2.9906797244254,57.495,-5.69268882427748));
#37861=CARTESIAN_POINT('Ctrl Pts',(2.9947301570106,57.495,-5.73687442119613));
#37862=CARTESIAN_POINT('Ctrl Pts',(2.99808342690946,57.495,-5.78211642456387));
#37863=CARTESIAN_POINT('Ctrl Pts',(3.00072490941932,57.495,-5.82837721216385));
#37864=CARTESIAN_POINT('Ctrl Pts',(3.00263159433912,57.495,-5.87560110342631));
#37865=CARTESIAN_POINT('Ctrl Pts',(3.00377540211877,57.495,-5.9237232280624));
#37866=CARTESIAN_POINT('Ctrl Pts',(3.00412716938109,57.495,-5.97267956506952));
#37867=CARTESIAN_POINT('Ctrl Pts',(3.00366113621882,57.495,-6.02241806591666));
#37868=CARTESIAN_POINT('Ctrl Pts',(3.00235671375967,57.495,-6.07290162599622));
#37869=CARTESIAN_POINT('Ctrl Pts',(3.00019778316108,57.495,-6.12410381716742));
#37870=CARTESIAN_POINT('Ctrl Pts',(2.99717295692919,57.495,-6.17600655789209));
#37871=CARTESIAN_POINT('Ctrl Pts',(2.99327554868811,57.495,-6.22859706400148));
#37872=CARTESIAN_POINT('Ctrl Pts',(2.98850417352769,57.495,-6.28186459845047));
#37873=CARTESIAN_POINT('Ctrl Pts',(2.98286238364857,57.495,-6.33579850967689));
#37874=CARTESIAN_POINT('Ctrl Pts',(2.97635619664337,57.495,-6.39038953466561));
#37875=CARTESIAN_POINT('Ctrl Pts',(2.97046502832945,57.495,-6.43458214159149));
#37876=CARTESIAN_POINT('Ctrl Pts',(2.96566304810549,57.495,-6.46801681444607));
#37877=CARTESIAN_POINT('Ctrl Pts',(2.96229154623625,57.495,-6.49043534784131));
#37878=CARTESIAN_POINT('Ctrl Pts',(2.96056324982543,57.495,-6.50167680247051));
#37879=CARTESIAN_POINT('',(2.50394540602692,57.495,-6.69081410619341));
#37880=CARTESIAN_POINT('Origin',(6.22890783902202E-13,57.495,-1.50487931058895E-12));
#37881=CARTESIAN_POINT('',(1.66039107437148,57.495,-5.73138421404289));
#37882=CARTESIAN_POINT('Ctrl Pts',(1.66039107437148,57.495,-5.73138421404289));
#37883=CARTESIAN_POINT('Ctrl Pts',(1.66156260377487,57.495,-5.73511540682056));
#37884=CARTESIAN_POINT('Ctrl Pts',(1.66409560210805,57.495,-5.7427802739896));
#37885=CARTESIAN_POINT('Ctrl Pts',(1.6684649226766,57.495,-5.75488502996861));
#37886=CARTESIAN_POINT('Ctrl Pts',(1.67543235427329,57.495,-5.77224172513541));
#37887=CARTESIAN_POINT('Ctrl Pts',(1.68604879760674,57.495,-5.79595877235177));
#37888=CARTESIAN_POINT('Ctrl Pts',(1.69856379474191,57.495,-5.82165132013192));
#37889=CARTESIAN_POINT('Ctrl Pts',(1.71294534020683,57.495,-5.84921363316513));
#37890=CARTESIAN_POINT('Ctrl Pts',(1.7291220610224,57.495,-5.87844620539462));
#37891=CARTESIAN_POINT('Ctrl Pts',(1.74698425466387,57.495,-5.90906068827411));
#37892=CARTESIAN_POINT('Ctrl Pts',(1.76640606389864,57.495,-5.94073262861949));
#37893=CARTESIAN_POINT('Ctrl Pts',(1.78726264793636,57.495,-5.97314358084403));
#37894=CARTESIAN_POINT('Ctrl Pts',(1.80944727788364,57.495,-6.00602283509639));
#37895=CARTESIAN_POINT('Ctrl Pts',(1.83289254541003,57.495,-6.03920034699149));
#37896=CARTESIAN_POINT('Ctrl Pts',(1.85756929242873,57.495,-6.07260331771232));
#37897=CARTESIAN_POINT('Ctrl Pts',(1.88347219921808,57.495,-6.106219268893));
#37898=CARTESIAN_POINT('Ctrl Pts',(1.91060895733316,57.495,-6.14006878432982));
#37899=CARTESIAN_POINT('Ctrl Pts',(1.93898880419737,57.495,-6.17417680788945));
#37900=CARTESIAN_POINT('Ctrl Pts',(1.96860861168851,57.495,-6.20853885514981));
#37901=CARTESIAN_POINT('Ctrl Pts',(1.99945211810836,57.495,-6.24311798195985));
#37902=CARTESIAN_POINT('Ctrl Pts',(2.03149622201768,57.495,-6.27785854554194));
#37903=CARTESIAN_POINT('Ctrl Pts',(2.06471490843563,57.495,-6.31269482043467));
#37904=CARTESIAN_POINT('Ctrl Pts',(2.09908352929888,57.495,-6.34756091533115));
#37905=CARTESIAN_POINT('Ctrl Pts',(2.13458349574329,57.495,-6.38240181135703));
#37906=CARTESIAN_POINT('Ctrl Pts',(2.17120312938042,57.495,-6.41717671306138));
#37907=CARTESIAN_POINT('Ctrl Pts',(2.20893514043555,57.495,-6.45185553518375));
#37908=CARTESIAN_POINT('Ctrl Pts',(2.24777479550457,57.495,-6.48641743997175));
#37909=CARTESIAN_POINT('Ctrl Pts',(2.2877177827968,57.495,-6.52084865967127));
#37910=CARTESIAN_POINT('Ctrl Pts',(2.3287574893542,57.495,-6.55514062276556));
#37911=CARTESIAN_POINT('Ctrl Pts',(2.37088387159981,57.495,-6.58928830924802));
#37912=CARTESIAN_POINT('Ctrl Pts',(2.41408612451229,57.495,-6.6232894242584));
#37913=CARTESIAN_POINT('Ctrl Pts',(2.4495007016118,57.495,-6.65037263123018));
#37914=CARTESIAN_POINT('Ctrl Pts',(2.47653809829358,57.495,-6.67061900235304));
#37915=CARTESIAN_POINT('Ctrl Pts',(2.49477440711619,57.495,-6.68408728750665));
#37916=CARTESIAN_POINT('Ctrl Pts',(2.50394540602692,57.495,-6.69081410619341));
#37917=CARTESIAN_POINT('',(1.4909173120086,57.495,-5.1463899549833));
#37918=CARTESIAN_POINT('',(1.44917830551339,57.495,-5.00231408838243));
#37919=CARTESIAN_POINT('',(0.592010183030743,57.495,-5.32519370006274));
#37920=CARTESIAN_POINT('Origin',(0.,57.495,0.));
#37921=CARTESIAN_POINT('',(0.659304453656786,57.495,-5.93051272372135));
#37922=CARTESIAN_POINT('',(0.659304453656786,57.495,-5.93051272372135));
#37923=CARTESIAN_POINT('',(0.247119796320915,57.495,-7.13972463098307));
#37924=CARTESIAN_POINT('Ctrl Pts',(0.659304453656786,57.495,-5.93051272372135));
#37925=CARTESIAN_POINT('Ctrl Pts',(0.659649967278209,57.495,-5.93440822125369));
#37926=CARTESIAN_POINT('Ctrl Pts',(0.660242999639131,57.495,-5.94245897164689));
#37927=CARTESIAN_POINT('Ctrl Pts',(0.660838563360811,57.495,-5.95531437453421));
#37928=CARTESIAN_POINT('Ctrl Pts',(0.661043615595394,57.495,-5.97401619058905));
#37929=CARTESIAN_POINT('Ctrl Pts',(0.660311421925919,57.495,-5.99999062205821));
#37930=CARTESIAN_POINT('Ctrl Pts',(0.658581184594064,57.495,-6.02851672315009));
#37931=CARTESIAN_POINT('Ctrl Pts',(0.655842009648654,57.495,-6.05948455921138));
#37932=CARTESIAN_POINT('Ctrl Pts',(0.652083489461663,57.495,-6.092682497423));
#37933=CARTESIAN_POINT('Ctrl Pts',(0.647296629738964,57.495,-6.12780215712609));
#37934=CARTESIAN_POINT('Ctrl Pts',(0.641473544543642,57.495,-6.16449561918681));
#37935=CARTESIAN_POINT('Ctrl Pts',(0.63460770787657,57.495,-6.2024209037432));
#37936=CARTESIAN_POINT('Ctrl Pts',(0.626694128202827,57.495,-6.24128706412512));
#37937=CARTESIAN_POINT('Ctrl Pts',(0.617730009530282,57.495,-6.28091120375433));
#37938=CARTESIAN_POINT('Ctrl Pts',(0.607714431517377,57.495,-6.32121490697708));
#37939=CARTESIAN_POINT('Ctrl Pts',(0.596647533682195,57.495,-6.36218460951721));
#37940=CARTESIAN_POINT('Ctrl Pts',(0.584530087032233,57.495,-6.40384227175349));
#37941=CARTESIAN_POINT('Ctrl Pts',(0.571363102905584,57.495,-6.4462144738227));
#37942=CARTESIAN_POINT('Ctrl Pts',(0.557147755196286,57.495,-6.48929587557851));
#37943=CARTESIAN_POINT('Ctrl Pts',(0.541884929839957,57.495,-6.53304612199338));
#37944=CARTESIAN_POINT('Ctrl Pts',(0.525574676214359,57.495,-6.57740496530586));
#37945=CARTESIAN_POINT('Ctrl Pts',(0.508215876982667,57.495,-6.62230172760518));
#37946=CARTESIAN_POINT('Ctrl Pts',(0.489806088474619,57.495,-6.66766610085612));
#37947=CARTESIAN_POINT('Ctrl Pts',(0.470341429749655,57.495,-6.71344014059646));
#37948=CARTESIAN_POINT('Ctrl Pts',(0.449817078488634,57.495,-6.75958168761835));
#37949=CARTESIAN_POINT('Ctrl Pts',(0.428228256434481,57.495,-6.80606015708944));
#37950=CARTESIAN_POINT('Ctrl Pts',(0.405571362419761,57.495,-6.85285448604147));
#37951=CARTESIAN_POINT('Ctrl Pts',(0.38184511132823,57.495,-6.89995030467732));
#37952=CARTESIAN_POINT('Ctrl Pts',(0.357052332559016,57.495,-6.94733716327859));
#37953=CARTESIAN_POINT('Ctrl Pts',(0.331200384093974,57.495,-6.99500658045334));
#37954=CARTESIAN_POINT('Ctrl Pts',(0.304298370266162,57.495,-7.04295230112448));
#37955=CARTESIAN_POINT('Ctrl Pts',(0.281943861934803,57.495,-7.0815264936406));
#37956=CARTESIAN_POINT('Ctrl Pts',(0.264712515322363,57.495,-7.1105784652929));
#37957=CARTESIAN_POINT('Ctrl Pts',(0.253018452443265,57.495,-7.13000027153814));
#37958=CARTESIAN_POINT('Ctrl Pts',(0.247119796320915,57.495,-7.13972463098307));
#37959=CARTESIAN_POINT('',(-0.247119796320921,57.495,-7.13972463098307));
#37960=CARTESIAN_POINT('Origin',(-4.16333634234633E-16,57.495,-1.6286971771251E-12));
#37961=CARTESIAN_POINT('',(-0.659304453656788,57.495,-5.93051272372135));
#37962=CARTESIAN_POINT('Ctrl Pts',(-0.659304453656788,57.495,-5.93051272372135));
#37963=CARTESIAN_POINT('Ctrl Pts',(-0.659649967278237,57.495,-5.9344082212537));
#37964=CARTESIAN_POINT('Ctrl Pts',(-0.660242999639202,57.495,-5.94245897164691));
#37965=CARTESIAN_POINT('Ctrl Pts',(-0.660838563360922,57.495,-5.95531437453424));
#37966=CARTESIAN_POINT('Ctrl Pts',(-0.661043615595512,57.495,-5.97401619058907));
#37967=CARTESIAN_POINT('Ctrl Pts',(-0.660311421925998,57.495,-5.99999062205823));
#37968=CARTESIAN_POINT('Ctrl Pts',(-0.658581184594089,57.495,-6.0285167231501));
#37969=CARTESIAN_POINT('Ctrl Pts',(-0.655842009648634,57.495,-6.05948455921138));
#37970=CARTESIAN_POINT('Ctrl Pts',(-0.65208348946162,57.495,-6.09268249742298));
#37971=CARTESIAN_POINT('Ctrl Pts',(-0.647296629738921,57.495,-6.12780215712604));
#37972=CARTESIAN_POINT('Ctrl Pts',(-0.641473544543615,57.495,-6.16449561918676));
#37973=CARTESIAN_POINT('Ctrl Pts',(-0.634607707876565,57.495,-6.20242090374318));
#37974=CARTESIAN_POINT('Ctrl Pts',(-0.626694128202842,57.495,-6.24128706412515));
#37975=CARTESIAN_POINT('Ctrl Pts',(-0.617730009530307,57.495,-6.2809112037544));
#37976=CARTESIAN_POINT('Ctrl Pts',(-0.607714431517402,57.495,-6.32121490697716));
#37977=CARTESIAN_POINT('Ctrl Pts',(-0.596647533682212,57.495,-6.36218460951727));
#37978=CARTESIAN_POINT('Ctrl Pts',(-0.584530087032238,57.495,-6.40384227175352));
#37979=CARTESIAN_POINT('Ctrl Pts',(-0.57136310290558,57.495,-6.44621447382266));
#37980=CARTESIAN_POINT('Ctrl Pts',(-0.557147755196278,57.495,-6.4892958755784));
#37981=CARTESIAN_POINT('Ctrl Pts',(-0.54188492983995,57.495,-6.53304612199323));
#37982=CARTESIAN_POINT('Ctrl Pts',(-0.525574676214357,57.495,-6.57740496530571));
#37983=CARTESIAN_POINT('Ctrl Pts',(-0.508215876982669,57.495,-6.62230172760513));
#37984=CARTESIAN_POINT('Ctrl Pts',(-0.489806088474623,57.495,-6.66766610085618));
#37985=CARTESIAN_POINT('Ctrl Pts',(-0.470341429749656,57.495,-6.71344014059664));
#37986=CARTESIAN_POINT('Ctrl Pts',(-0.44981707848863,57.495,-6.75958168761858));
#37987=CARTESIAN_POINT('Ctrl Pts',(-0.428228256434474,57.495,-6.80606015708966));
#37988=CARTESIAN_POINT('Ctrl Pts',(-0.405571362419757,57.495,-6.85285448604159));
#37989=CARTESIAN_POINT('Ctrl Pts',(-0.381845111328235,57.495,-6.89995030467727));
#37990=CARTESIAN_POINT('Ctrl Pts',(-0.357052332559036,57.495,-6.94733716327837));
#37991=CARTESIAN_POINT('Ctrl Pts',(-0.331200384094009,57.495,-6.99500658045299));
#37992=CARTESIAN_POINT('Ctrl Pts',(-0.304298370266205,57.495,-7.0429523011241));
#37993=CARTESIAN_POINT('Ctrl Pts',(-0.281943861934841,57.495,-7.0815264936403));
#37994=CARTESIAN_POINT('Ctrl Pts',(-0.264712515322388,57.495,-7.11057846529273));
#37995=CARTESIAN_POINT('Ctrl Pts',(-0.253018452443276,57.495,-7.13000027153808));
#37996=CARTESIAN_POINT('Ctrl Pts',(-0.247119796320918,57.495,-7.13972463098307));
#37997=CARTESIAN_POINT('',(-0.592010183030745,57.495,-5.32519370006274));
#37998=CARTESIAN_POINT('',(-0.575436549687219,57.495,-5.17611212951227));
#37999=CARTESIAN_POINT('',(-1.4909173120086,57.495,-5.1463899549833));
#38000=CARTESIAN_POINT('Origin',(0.,57.495,0.));
#38001=CARTESIAN_POINT('',(-1.66039107437148,57.495,-5.73138421404289));
#38002=CARTESIAN_POINT('',(-1.66039107437148,57.495,-5.73138421404289));
#38003=CARTESIAN_POINT('',(-2.50394540602692,57.495,-6.69081410619341));
#38004=CARTESIAN_POINT('Ctrl Pts',(-1.66039107437148,57.495,-5.73138421404289));
#38005=CARTESIAN_POINT('Ctrl Pts',(-1.66156260377489,57.495,-5.73511540682054));
#38006=CARTESIAN_POINT('Ctrl Pts',(-1.66409560210811,57.495,-5.74278027398956));
#38007=CARTESIAN_POINT('Ctrl Pts',(-1.66846492267669,57.495,-5.75488502996854));
#38008=CARTESIAN_POINT('Ctrl Pts',(-1.67543235427339,57.495,-5.77224172513534));
#38009=CARTESIAN_POINT('Ctrl Pts',(-1.68604879760681,57.495,-5.79595877235173));
#38010=CARTESIAN_POINT('Ctrl Pts',(-1.69856379474193,57.495,-5.8216513201319));
#38011=CARTESIAN_POINT('Ctrl Pts',(-1.71294534020681,57.495,-5.84921363316514));
#38012=CARTESIAN_POINT('Ctrl Pts',(-1.72912206102237,57.495,-5.87844620539466));
#38013=CARTESIAN_POINT('Ctrl Pts',(-1.74698425466385,57.495,-5.90906068827417));
#38014=CARTESIAN_POINT('Ctrl Pts',(-1.76640606389863,57.495,-5.94073262861954));
#38015=CARTESIAN_POINT('Ctrl Pts',(-1.78726264793637,57.495,-5.97314358084405));
#38016=CARTESIAN_POINT('Ctrl Pts',(-1.80944727788364,57.495,-6.00602283509636));
#38017=CARTESIAN_POINT('Ctrl Pts',(-1.83289254541003,57.495,-6.03920034699142));
#38018=CARTESIAN_POINT('Ctrl Pts',(-1.85756929242873,57.495,-6.07260331771224));
#38019=CARTESIAN_POINT('Ctrl Pts',(-1.88347219921807,57.495,-6.10621926889293));
#38020=CARTESIAN_POINT('Ctrl Pts',(-1.91060895733316,57.495,-6.14006878432979));
#38021=CARTESIAN_POINT('Ctrl Pts',(-1.93898880419738,57.495,-6.17417680788948));
#38022=CARTESIAN_POINT('Ctrl Pts',(-1.96860861168855,57.495,-6.20853885514991));
#38023=CARTESIAN_POINT('Ctrl Pts',(-1.99945211810842,57.495,-6.24311798195999));
#38024=CARTESIAN_POINT('Ctrl Pts',(-2.03149622201774,57.495,-6.27785854554207));
#38025=CARTESIAN_POINT('Ctrl Pts',(-2.06471490843566,57.495,-6.31269482043472));
#38026=CARTESIAN_POINT('Ctrl Pts',(-2.09908352929886,57.495,-6.34756091533109));
#38027=CARTESIAN_POINT('Ctrl Pts',(-2.13458349574322,57.495,-6.38240181135686));
#38028=CARTESIAN_POINT('Ctrl Pts',(-2.17120312938032,57.495,-6.41717671306116));
#38029=CARTESIAN_POINT('Ctrl Pts',(-2.20893514043546,57.495,-6.45185553518355));
#38030=CARTESIAN_POINT('Ctrl Pts',(-2.24777479550452,57.495,-6.48641743997165));
#38031=CARTESIAN_POINT('Ctrl Pts',(-2.28771778279682,57.495,-6.52084865967131));
#38032=CARTESIAN_POINT('Ctrl Pts',(-2.32875748935431,57.495,-6.55514062276576));
#38033=CARTESIAN_POINT('Ctrl Pts',(-2.37088387159997,57.495,-6.58928830924833));
#38034=CARTESIAN_POINT('Ctrl Pts',(-2.41408612451247,57.495,-6.62328942425873));
#38035=CARTESIAN_POINT('Ctrl Pts',(-2.44950070161195,57.495,-6.65037263123044));
#38036=CARTESIAN_POINT('Ctrl Pts',(-2.47653809829367,57.495,-6.67061900235319));
#38037=CARTESIAN_POINT('Ctrl Pts',(-2.49477440711622,57.495,-6.6840872875067));
#38038=CARTESIAN_POINT('Ctrl Pts',(-2.50394540602692,57.495,-6.69081410619341));
#38039=CARTESIAN_POINT('',(-2.96056324982543,57.495,-6.5016768024705));
#38040=CARTESIAN_POINT('Origin',(-6.23660068148933E-13,57.495,-1.50456066262064E-12));
#38041=CARTESIAN_POINT('',(-2.87862685522557,57.495,-5.22677443144495));
#38042=CARTESIAN_POINT('Ctrl Pts',(-2.87862685522557,57.495,-5.22677443144495));
#38043=CARTESIAN_POINT('Ctrl Pts',(-2.88043681055508,57.495,-5.23024117954545));
#38044=CARTESIAN_POINT('Ctrl Pts',(-2.88406558980908,57.495,-5.2374521593957));
#38045=CARTESIAN_POINT('Ctrl Pts',(-2.88953536864324,57.495,-5.24910109063627));
#38046=CARTESIAN_POINT('Ctrl Pts',(-2.8968816873652,57.495,-5.26630084561717));
#38047=CARTESIAN_POINT('Ctrl Pts',(-2.90614521320845,57.495,-5.29057828960674));
#38048=CARTESIAN_POINT('Ctrl Pts',(-2.91546314862894,57.495,-5.31759510370885));
#38049=CARTESIAN_POINT('Ctrl Pts',(-2.92478335875772,57.495,-5.34725389048201));
#38050=CARTESIAN_POINT('Ctrl Pts',(-2.93401523982666,57.495,-5.37936310952307));
#38051=CARTESIAN_POINT('Ctrl Pts',(-2.94303247002252,57.495,-5.41364129622042));
#38052=CARTESIAN_POINT('Ctrl Pts',(-2.95169462080126,57.495,-5.44977003302479));
#38053=CARTESIAN_POINT('Ctrl Pts',(-2.95986479289848,57.495,-5.48743586913294));
#38054=CARTESIAN_POINT('Ctrl Pts',(-2.96742703426686,57.495,-5.52637191504897));
#38055=CARTESIAN_POINT('Ctrl Pts',(-2.97430877025613,57.495,-5.56641026634754));
#38056=CARTESIAN_POINT('Ctrl Pts',(-2.98047914221005,57.495,-5.60747882861056));
#38057=CARTESIAN_POINT('Ctrl Pts',(-2.98593308820275,57.495,-5.64956501668965));
#38058=CARTESIAN_POINT('Ctrl Pts',(-2.99067972442542,57.495,-5.6926888242775));
#38059=CARTESIAN_POINT('Ctrl Pts',(-2.99473015701058,57.495,-5.7368744211961));
#38060=CARTESIAN_POINT('Ctrl Pts',(-2.99808342690941,57.495,-5.78211642456377));
#38061=CARTESIAN_POINT('Ctrl Pts',(-3.00072490941925,57.495,-5.82837721216372));
#38062=CARTESIAN_POINT('Ctrl Pts',(-3.00263159433907,57.495,-5.87560110342618));
#38063=CARTESIAN_POINT('Ctrl Pts',(-3.00377540211876,57.495,-5.92372322806235));
#38064=CARTESIAN_POINT('Ctrl Pts',(-3.00412716938111,57.495,-5.97267956506957));
#38065=CARTESIAN_POINT('Ctrl Pts',(-3.00366113621889,57.495,-6.02241806591683));
#38066=CARTESIAN_POINT('Ctrl Pts',(-3.00235671375975,57.495,-6.07290162599645));
#38067=CARTESIAN_POINT('Ctrl Pts',(-3.00019778316116,57.495,-6.12410381716763));
#38068=CARTESIAN_POINT('Ctrl Pts',(-2.99717295692923,57.495,-6.1760065578922));
#38069=CARTESIAN_POINT('Ctrl Pts',(-2.9932755486881,57.495,-6.22859706400143));
#38070=CARTESIAN_POINT('Ctrl Pts',(-2.98850417352762,57.495,-6.28186459845025));
#38071=CARTESIAN_POINT('Ctrl Pts',(-2.98286238364847,57.495,-6.33579850967655));
#38072=CARTESIAN_POINT('Ctrl Pts',(-2.97635619664327,57.495,-6.39038953466525));
#38073=CARTESIAN_POINT('Ctrl Pts',(-2.97046502832937,57.495,-6.43458214159119));
#38074=CARTESIAN_POINT('Ctrl Pts',(-2.96566304810545,57.495,-6.4680168144459));
#38075=CARTESIAN_POINT('Ctrl Pts',(-2.96229154623624,57.495,-6.49043534784125));
#38076=CARTESIAN_POINT('Ctrl Pts',(-2.96056324982543,57.495,-6.5016768024705));
#38077=CARTESIAN_POINT('',(-2.58480949428933,57.495,-4.69328497730872));
#38078=CARTESIAN_POINT('',(-2.51244640654327,57.495,-4.56189402049717));
#38079=CARTESIAN_POINT('',(-3.34686616149372,57.495,-4.18409499139877));
#38080=CARTESIAN_POINT('Origin',(0.,57.495,0.));
#38081=CARTESIAN_POINT('',(-3.72730711280926,57.495,-4.65970441290367));
#38082=CARTESIAN_POINT('',(-3.72730711280926,57.495,-4.65970441290367));
#38083=CARTESIAN_POINT('',(-4.87380761862879,57.495,-5.22328778611671));
#38084=CARTESIAN_POINT('Ctrl Pts',(-3.72730711280926,57.495,-4.65970441290367));
#38085=CARTESIAN_POINT('Ctrl Pts',(-3.72981733050578,57.495,-4.66270326064959));
#38086=CARTESIAN_POINT('Ctrl Pts',(-3.73509073349858,57.495,-4.66881533805013));
#38087=CARTESIAN_POINT('Ctrl Pts',(-3.74375974890886,57.495,-4.67832660775287));
#38088=CARTESIAN_POINT('Ctrl Pts',(-3.75683893603616,57.495,-4.69169578253132));
#38089=CARTESIAN_POINT('Ctrl Pts',(-3.77572337177431,57.495,-4.7095447400518));
#38090=CARTESIAN_POINT('Ctrl Pts',(-3.7971178338476,57.495,-4.72849227702427));
#38091=CARTESIAN_POINT('Ctrl Pts',(-3.82095228990397,57.495,-4.74845295472312));
#38092=CARTESIAN_POINT('Ctrl Pts',(-3.84708445224627,57.495,-4.76926976684252));
#38093=CARTESIAN_POINT('Ctrl Pts',(-3.8753026227458,57.495,-4.79071829540103));
#38094=CARTESIAN_POINT('Ctrl Pts',(-3.90536636162318,57.495,-4.81254694822034));
#38095=CARTESIAN_POINT('Ctrl Pts',(-3.93703846717724,57.495,-4.83450929444279));
#38096=CARTESIAN_POINT('Ctrl Pts',(-3.97011673859274,57.495,-4.85639607415676));
#38097=CARTESIAN_POINT('Ctrl Pts',(-4.00447382552396,57.495,-4.87807598288654));
#38098=CARTESIAN_POINT('Ctrl Pts',(-4.04005493051012,57.495,-4.89949292161185));
#38099=CARTESIAN_POINT('Ctrl Pts',(-4.07685036350539,57.495,-4.92063739759521));
#38100=CARTESIAN_POINT('Ctrl Pts',(-4.11487510765791,57.495,-4.94152548435402));
#38101=CARTESIAN_POINT('Ctrl Pts',(-4.15414724283858,57.495,-4.96217669200723));
#38102=CARTESIAN_POINT('Ctrl Pts',(-4.1946621629253,57.495,-4.98258807456961));
#38103=CARTESIAN_POINT('Ctrl Pts',(-4.23639070615337,57.495,-5.00273172317863));
#38104=CARTESIAN_POINT('Ctrl Pts',(-4.27929023600674,57.495,-5.02256507114894));
#38105=CARTESIAN_POINT('Ctrl Pts',(-4.3233115657319,57.495,-5.04203735157413));
#38106=CARTESIAN_POINT('Ctrl Pts',(-4.36840670797617,57.495,-5.06109712122989));
#38107=CARTESIAN_POINT('Ctrl Pts',(-4.41453743405677,57.495,-5.07970066295468));
#38108=CARTESIAN_POINT('Ctrl Pts',(-4.4616773428065,57.495,-5.09781475579217));
#38109=CARTESIAN_POINT('Ctrl Pts',(-4.50980818622101,57.495,-5.11541439426204));
#38110=CARTESIAN_POINT('Ctrl Pts',(-4.5589176169425,57.495,-5.13248213818666));
#38111=CARTESIAN_POINT('Ctrl Pts',(-4.60899638270439,57.495,-5.14900691787064));
#38112=CARTESIAN_POINT('Ctrl Pts',(-4.66003509375265,57.495,-5.16498334493456));
#38113=CARTESIAN_POINT('Ctrl Pts',(-4.71202254995864,57.495,-5.18041062500752));
#38114=CARTESIAN_POINT('Ctrl Pts',(-4.7649478905793,57.495,-5.19529077281773));
#38115=CARTESIAN_POINT('Ctrl Pts',(-4.80803098811744,57.495,-5.20675982149348));
#38116=CARTESIAN_POINT('Ctrl Pts',(-4.84075823631825,57.495,-5.21511826561704));
#38117=CARTESIAN_POINT('Ctrl Pts',(-4.86276047837859,57.495,-5.2205826053545));
#38118=CARTESIAN_POINT('Ctrl Pts',(-4.87380761862879,57.495,-5.22328778611671));
#38119=CARTESIAN_POINT('',(-5.22328778611671,57.495,-4.87380761862879));
#38120=CARTESIAN_POINT('Origin',(-1.15195721078055E-12,57.495,-1.15136842610855E-12));
#38121=CARTESIAN_POINT('',(-4.65970441290367,57.495,-3.72730711280926));
#38122=CARTESIAN_POINT('Ctrl Pts',(-4.65970441290367,57.495,-3.72730711280926));
#38123=CARTESIAN_POINT('Ctrl Pts',(-4.66270326064961,57.495,-3.72981733050576));
#38124=CARTESIAN_POINT('Ctrl Pts',(-4.6688153380502,57.495,-3.73509073349854));
#38125=CARTESIAN_POINT('Ctrl Pts',(-4.67832660775297,57.495,-3.7437597489088));
#38126=CARTESIAN_POINT('Ctrl Pts',(-4.69169578253142,57.495,-3.7568389360361));
#38127=CARTESIAN_POINT('Ctrl Pts',(-4.70954474005187,57.495,-3.77572337177426));
#38128=CARTESIAN_POINT('Ctrl Pts',(-4.72849227702429,57.495,-3.79711783384759));
#38129=CARTESIAN_POINT('Ctrl Pts',(-4.74845295472311,57.495,-3.82095228990398));
#38130=CARTESIAN_POINT('Ctrl Pts',(-4.76926976684248,57.495,-3.84708445224628));
#38131=CARTESIAN_POINT('Ctrl Pts',(-4.79071829540097,57.495,-3.87530262274579));
#38132=CARTESIAN_POINT('Ctrl Pts',(-4.81254694822028,57.495,-3.90536636162316));
#38133=CARTESIAN_POINT('Ctrl Pts',(-4.83450929444277,57.495,-3.93703846717723));
#38134=CARTESIAN_POINT('Ctrl Pts',(-4.85639607415679,57.495,-3.97011673859275));
#38135=CARTESIAN_POINT('Ctrl Pts',(-4.8780759828866,57.495,-4.00447382552398));
#38136=CARTESIAN_POINT('Ctrl Pts',(-4.89949292161193,57.495,-4.04005493051016));
#38137=CARTESIAN_POINT('Ctrl Pts',(-4.92063739759527,57.495,-4.07685036350543));
#38138=CARTESIAN_POINT('Ctrl Pts',(-4.94152548435404,57.495,-4.11487510765792));
#38139=CARTESIAN_POINT('Ctrl Pts',(-4.9621766920072,57.495,-4.15414724283855));
#38140=CARTESIAN_POINT('Ctrl Pts',(-4.98258807456953,57.495,-4.19466216292523));
#38141=CARTESIAN_POINT('Ctrl Pts',(-5.00273172317852,57.495,-4.23639070615327));
#38142=CARTESIAN_POINT('Ctrl Pts',(-5.02256507114883,57.495,-4.27929023600664));
#38143=CARTESIAN_POINT('Ctrl Pts',(-5.04203735157409,57.495,-4.32331156573186));
#38144=CARTESIAN_POINT('Ctrl Pts',(-5.06109712122993,57.495,-4.36840670797621));
#38145=CARTESIAN_POINT('Ctrl Pts',(-5.07970066295481,57.495,-4.41453743405689));
#38146=CARTESIAN_POINT('Ctrl Pts',(-5.09781475579234,57.495,-4.46167734280668));
#38147=CARTESIAN_POINT('Ctrl Pts',(-5.11541439426219,57.495,-4.50980818622117));
#38148=CARTESIAN_POINT('Ctrl Pts',(-5.13248213818673,57.495,-4.55891761694258));
#38149=CARTESIAN_POINT('Ctrl Pts',(-5.14900691787061,57.495,-4.60899638270436));
#38150=CARTESIAN_POINT('Ctrl Pts',(-5.16498334493441,57.495,-4.66003509375248));
#38151=CARTESIAN_POINT('Ctrl Pts',(-5.1804106250073,57.495,-4.71202254995837));
#38152=CARTESIAN_POINT('Ctrl Pts',(-5.1952907728175,57.495,-4.764947890579));
#38153=CARTESIAN_POINT('Ctrl Pts',(-5.2067598214933,57.495,-4.8080309881172));
#38154=CARTESIAN_POINT('Ctrl Pts',(-5.21511826561693,57.495,-4.84075823631811));
#38155=CARTESIAN_POINT('Ctrl Pts',(-5.22058260535447,57.495,-4.86276047837853));
#38156=CARTESIAN_POINT('Ctrl Pts',(-5.22328778611671,57.495,-4.87380761862879));
#38157=CARTESIAN_POINT('',(-4.18409499139877,57.495,-3.34686616149372));
#38158=CARTESIAN_POINT('',(-4.06695907338649,57.495,-3.25316890053365));
#38159=CARTESIAN_POINT('',(-4.69328497730872,57.495,-2.58480949428933));
#38160=CARTESIAN_POINT('Origin',(0.,57.495,0.));
#38161=CARTESIAN_POINT('',(-5.22677443144495,57.495,-2.87862685522556));
#38162=CARTESIAN_POINT('',(-5.22677443144495,57.495,-2.87862685522556));
#38163=CARTESIAN_POINT('',(-6.50167680247051,57.495,-2.96056324982543));
#38164=CARTESIAN_POINT('Ctrl Pts',(-5.22677443144495,57.495,-2.87862685522556));
#38165=CARTESIAN_POINT('Ctrl Pts',(-5.23024117954545,57.495,-2.88043681055505));
#38166=CARTESIAN_POINT('Ctrl Pts',(-5.23745215939571,57.495,-2.884065589809));
#38167=CARTESIAN_POINT('Ctrl Pts',(-5.24910109063628,57.495,-2.88953536864313));
#38168=CARTESIAN_POINT('Ctrl Pts',(-5.26630084561719,57.495,-2.89688168736508));
#38169=CARTESIAN_POINT('Ctrl Pts',(-5.29057828960676,57.495,-2.90614521320837));
#38170=CARTESIAN_POINT('Ctrl Pts',(-5.31759510370885,57.495,-2.91546314862891));
#38171=CARTESIAN_POINT('Ctrl Pts',(-5.34725389048201,57.495,-2.92478335875774));
#38172=CARTESIAN_POINT('Ctrl Pts',(-5.37936310952307,57.495,-2.93401523982671));
#38173=CARTESIAN_POINT('Ctrl Pts',(-5.41364129622045,57.495,-2.94303247002258));
#38174=CARTESIAN_POINT('Ctrl Pts',(-5.44977003302482,57.495,-2.95169462080131));
#38175=CARTESIAN_POINT('Ctrl Pts',(-5.48743586913296,57.495,-2.9598647928985));
#38176=CARTESIAN_POINT('Ctrl Pts',(-5.52637191504895,57.495,-2.96742703426683));
#38177=CARTESIAN_POINT('Ctrl Pts',(-5.56641026634749,57.495,-2.97430877025609));
#38178=CARTESIAN_POINT('Ctrl Pts',(-5.6074788286105,57.495,-2.98047914221));
#38179=CARTESIAN_POINT('Ctrl Pts',(-5.64956501668959,57.495,-2.98593308820271));
#38180=CARTESIAN_POINT('Ctrl Pts',(-5.69268882427748,57.495,-2.9906797244254));
#38181=CARTESIAN_POINT('Ctrl Pts',(-5.73687442119613,57.495,-2.9947301570106));
#38182=CARTESIAN_POINT('Ctrl Pts',(-5.78211642456387,57.495,-2.99808342690946));
#38183=CARTESIAN_POINT('Ctrl Pts',(-5.82837721216385,57.495,-3.00072490941932));
#38184=CARTESIAN_POINT('Ctrl Pts',(-5.87560110342631,57.495,-3.00263159433912));
#38185=CARTESIAN_POINT('Ctrl Pts',(-5.9237232280624,57.495,-3.00377540211877));
#38186=CARTESIAN_POINT('Ctrl Pts',(-5.97267956506952,57.495,-3.00412716938109));
#38187=CARTESIAN_POINT('Ctrl Pts',(-6.02241806591666,57.495,-3.00366113621883));
#38188=CARTESIAN_POINT('Ctrl Pts',(-6.07290162599622,57.495,-3.00235671375967));
#38189=CARTESIAN_POINT('Ctrl Pts',(-6.12410381716742,57.495,-3.00019778316108));
#38190=CARTESIAN_POINT('Ctrl Pts',(-6.17600655789209,57.495,-2.99717295692919));
#38191=CARTESIAN_POINT('Ctrl Pts',(-6.22859706400147,57.495,-2.99327554868811));
#38192=CARTESIAN_POINT('Ctrl Pts',(-6.28186459845047,57.495,-2.98850417352769));
#38193=CARTESIAN_POINT('Ctrl Pts',(-6.33579850967689,57.495,-2.98286238364857));
#38194=CARTESIAN_POINT('Ctrl Pts',(-6.39038953466561,57.495,-2.97635619664337));
#38195=CARTESIAN_POINT('Ctrl Pts',(-6.43458214159149,57.495,-2.97046502832945));
#38196=CARTESIAN_POINT('Ctrl Pts',(-6.46801681444607,57.495,-2.96566304810549));
#38197=CARTESIAN_POINT('Ctrl Pts',(-6.49043534784131,57.495,-2.96229154623625));
#38198=CARTESIAN_POINT('Ctrl Pts',(-6.50167680247051,57.495,-2.96056324982543));
#38199=CARTESIAN_POINT('',(-6.69081410619341,57.495,-2.50394540602692));
#38200=CARTESIAN_POINT('Origin',(-1.50487931058895E-12,57.495,-6.22890783902202E-13));
#38201=CARTESIAN_POINT('',(-5.73138421404289,57.495,-1.66039107437148));
#38202=CARTESIAN_POINT('Ctrl Pts',(-5.73138421404289,57.495,-1.66039107437148));
#38203=CARTESIAN_POINT('Ctrl Pts',(-5.73511540682056,57.495,-1.66156260377487));
#38204=CARTESIAN_POINT('Ctrl Pts',(-5.7427802739896,57.495,-1.66409560210805));
#38205=CARTESIAN_POINT('Ctrl Pts',(-5.75488502996861,57.495,-1.6684649226766));
#38206=CARTESIAN_POINT('Ctrl Pts',(-5.77224172513541,57.495,-1.67543235427329));
#38207=CARTESIAN_POINT('Ctrl Pts',(-5.79595877235177,57.495,-1.68604879760674));
#38208=CARTESIAN_POINT('Ctrl Pts',(-5.82165132013192,57.495,-1.69856379474191));
#38209=CARTESIAN_POINT('Ctrl Pts',(-5.84921363316513,57.495,-1.71294534020683));
#38210=CARTESIAN_POINT('Ctrl Pts',(-5.87844620539462,57.495,-1.7291220610224));
#38211=CARTESIAN_POINT('Ctrl Pts',(-5.90906068827411,57.495,-1.74698425466387));
#38212=CARTESIAN_POINT('Ctrl Pts',(-5.94073262861949,57.495,-1.76640606389864));
#38213=CARTESIAN_POINT('Ctrl Pts',(-5.97314358084403,57.495,-1.78726264793636));
#38214=CARTESIAN_POINT('Ctrl Pts',(-6.00602283509639,57.495,-1.80944727788364));
#38215=CARTESIAN_POINT('Ctrl Pts',(-6.03920034699149,57.495,-1.83289254541003));
#38216=CARTESIAN_POINT('Ctrl Pts',(-6.07260331771232,57.495,-1.85756929242873));
#38217=CARTESIAN_POINT('Ctrl Pts',(-6.10621926889299,57.495,-1.88347219921808));
#38218=CARTESIAN_POINT('Ctrl Pts',(-6.14006878432982,57.495,-1.91060895733317));
#38219=CARTESIAN_POINT('Ctrl Pts',(-6.17417680788945,57.495,-1.93898880419737));
#38220=CARTESIAN_POINT('Ctrl Pts',(-6.20853885514981,57.495,-1.96860861168851));
#38221=CARTESIAN_POINT('Ctrl Pts',(-6.24311798195985,57.495,-1.99945211810837));
#38222=CARTESIAN_POINT('Ctrl Pts',(-6.27785854554194,57.495,-2.03149622201768));
#38223=CARTESIAN_POINT('Ctrl Pts',(-6.31269482043467,57.495,-2.06471490843563));
#38224=CARTESIAN_POINT('Ctrl Pts',(-6.34756091533115,57.495,-2.09908352929888));
#38225=CARTESIAN_POINT('Ctrl Pts',(-6.38240181135703,57.495,-2.13458349574329));
#38226=CARTESIAN_POINT('Ctrl Pts',(-6.41717671306138,57.495,-2.17120312938042));
#38227=CARTESIAN_POINT('Ctrl Pts',(-6.45185553518375,57.495,-2.20893514043555));
#38228=CARTESIAN_POINT('Ctrl Pts',(-6.48641743997175,57.495,-2.24777479550457));
#38229=CARTESIAN_POINT('Ctrl Pts',(-6.52084865967127,57.495,-2.2877177827968));
#38230=CARTESIAN_POINT('Ctrl Pts',(-6.55514062276556,57.495,-2.32875748935421));
#38231=CARTESIAN_POINT('Ctrl Pts',(-6.58928830924802,57.495,-2.37088387159981));
#38232=CARTESIAN_POINT('Ctrl Pts',(-6.6232894242584,57.495,-2.41408612451229));
#38233=CARTESIAN_POINT('Ctrl Pts',(-6.65037263123018,57.495,-2.4495007016118));
#38234=CARTESIAN_POINT('Ctrl Pts',(-6.67061900235304,57.495,-2.47653809829358));
#38235=CARTESIAN_POINT('Ctrl Pts',(-6.68408728750664,57.495,-2.49477440711619));
#38236=CARTESIAN_POINT('Ctrl Pts',(-6.69081410619341,57.495,-2.50394540602692));
#38237=CARTESIAN_POINT('',(-5.1463899549833,57.495,-1.4909173120086));
#38238=CARTESIAN_POINT('',(-5.00231408838243,57.495,-1.44917830551339));
#38239=CARTESIAN_POINT('',(-5.32519370006274,57.495,-0.592010183030743));
#38240=CARTESIAN_POINT('Origin',(0.,57.495,0.));
#38241=CARTESIAN_POINT('',(-5.93051272372135,57.495,-0.659304453656786));
#38242=CARTESIAN_POINT('',(-5.93051272372135,57.495,-0.659304453656786));
#38243=CARTESIAN_POINT('',(-7.13972463098307,57.495,-0.247119796320916));
#38244=CARTESIAN_POINT('Ctrl Pts',(-5.93051272372135,57.495,-0.659304453656786));
#38245=CARTESIAN_POINT('Ctrl Pts',(-5.93440822125369,57.495,-0.659649967278209));
#38246=CARTESIAN_POINT('Ctrl Pts',(-5.94245897164689,57.495,-0.660242999639131));
#38247=CARTESIAN_POINT('Ctrl Pts',(-5.95531437453421,57.495,-0.660838563360812));
#38248=CARTESIAN_POINT('Ctrl Pts',(-5.97401619058905,57.495,-0.661043615595395));
#38249=CARTESIAN_POINT('Ctrl Pts',(-5.99999062205821,57.495,-0.660311421925919));
#38250=CARTESIAN_POINT('Ctrl Pts',(-6.02851672315009,57.495,-0.658581184594065));
#38251=CARTESIAN_POINT('Ctrl Pts',(-6.05948455921138,57.495,-0.655842009648654));
#38252=CARTESIAN_POINT('Ctrl Pts',(-6.092682497423,57.495,-0.652083489461663));
#38253=CARTESIAN_POINT('Ctrl Pts',(-6.12780215712609,57.495,-0.647296629738964));
#38254=CARTESIAN_POINT('Ctrl Pts',(-6.16449561918681,57.495,-0.641473544543642));
#38255=CARTESIAN_POINT('Ctrl Pts',(-6.2024209037432,57.495,-0.63460770787657));
#38256=CARTESIAN_POINT('Ctrl Pts',(-6.24128706412512,57.495,-0.626694128202827));
#38257=CARTESIAN_POINT('Ctrl Pts',(-6.28091120375433,57.495,-0.617730009530283));
#38258=CARTESIAN_POINT('Ctrl Pts',(-6.32121490697708,57.495,-0.607714431517378));
#38259=CARTESIAN_POINT('Ctrl Pts',(-6.36218460951721,57.495,-0.596647533682195));
#38260=CARTESIAN_POINT('Ctrl Pts',(-6.40384227175349,57.495,-0.584530087032233));
#38261=CARTESIAN_POINT('Ctrl Pts',(-6.4462144738227,57.495,-0.571363102905585));
#38262=CARTESIAN_POINT('Ctrl Pts',(-6.48929587557851,57.495,-0.557147755196287));
#38263=CARTESIAN_POINT('Ctrl Pts',(-6.53304612199338,57.495,-0.541884929839958));
#38264=CARTESIAN_POINT('Ctrl Pts',(-6.57740496530586,57.495,-0.52557467621436));
#38265=CARTESIAN_POINT('Ctrl Pts',(-6.62230172760518,57.495,-0.508215876982667));
#38266=CARTESIAN_POINT('Ctrl Pts',(-6.66766610085612,57.495,-0.48980608847462));
#38267=CARTESIAN_POINT('Ctrl Pts',(-6.71344014059646,57.495,-0.470341429749656));
#38268=CARTESIAN_POINT('Ctrl Pts',(-6.75958168761835,57.495,-0.449817078488634));
#38269=CARTESIAN_POINT('Ctrl Pts',(-6.80606015708944,57.495,-0.428228256434481));
#38270=CARTESIAN_POINT('Ctrl Pts',(-6.85285448604147,57.495,-0.405571362419762));
#38271=CARTESIAN_POINT('Ctrl Pts',(-6.89995030467732,57.495,-0.381845111328231));
#38272=CARTESIAN_POINT('Ctrl Pts',(-6.94733716327859,57.495,-0.357052332559016));
#38273=CARTESIAN_POINT('Ctrl Pts',(-6.99500658045334,57.495,-0.331200384093975));
#38274=CARTESIAN_POINT('Ctrl Pts',(-7.04295230112448,57.495,-0.304298370266162));
#38275=CARTESIAN_POINT('Ctrl Pts',(-7.0815264936406,57.495,-0.281943861934803));
#38276=CARTESIAN_POINT('Ctrl Pts',(-7.1105784652929,57.495,-0.264712515322364));
#38277=CARTESIAN_POINT('Ctrl Pts',(-7.13000027153814,57.495,-0.253018452443266));
#38278=CARTESIAN_POINT('Ctrl Pts',(-7.13972463098307,57.495,-0.247119796320916));
#38279=CARTESIAN_POINT('',(-7.13972463098307,57.495,0.24711979632092));
#38280=CARTESIAN_POINT('Origin',(-1.6286971771251E-12,57.495,4.16333634234533E-16));
#38281=CARTESIAN_POINT('',(-5.93051272372135,57.495,0.659304453656788));
#38282=CARTESIAN_POINT('Ctrl Pts',(-5.93051272372135,57.495,0.659304453656788));
#38283=CARTESIAN_POINT('Ctrl Pts',(-5.9344082212537,57.495,0.659649967278237));
#38284=CARTESIAN_POINT('Ctrl Pts',(-5.94245897164691,57.495,0.660242999639201));
#38285=CARTESIAN_POINT('Ctrl Pts',(-5.95531437453424,57.495,0.660838563360922));
#38286=CARTESIAN_POINT('Ctrl Pts',(-5.97401619058907,57.495,0.661043615595512));
#38287=CARTESIAN_POINT('Ctrl Pts',(-5.99999062205823,57.495,0.660311421925997));
#38288=CARTESIAN_POINT('Ctrl Pts',(-6.0285167231501,57.495,0.658581184594089));
#38289=CARTESIAN_POINT('Ctrl Pts',(-6.05948455921138,57.495,0.655842009648634));
#38290=CARTESIAN_POINT('Ctrl Pts',(-6.09268249742298,57.495,0.65208348946162));
#38291=CARTESIAN_POINT('Ctrl Pts',(-6.12780215712604,57.495,0.64729662973892));
#38292=CARTESIAN_POINT('Ctrl Pts',(-6.16449561918676,57.495,0.641473544543615));
#38293=CARTESIAN_POINT('Ctrl Pts',(-6.20242090374318,57.495,0.634607707876565));
#38294=CARTESIAN_POINT('Ctrl Pts',(-6.24128706412515,57.495,0.626694128202842));
#38295=CARTESIAN_POINT('Ctrl Pts',(-6.2809112037544,57.495,0.617730009530307));
#38296=CARTESIAN_POINT('Ctrl Pts',(-6.32121490697716,57.495,0.607714431517402));
#38297=CARTESIAN_POINT('Ctrl Pts',(-6.36218460951727,57.495,0.596647533682211));
#38298=CARTESIAN_POINT('Ctrl Pts',(-6.40384227175352,57.495,0.584530087032238));
#38299=CARTESIAN_POINT('Ctrl Pts',(-6.44621447382266,57.495,0.57136310290558));
#38300=CARTESIAN_POINT('Ctrl Pts',(-6.4892958755784,57.495,0.557147755196277));
#38301=CARTESIAN_POINT('Ctrl Pts',(-6.53304612199323,57.495,0.54188492983995));
#38302=CARTESIAN_POINT('Ctrl Pts',(-6.57740496530571,57.495,0.525574676214356));
#38303=CARTESIAN_POINT('Ctrl Pts',(-6.62230172760513,57.495,0.508215876982669));
#38304=CARTESIAN_POINT('Ctrl Pts',(-6.66766610085618,57.495,0.489806088474623));
#38305=CARTESIAN_POINT('Ctrl Pts',(-6.71344014059664,57.495,0.470341429749656));
#38306=CARTESIAN_POINT('Ctrl Pts',(-6.75958168761858,57.495,0.449817078488629));
#38307=CARTESIAN_POINT('Ctrl Pts',(-6.80606015708966,57.495,0.428228256434473));
#38308=CARTESIAN_POINT('Ctrl Pts',(-6.85285448604159,57.495,0.405571362419756));
#38309=CARTESIAN_POINT('Ctrl Pts',(-6.89995030467727,57.495,0.381845111328235));
#38310=CARTESIAN_POINT('Ctrl Pts',(-6.94733716327837,57.495,0.357052332559036));
#38311=CARTESIAN_POINT('Ctrl Pts',(-6.99500658045299,57.495,0.331200384094009));
#38312=CARTESIAN_POINT('Ctrl Pts',(-7.0429523011241,57.495,0.304298370266205));
#38313=CARTESIAN_POINT('Ctrl Pts',(-7.0815264936403,57.495,0.28194386193484));
#38314=CARTESIAN_POINT('Ctrl Pts',(-7.11057846529273,57.495,0.264712515322387));
#38315=CARTESIAN_POINT('Ctrl Pts',(-7.13000027153808,57.495,0.253018452443276));
#38316=CARTESIAN_POINT('Ctrl Pts',(-7.13972463098307,57.495,0.247119796320917));
#38317=CARTESIAN_POINT('',(-5.32519370006274,57.495,0.592010183030744));
#38318=CARTESIAN_POINT('',(-5.17611212951227,57.495,0.575436549687218));
#38319=CARTESIAN_POINT('',(-5.1463899549833,57.495,1.4909173120086));
#38320=CARTESIAN_POINT('Origin',(0.,57.495,0.));
#38321=CARTESIAN_POINT('',(-5.73138421404289,57.495,1.66039107437148));
#38322=CARTESIAN_POINT('',(-5.73138421404289,57.495,1.66039107437148));
#38323=CARTESIAN_POINT('',(-6.69081410619341,57.495,2.50394540602692));
#38324=CARTESIAN_POINT('Ctrl Pts',(-5.73138421404289,57.495,1.66039107437148));
#38325=CARTESIAN_POINT('Ctrl Pts',(-5.73511540682054,57.495,1.66156260377489));
#38326=CARTESIAN_POINT('Ctrl Pts',(-5.74278027398956,57.495,1.6640956021081));
#38327=CARTESIAN_POINT('Ctrl Pts',(-5.75488502996854,57.495,1.66846492267669));
#38328=CARTESIAN_POINT('Ctrl Pts',(-5.77224172513534,57.495,1.67543235427339));
#38329=CARTESIAN_POINT('Ctrl Pts',(-5.79595877235173,57.495,1.68604879760681));
#38330=CARTESIAN_POINT('Ctrl Pts',(-5.8216513201319,57.495,1.69856379474193));
#38331=CARTESIAN_POINT('Ctrl Pts',(-5.84921363316514,57.495,1.71294534020681));
#38332=CARTESIAN_POINT('Ctrl Pts',(-5.87844620539466,57.495,1.72912206102237));
#38333=CARTESIAN_POINT('Ctrl Pts',(-5.90906068827417,57.495,1.74698425466385));
#38334=CARTESIAN_POINT('Ctrl Pts',(-5.94073262861954,57.495,1.76640606389863));
#38335=CARTESIAN_POINT('Ctrl Pts',(-5.97314358084405,57.495,1.78726264793637));
#38336=CARTESIAN_POINT('Ctrl Pts',(-6.00602283509636,57.495,1.80944727788364));
#38337=CARTESIAN_POINT('Ctrl Pts',(-6.03920034699142,57.495,1.83289254541003));
#38338=CARTESIAN_POINT('Ctrl Pts',(-6.07260331771224,57.495,1.85756929242873));
#38339=CARTESIAN_POINT('Ctrl Pts',(-6.10621926889293,57.495,1.88347219921807));
#38340=CARTESIAN_POINT('Ctrl Pts',(-6.14006878432979,57.495,1.91060895733316));
#38341=CARTESIAN_POINT('Ctrl Pts',(-6.17417680788948,57.495,1.93898880419738));
#38342=CARTESIAN_POINT('Ctrl Pts',(-6.20853885514991,57.495,1.96860861168855));
#38343=CARTESIAN_POINT('Ctrl Pts',(-6.24311798195999,57.495,1.99945211810842));
#38344=CARTESIAN_POINT('Ctrl Pts',(-6.27785854554207,57.495,2.03149622201774));
#38345=CARTESIAN_POINT('Ctrl Pts',(-6.31269482043472,57.495,2.06471490843565));
#38346=CARTESIAN_POINT('Ctrl Pts',(-6.34756091533109,57.495,2.09908352929886));
#38347=CARTESIAN_POINT('Ctrl Pts',(-6.38240181135686,57.495,2.13458349574322));
#38348=CARTESIAN_POINT('Ctrl Pts',(-6.41717671306116,57.495,2.17120312938032));
#38349=CARTESIAN_POINT('Ctrl Pts',(-6.45185553518355,57.495,2.20893514043546));
#38350=CARTESIAN_POINT('Ctrl Pts',(-6.48641743997165,57.495,2.24777479550452));
#38351=CARTESIAN_POINT('Ctrl Pts',(-6.52084865967131,57.495,2.28771778279682));
#38352=CARTESIAN_POINT('Ctrl Pts',(-6.55514062276576,57.495,2.32875748935431));
#38353=CARTESIAN_POINT('Ctrl Pts',(-6.58928830924833,57.495,2.37088387159997));
#38354=CARTESIAN_POINT('Ctrl Pts',(-6.62328942425873,57.495,2.41408612451247));
#38355=CARTESIAN_POINT('Ctrl Pts',(-6.65037263123044,57.495,2.44950070161195));
#38356=CARTESIAN_POINT('Ctrl Pts',(-6.67061900235319,57.495,2.47653809829367));
#38357=CARTESIAN_POINT('Ctrl Pts',(-6.6840872875067,57.495,2.49477440711622));
#38358=CARTESIAN_POINT('Ctrl Pts',(-6.69081410619341,57.495,2.50394540602692));
#38359=CARTESIAN_POINT('',(-6.5016768024705,57.495,2.96056324982543));
#38360=CARTESIAN_POINT('Origin',(-1.50456066262064E-12,57.495,6.23660068148933E-13));
#38361=CARTESIAN_POINT('',(-5.22677443144495,57.495,2.87862685522557));
#38362=CARTESIAN_POINT('Ctrl Pts',(-5.22677443144495,57.495,2.87862685522557));
#38363=CARTESIAN_POINT('Ctrl Pts',(-5.23024117954545,57.495,2.88043681055507));
#38364=CARTESIAN_POINT('Ctrl Pts',(-5.2374521593957,57.495,2.88406558980908));
#38365=CARTESIAN_POINT('Ctrl Pts',(-5.24910109063627,57.495,2.88953536864324));
#38366=CARTESIAN_POINT('Ctrl Pts',(-5.26630084561717,57.495,2.8968816873652));
#38367=CARTESIAN_POINT('Ctrl Pts',(-5.29057828960674,57.495,2.90614521320845));
#38368=CARTESIAN_POINT('Ctrl Pts',(-5.31759510370885,57.495,2.91546314862894));
#38369=CARTESIAN_POINT('Ctrl Pts',(-5.34725389048201,57.495,2.92478335875772));
#38370=CARTESIAN_POINT('Ctrl Pts',(-5.37936310952307,57.495,2.93401523982666));
#38371=CARTESIAN_POINT('Ctrl Pts',(-5.41364129622042,57.495,2.94303247002252));
#38372=CARTESIAN_POINT('Ctrl Pts',(-5.44977003302479,57.495,2.95169462080126));
#38373=CARTESIAN_POINT('Ctrl Pts',(-5.48743586913294,57.495,2.95986479289848));
#38374=CARTESIAN_POINT('Ctrl Pts',(-5.52637191504897,57.495,2.96742703426686));
#38375=CARTESIAN_POINT('Ctrl Pts',(-5.56641026634754,57.495,2.97430877025613));
#38376=CARTESIAN_POINT('Ctrl Pts',(-5.60747882861056,57.495,2.98047914221005));
#38377=CARTESIAN_POINT('Ctrl Pts',(-5.64956501668965,57.495,2.98593308820275));
#38378=CARTESIAN_POINT('Ctrl Pts',(-5.6926888242775,57.495,2.99067972442542));
#38379=CARTESIAN_POINT('Ctrl Pts',(-5.7368744211961,57.495,2.99473015701058));
#38380=CARTESIAN_POINT('Ctrl Pts',(-5.78211642456377,57.495,2.99808342690941));
#38381=CARTESIAN_POINT('Ctrl Pts',(-5.82837721216372,57.495,3.00072490941925));
#38382=CARTESIAN_POINT('Ctrl Pts',(-5.87560110342618,57.495,3.00263159433907));
#38383=CARTESIAN_POINT('Ctrl Pts',(-5.92372322806235,57.495,3.00377540211876));
#38384=CARTESIAN_POINT('Ctrl Pts',(-5.97267956506957,57.495,3.00412716938111));
#38385=CARTESIAN_POINT('Ctrl Pts',(-6.02241806591683,57.495,3.00366113621889));
#38386=CARTESIAN_POINT('Ctrl Pts',(-6.07290162599645,57.495,3.00235671375975));
#38387=CARTESIAN_POINT('Ctrl Pts',(-6.12410381716763,57.495,3.00019778316116));
#38388=CARTESIAN_POINT('Ctrl Pts',(-6.1760065578922,57.495,2.99717295692923));
#38389=CARTESIAN_POINT('Ctrl Pts',(-6.22859706400143,57.495,2.9932755486881));
#38390=CARTESIAN_POINT('Ctrl Pts',(-6.28186459845025,57.495,2.98850417352762));
#38391=CARTESIAN_POINT('Ctrl Pts',(-6.33579850967655,57.495,2.98286238364847));
#38392=CARTESIAN_POINT('Ctrl Pts',(-6.39038953466525,57.495,2.97635619664327));
#38393=CARTESIAN_POINT('Ctrl Pts',(-6.43458214159119,57.495,2.97046502832937));
#38394=CARTESIAN_POINT('Ctrl Pts',(-6.4680168144459,57.495,2.96566304810545));
#38395=CARTESIAN_POINT('Ctrl Pts',(-6.49043534784125,57.495,2.96229154623624));
#38396=CARTESIAN_POINT('Ctrl Pts',(-6.5016768024705,57.495,2.96056324982543));
#38397=CARTESIAN_POINT('',(-4.69328497730872,57.495,2.58480949428933));
#38398=CARTESIAN_POINT('',(-4.56189402049717,57.495,2.51244640654327));
#38399=CARTESIAN_POINT('',(-4.18409499139877,57.495,3.34686616149372));
#38400=CARTESIAN_POINT('Origin',(0.,57.495,0.));
#38401=CARTESIAN_POINT('',(-4.65970441290367,57.495,3.72730711280926));
#38402=CARTESIAN_POINT('',(-4.65970441290367,57.495,3.72730711280926));
#38403=CARTESIAN_POINT('',(-5.22328778611671,57.495,4.87380761862879));
#38404=CARTESIAN_POINT('Ctrl Pts',(-4.65970441290367,57.495,3.72730711280926));
#38405=CARTESIAN_POINT('Ctrl Pts',(-4.66270326064959,57.495,3.72981733050578));
#38406=CARTESIAN_POINT('Ctrl Pts',(-4.66881533805013,57.495,3.73509073349858));
#38407=CARTESIAN_POINT('Ctrl Pts',(-4.67832660775287,57.495,3.74375974890886));
#38408=CARTESIAN_POINT('Ctrl Pts',(-4.69169578253132,57.495,3.75683893603616));
#38409=CARTESIAN_POINT('Ctrl Pts',(-4.7095447400518,57.495,3.77572337177431));
#38410=CARTESIAN_POINT('Ctrl Pts',(-4.72849227702427,57.495,3.7971178338476));
#38411=CARTESIAN_POINT('Ctrl Pts',(-4.74845295472312,57.495,3.82095228990397));
#38412=CARTESIAN_POINT('Ctrl Pts',(-4.76926976684252,57.495,3.84708445224627));
#38413=CARTESIAN_POINT('Ctrl Pts',(-4.79071829540103,57.495,3.8753026227458));
#38414=CARTESIAN_POINT('Ctrl Pts',(-4.81254694822034,57.495,3.90536636162318));
#38415=CARTESIAN_POINT('Ctrl Pts',(-4.83450929444279,57.495,3.93703846717724));
#38416=CARTESIAN_POINT('Ctrl Pts',(-4.85639607415676,57.495,3.97011673859274));
#38417=CARTESIAN_POINT('Ctrl Pts',(-4.87807598288654,57.495,4.00447382552396));
#38418=CARTESIAN_POINT('Ctrl Pts',(-4.89949292161185,57.495,4.04005493051012));
#38419=CARTESIAN_POINT('Ctrl Pts',(-4.92063739759521,57.495,4.07685036350539));
#38420=CARTESIAN_POINT('Ctrl Pts',(-4.94152548435402,57.495,4.11487510765791));
#38421=CARTESIAN_POINT('Ctrl Pts',(-4.96217669200723,57.495,4.15414724283858));
#38422=CARTESIAN_POINT('Ctrl Pts',(-4.98258807456962,57.495,4.1946621629253));
#38423=CARTESIAN_POINT('Ctrl Pts',(-5.00273172317863,57.495,4.23639070615337));
#38424=CARTESIAN_POINT('Ctrl Pts',(-5.02256507114894,57.495,4.27929023600674));
#38425=CARTESIAN_POINT('Ctrl Pts',(-5.04203735157413,57.495,4.3233115657319));
#38426=CARTESIAN_POINT('Ctrl Pts',(-5.06109712122989,57.495,4.36840670797617));
#38427=CARTESIAN_POINT('Ctrl Pts',(-5.07970066295468,57.495,4.41453743405677));
#38428=CARTESIAN_POINT('Ctrl Pts',(-5.09781475579217,57.495,4.4616773428065));
#38429=CARTESIAN_POINT('Ctrl Pts',(-5.11541439426204,57.495,4.50980818622101));
#38430=CARTESIAN_POINT('Ctrl Pts',(-5.13248213818666,57.495,4.5589176169425));
#38431=CARTESIAN_POINT('Ctrl Pts',(-5.14900691787064,57.495,4.60899638270439));
#38432=CARTESIAN_POINT('Ctrl Pts',(-5.16498334493456,57.495,4.66003509375265));
#38433=CARTESIAN_POINT('Ctrl Pts',(-5.18041062500752,57.495,4.71202254995864));
#38434=CARTESIAN_POINT('Ctrl Pts',(-5.19529077281773,57.495,4.7649478905793));
#38435=CARTESIAN_POINT('Ctrl Pts',(-5.20675982149348,57.495,4.80803098811744));
#38436=CARTESIAN_POINT('Ctrl Pts',(-5.21511826561704,57.495,4.84075823631825));
#38437=CARTESIAN_POINT('Ctrl Pts',(-5.22058260535451,57.495,4.86276047837859));
#38438=CARTESIAN_POINT('Ctrl Pts',(-5.22328778611671,57.495,4.87380761862879));
#38439=CARTESIAN_POINT('',(-4.87380761862879,57.495,5.22328778611671));
#38440=CARTESIAN_POINT('Origin',(-1.15136842610855E-12,57.495,1.15195721078055E-12));
#38441=CARTESIAN_POINT('',(-3.72730711280926,57.495,4.65970441290367));
#38442=CARTESIAN_POINT('Ctrl Pts',(-3.72730711280926,57.495,4.65970441290367));
#38443=CARTESIAN_POINT('Ctrl Pts',(-3.72981733050576,57.495,4.66270326064961));
#38444=CARTESIAN_POINT('Ctrl Pts',(-3.73509073349854,57.495,4.6688153380502));
#38445=CARTESIAN_POINT('Ctrl Pts',(-3.7437597489088,57.495,4.67832660775297));
#38446=CARTESIAN_POINT('Ctrl Pts',(-3.7568389360361,57.495,4.69169578253142));
#38447=CARTESIAN_POINT('Ctrl Pts',(-3.77572337177426,57.495,4.70954474005187));
#38448=CARTESIAN_POINT('Ctrl Pts',(-3.79711783384759,57.495,4.72849227702429));
#38449=CARTESIAN_POINT('Ctrl Pts',(-3.82095228990398,57.495,4.74845295472311));
#38450=CARTESIAN_POINT('Ctrl Pts',(-3.84708445224628,57.495,4.76926976684248));
#38451=CARTESIAN_POINT('Ctrl Pts',(-3.87530262274579,57.495,4.79071829540097));
#38452=CARTESIAN_POINT('Ctrl Pts',(-3.90536636162316,57.495,4.81254694822028));
#38453=CARTESIAN_POINT('Ctrl Pts',(-3.93703846717723,57.495,4.83450929444277));
#38454=CARTESIAN_POINT('Ctrl Pts',(-3.97011673859275,57.495,4.85639607415679));
#38455=CARTESIAN_POINT('Ctrl Pts',(-4.00447382552398,57.495,4.8780759828866));
#38456=CARTESIAN_POINT('Ctrl Pts',(-4.04005493051016,57.495,4.89949292161193));
#38457=CARTESIAN_POINT('Ctrl Pts',(-4.07685036350543,57.495,4.92063739759527));
#38458=CARTESIAN_POINT('Ctrl Pts',(-4.11487510765792,57.495,4.94152548435404));
#38459=CARTESIAN_POINT('Ctrl Pts',(-4.15414724283855,57.495,4.9621766920072));
#38460=CARTESIAN_POINT('Ctrl Pts',(-4.19466216292523,57.495,4.98258807456953));
#38461=CARTESIAN_POINT('Ctrl Pts',(-4.23639070615327,57.495,5.00273172317852));
#38462=CARTESIAN_POINT('Ctrl Pts',(-4.27929023600664,57.495,5.02256507114883));
#38463=CARTESIAN_POINT('Ctrl Pts',(-4.32331156573186,57.495,5.04203735157409));
#38464=CARTESIAN_POINT('Ctrl Pts',(-4.36840670797621,57.495,5.06109712122993));
#38465=CARTESIAN_POINT('Ctrl Pts',(-4.41453743405689,57.495,5.07970066295481));
#38466=CARTESIAN_POINT('Ctrl Pts',(-4.46167734280668,57.495,5.09781475579234));
#38467=CARTESIAN_POINT('Ctrl Pts',(-4.50980818622117,57.495,5.11541439426219));
#38468=CARTESIAN_POINT('Ctrl Pts',(-4.55891761694258,57.495,5.13248213818673));
#38469=CARTESIAN_POINT('Ctrl Pts',(-4.60899638270436,57.495,5.14900691787061));
#38470=CARTESIAN_POINT('Ctrl Pts',(-4.66003509375248,57.495,5.16498334493441));
#38471=CARTESIAN_POINT('Ctrl Pts',(-4.71202254995837,57.495,5.1804106250073));
#38472=CARTESIAN_POINT('Ctrl Pts',(-4.764947890579,57.495,5.1952907728175));
#38473=CARTESIAN_POINT('Ctrl Pts',(-4.8080309881172,57.495,5.2067598214933));
#38474=CARTESIAN_POINT('Ctrl Pts',(-4.84075823631812,57.495,5.21511826561693));
#38475=CARTESIAN_POINT('Ctrl Pts',(-4.86276047837854,57.495,5.22058260535447));
#38476=CARTESIAN_POINT('Ctrl Pts',(-4.87380761862879,57.495,5.22328778611671));
#38477=CARTESIAN_POINT('',(-3.34686616149372,57.495,4.18409499139877));
#38478=CARTESIAN_POINT('',(-3.25316890053365,57.495,4.06695907338649));
#38479=CARTESIAN_POINT('',(-2.58480949428933,57.495,4.69328497730872));
#38480=CARTESIAN_POINT('Origin',(0.,57.495,0.));
#38481=CARTESIAN_POINT('',(-2.87862685522557,57.495,5.22677443144495));
#38482=CARTESIAN_POINT('',(-2.87862685522557,57.495,5.22677443144495));
#38483=CARTESIAN_POINT('',(-2.96056324982543,57.495,6.50167680247051));
#38484=CARTESIAN_POINT('Ctrl Pts',(-2.87862685522557,57.495,5.22677443144495));
#38485=CARTESIAN_POINT('Ctrl Pts',(-2.88043681055505,57.495,5.23024117954545));
#38486=CARTESIAN_POINT('Ctrl Pts',(-2.884065589809,57.495,5.23745215939571));
#38487=CARTESIAN_POINT('Ctrl Pts',(-2.88953536864313,57.495,5.24910109063628));
#38488=CARTESIAN_POINT('Ctrl Pts',(-2.89688168736508,57.495,5.26630084561719));
#38489=CARTESIAN_POINT('Ctrl Pts',(-2.90614521320837,57.495,5.29057828960676));
#38490=CARTESIAN_POINT('Ctrl Pts',(-2.91546314862891,57.495,5.31759510370885));
#38491=CARTESIAN_POINT('Ctrl Pts',(-2.92478335875774,57.495,5.34725389048201));
#38492=CARTESIAN_POINT('Ctrl Pts',(-2.93401523982671,57.495,5.37936310952307));
#38493=CARTESIAN_POINT('Ctrl Pts',(-2.94303247002258,57.495,5.41364129622045));
#38494=CARTESIAN_POINT('Ctrl Pts',(-2.95169462080131,57.495,5.44977003302482));
#38495=CARTESIAN_POINT('Ctrl Pts',(-2.9598647928985,57.495,5.48743586913296));
#38496=CARTESIAN_POINT('Ctrl Pts',(-2.96742703426683,57.495,5.52637191504895));
#38497=CARTESIAN_POINT('Ctrl Pts',(-2.97430877025609,57.495,5.56641026634749));
#38498=CARTESIAN_POINT('Ctrl Pts',(-2.98047914221,57.495,5.6074788286105));
#38499=CARTESIAN_POINT('Ctrl Pts',(-2.98593308820271,57.495,5.64956501668959));
#38500=CARTESIAN_POINT('Ctrl Pts',(-2.9906797244254,57.495,5.69268882427748));
#38501=CARTESIAN_POINT('Ctrl Pts',(-2.9947301570106,57.495,5.73687442119613));
#38502=CARTESIAN_POINT('Ctrl Pts',(-2.99808342690946,57.495,5.78211642456387));
#38503=CARTESIAN_POINT('Ctrl Pts',(-3.00072490941932,57.495,5.82837721216385));
#38504=CARTESIAN_POINT('Ctrl Pts',(-3.00263159433912,57.495,5.87560110342631));
#38505=CARTESIAN_POINT('Ctrl Pts',(-3.00377540211877,57.495,5.9237232280624));
#38506=CARTESIAN_POINT('Ctrl Pts',(-3.00412716938109,57.495,5.97267956506952));
#38507=CARTESIAN_POINT('Ctrl Pts',(-3.00366113621883,57.495,6.02241806591666));
#38508=CARTESIAN_POINT('Ctrl Pts',(-3.00235671375967,57.495,6.07290162599622));
#38509=CARTESIAN_POINT('Ctrl Pts',(-3.00019778316108,57.495,6.12410381716742));
#38510=CARTESIAN_POINT('Ctrl Pts',(-2.99717295692919,57.495,6.17600655789209));
#38511=CARTESIAN_POINT('Ctrl Pts',(-2.99327554868811,57.495,6.22859706400147));
#38512=CARTESIAN_POINT('Ctrl Pts',(-2.98850417352769,57.495,6.28186459845047));
#38513=CARTESIAN_POINT('Ctrl Pts',(-2.98286238364857,57.495,6.33579850967689));
#38514=CARTESIAN_POINT('Ctrl Pts',(-2.97635619664337,57.495,6.39038953466561));
#38515=CARTESIAN_POINT('Ctrl Pts',(-2.97046502832945,57.495,6.43458214159149));
#38516=CARTESIAN_POINT('Ctrl Pts',(-2.96566304810549,57.495,6.46801681444607));
#38517=CARTESIAN_POINT('Ctrl Pts',(-2.96229154623625,57.495,6.49043534784131));
#38518=CARTESIAN_POINT('Ctrl Pts',(-2.96056324982543,57.495,6.50167680247051));
#38519=CARTESIAN_POINT('',(-2.50394540602692,57.495,6.69081410619341));
#38520=CARTESIAN_POINT('Origin',(-6.22890783902202E-13,57.495,1.50487931058895E-12));
#38521=CARTESIAN_POINT('',(-1.66039107437148,57.495,5.73138421404289));
#38522=CARTESIAN_POINT('Ctrl Pts',(-1.66039107437148,57.495,5.73138421404289));
#38523=CARTESIAN_POINT('Ctrl Pts',(-1.66156260377487,57.495,5.73511540682056));
#38524=CARTESIAN_POINT('Ctrl Pts',(-1.66409560210805,57.495,5.7427802739896));
#38525=CARTESIAN_POINT('Ctrl Pts',(-1.6684649226766,57.495,5.75488502996861));
#38526=CARTESIAN_POINT('Ctrl Pts',(-1.67543235427329,57.495,5.77224172513541));
#38527=CARTESIAN_POINT('Ctrl Pts',(-1.68604879760674,57.495,5.79595877235177));
#38528=CARTESIAN_POINT('Ctrl Pts',(-1.69856379474191,57.495,5.82165132013192));
#38529=CARTESIAN_POINT('Ctrl Pts',(-1.71294534020683,57.495,5.84921363316513));
#38530=CARTESIAN_POINT('Ctrl Pts',(-1.7291220610224,57.495,5.87844620539462));
#38531=CARTESIAN_POINT('Ctrl Pts',(-1.74698425466387,57.495,5.90906068827411));
#38532=CARTESIAN_POINT('Ctrl Pts',(-1.76640606389864,57.495,5.94073262861949));
#38533=CARTESIAN_POINT('Ctrl Pts',(-1.78726264793636,57.495,5.97314358084403));
#38534=CARTESIAN_POINT('Ctrl Pts',(-1.80944727788364,57.495,6.0060228350964));
#38535=CARTESIAN_POINT('Ctrl Pts',(-1.83289254541003,57.495,6.03920034699149));
#38536=CARTESIAN_POINT('Ctrl Pts',(-1.85756929242873,57.495,6.07260331771232));
#38537=CARTESIAN_POINT('Ctrl Pts',(-1.88347219921808,57.495,6.10621926889299));
#38538=CARTESIAN_POINT('Ctrl Pts',(-1.91060895733317,57.495,6.14006878432982));
#38539=CARTESIAN_POINT('Ctrl Pts',(-1.93898880419737,57.495,6.17417680788945));
#38540=CARTESIAN_POINT('Ctrl Pts',(-1.96860861168851,57.495,6.20853885514981));
#38541=CARTESIAN_POINT('Ctrl Pts',(-1.99945211810837,57.495,6.24311798195985));
#38542=CARTESIAN_POINT('Ctrl Pts',(-2.03149622201768,57.495,6.27785854554194));
#38543=CARTESIAN_POINT('Ctrl Pts',(-2.06471490843563,57.495,6.31269482043467));
#38544=CARTESIAN_POINT('Ctrl Pts',(-2.09908352929888,57.495,6.34756091533115));
#38545=CARTESIAN_POINT('Ctrl Pts',(-2.13458349574329,57.495,6.38240181135703));
#38546=CARTESIAN_POINT('Ctrl Pts',(-2.17120312938042,57.495,6.41717671306138));
#38547=CARTESIAN_POINT('Ctrl Pts',(-2.20893514043555,57.495,6.45185553518375));
#38548=CARTESIAN_POINT('Ctrl Pts',(-2.24777479550457,57.495,6.48641743997175));
#38549=CARTESIAN_POINT('Ctrl Pts',(-2.2877177827968,57.495,6.52084865967127));
#38550=CARTESIAN_POINT('Ctrl Pts',(-2.32875748935421,57.495,6.55514062276556));
#38551=CARTESIAN_POINT('Ctrl Pts',(-2.37088387159981,57.495,6.58928830924802));
#38552=CARTESIAN_POINT('Ctrl Pts',(-2.41408612451229,57.495,6.6232894242584));
#38553=CARTESIAN_POINT('Ctrl Pts',(-2.4495007016118,57.495,6.65037263123018));
#38554=CARTESIAN_POINT('Ctrl Pts',(-2.47653809829358,57.495,6.67061900235304));
#38555=CARTESIAN_POINT('Ctrl Pts',(-2.49477440711619,57.495,6.68408728750664));
#38556=CARTESIAN_POINT('Ctrl Pts',(-2.50394540602692,57.495,6.69081410619341));
#38557=CARTESIAN_POINT('',(-1.4909173120086,57.495,5.1463899549833));
#38558=CARTESIAN_POINT('',(-1.4491783055134,57.495,5.00231408838243));
#38559=CARTESIAN_POINT('',(-0.592010183030743,57.495,5.32519370006274));
#38560=CARTESIAN_POINT('Origin',(0.,57.495,0.));
#38561=CARTESIAN_POINT('',(-0.659304453656787,57.495,5.93051272372135));
#38562=CARTESIAN_POINT('',(-0.659304453656787,57.495,5.93051272372135));
#38563=CARTESIAN_POINT('',(-0.247119796320916,57.495,7.13972463098307));
#38564=CARTESIAN_POINT('Ctrl Pts',(-0.659304453656787,57.495,5.93051272372135));
#38565=CARTESIAN_POINT('Ctrl Pts',(-0.65964996727821,57.495,5.93440822125369));
#38566=CARTESIAN_POINT('Ctrl Pts',(-0.660242999639131,57.495,5.94245897164689));
#38567=CARTESIAN_POINT('Ctrl Pts',(-0.660838563360812,57.495,5.95531437453421));
#38568=CARTESIAN_POINT('Ctrl Pts',(-0.661043615595395,57.495,5.97401619058905));
#38569=CARTESIAN_POINT('Ctrl Pts',(-0.660311421925919,57.495,5.99999062205821));
#38570=CARTESIAN_POINT('Ctrl Pts',(-0.658581184594065,57.495,6.02851672315009));
#38571=CARTESIAN_POINT('Ctrl Pts',(-0.655842009648655,57.495,6.05948455921138));
#38572=CARTESIAN_POINT('Ctrl Pts',(-0.652083489461663,57.495,6.092682497423));
#38573=CARTESIAN_POINT('Ctrl Pts',(-0.647296629738964,57.495,6.12780215712609));
#38574=CARTESIAN_POINT('Ctrl Pts',(-0.641473544543643,57.495,6.16449561918681));
#38575=CARTESIAN_POINT('Ctrl Pts',(-0.63460770787657,57.495,6.2024209037432));
#38576=CARTESIAN_POINT('Ctrl Pts',(-0.626694128202828,57.495,6.24128706412512));
#38577=CARTESIAN_POINT('Ctrl Pts',(-0.617730009530283,57.495,6.28091120375433));
#38578=CARTESIAN_POINT('Ctrl Pts',(-0.607714431517378,57.495,6.32121490697708));
#38579=CARTESIAN_POINT('Ctrl Pts',(-0.596647533682196,57.495,6.36218460951721));
#38580=CARTESIAN_POINT('Ctrl Pts',(-0.584530087032233,57.495,6.40384227175349));
#38581=CARTESIAN_POINT('Ctrl Pts',(-0.571363102905585,57.495,6.4462144738227));
#38582=CARTESIAN_POINT('Ctrl Pts',(-0.557147755196287,57.495,6.48929587557851));
#38583=CARTESIAN_POINT('Ctrl Pts',(-0.541884929839958,57.495,6.53304612199338));
#38584=CARTESIAN_POINT('Ctrl Pts',(-0.52557467621436,57.495,6.57740496530586));
#38585=CARTESIAN_POINT('Ctrl Pts',(-0.508215876982667,57.495,6.62230172760518));
#38586=CARTESIAN_POINT('Ctrl Pts',(-0.48980608847462,57.495,6.66766610085612));
#38587=CARTESIAN_POINT('Ctrl Pts',(-0.470341429749656,57.495,6.71344014059646));
#38588=CARTESIAN_POINT('Ctrl Pts',(-0.449817078488635,57.495,6.75958168761835));
#38589=CARTESIAN_POINT('Ctrl Pts',(-0.428228256434482,57.495,6.80606015708944));
#38590=CARTESIAN_POINT('Ctrl Pts',(-0.405571362419762,57.495,6.85285448604147));
#38591=CARTESIAN_POINT('Ctrl Pts',(-0.381845111328231,57.495,6.89995030467732));
#38592=CARTESIAN_POINT('Ctrl Pts',(-0.357052332559017,57.495,6.94733716327859));
#38593=CARTESIAN_POINT('Ctrl Pts',(-0.331200384093975,57.495,6.99500658045334));
#38594=CARTESIAN_POINT('Ctrl Pts',(-0.304298370266163,57.495,7.04295230112448));
#38595=CARTESIAN_POINT('Ctrl Pts',(-0.281943861934804,57.495,7.0815264936406));
#38596=CARTESIAN_POINT('Ctrl Pts',(-0.264712515322364,57.495,7.1105784652929));
#38597=CARTESIAN_POINT('Ctrl Pts',(-0.253018452443266,57.495,7.13000027153814));
#38598=CARTESIAN_POINT('Ctrl Pts',(-0.247119796320916,57.495,7.13972463098307));
#38599=CARTESIAN_POINT('',(0.24711979632092,57.495,7.13972463098307));
#38600=CARTESIAN_POINT('Origin',(4.16333634234434E-16,57.495,1.6286971771251E-12));
#38601=CARTESIAN_POINT('',(0.659304453656788,57.495,5.93051272372135));
#38602=CARTESIAN_POINT('Ctrl Pts',(0.659304453656788,57.495,5.93051272372135));
#38603=CARTESIAN_POINT('Ctrl Pts',(0.659649967278236,57.495,5.9344082212537));
#38604=CARTESIAN_POINT('Ctrl Pts',(0.660242999639201,57.495,5.94245897164691));
#38605=CARTESIAN_POINT('Ctrl Pts',(0.660838563360921,57.495,5.95531437453424));
#38606=CARTESIAN_POINT('Ctrl Pts',(0.661043615595512,57.495,5.97401619058907));
#38607=CARTESIAN_POINT('Ctrl Pts',(0.660311421925997,57.495,5.99999062205823));
#38608=CARTESIAN_POINT('Ctrl Pts',(0.658581184594088,57.495,6.0285167231501));
#38609=CARTESIAN_POINT('Ctrl Pts',(0.655842009648633,57.495,6.05948455921138));
#38610=CARTESIAN_POINT('Ctrl Pts',(0.652083489461619,57.495,6.09268249742298));
#38611=CARTESIAN_POINT('Ctrl Pts',(0.64729662973892,57.495,6.12780215712604));
#38612=CARTESIAN_POINT('Ctrl Pts',(0.641473544543614,57.495,6.16449561918676));
#38613=CARTESIAN_POINT('Ctrl Pts',(0.634607707876564,57.495,6.20242090374318));
#38614=CARTESIAN_POINT('Ctrl Pts',(0.626694128202842,57.495,6.24128706412515));
#38615=CARTESIAN_POINT('Ctrl Pts',(0.617730009530307,57.495,6.2809112037544));
#38616=CARTESIAN_POINT('Ctrl Pts',(0.607714431517401,57.495,6.32121490697716));
#38617=CARTESIAN_POINT('Ctrl Pts',(0.596647533682211,57.495,6.36218460951727));
#38618=CARTESIAN_POINT('Ctrl Pts',(0.584530087032237,57.495,6.40384227175352));
#38619=CARTESIAN_POINT('Ctrl Pts',(0.571363102905579,57.495,6.44621447382266));
#38620=CARTESIAN_POINT('Ctrl Pts',(0.557147755196277,57.495,6.4892958755784));
#38621=CARTESIAN_POINT('Ctrl Pts',(0.541884929839949,57.495,6.53304612199323));
#38622=CARTESIAN_POINT('Ctrl Pts',(0.525574676214356,57.495,6.57740496530571));
#38623=CARTESIAN_POINT('Ctrl Pts',(0.508215876982668,57.495,6.62230172760513));
#38624=CARTESIAN_POINT('Ctrl Pts',(0.489806088474622,57.495,6.66766610085618));
#38625=CARTESIAN_POINT('Ctrl Pts',(0.470341429749655,57.495,6.71344014059664));
#38626=CARTESIAN_POINT('Ctrl Pts',(0.449817078488629,57.495,6.75958168761858));
#38627=CARTESIAN_POINT('Ctrl Pts',(0.428228256434473,57.495,6.80606015708966));
#38628=CARTESIAN_POINT('Ctrl Pts',(0.405571362419756,57.495,6.85285448604159));
#38629=CARTESIAN_POINT('Ctrl Pts',(0.381845111328234,57.495,6.89995030467727));
#38630=CARTESIAN_POINT('Ctrl Pts',(0.357052332559035,57.495,6.94733716327837));
#38631=CARTESIAN_POINT('Ctrl Pts',(0.331200384094009,57.495,6.99500658045299));
#38632=CARTESIAN_POINT('Ctrl Pts',(0.304298370266204,57.495,7.0429523011241));
#38633=CARTESIAN_POINT('Ctrl Pts',(0.28194386193484,57.495,7.0815264936403));
#38634=CARTESIAN_POINT('Ctrl Pts',(0.264712515322387,57.495,7.11057846529273));
#38635=CARTESIAN_POINT('Ctrl Pts',(0.253018452443275,57.495,7.13000027153808));
#38636=CARTESIAN_POINT('Ctrl Pts',(0.247119796320917,57.495,7.13972463098307));
#38637=CARTESIAN_POINT('',(0.592010183030744,57.495,5.32519370006274));
#38638=CARTESIAN_POINT('',(0.575436549687218,57.495,5.17611212951227));
#38639=CARTESIAN_POINT('Origin',(0.,57.495,0.));
#38640=CARTESIAN_POINT('',(-4.477,57.495,-5.4827437197827E-16));
#38641=CARTESIAN_POINT('Origin',(0.,57.495,0.));
#38642=CARTESIAN_POINT('Origin',(0.,54.32,0.));
#38643=CARTESIAN_POINT('',(3.34686616149372,51.145,4.18409499139877));
#38644=CARTESIAN_POINT('Origin',(0.,51.145,0.));
#38645=CARTESIAN_POINT('',(3.34686616149372,54.32,4.18409499139877));
#38646=CARTESIAN_POINT('Origin',(3.72730711280926,57.495,4.65970441290367));
#38647=CARTESIAN_POINT('',(3.72730711280926,51.145,4.65970441290367));
#38648=CARTESIAN_POINT('',(3.72730711280926,51.145,4.65970441290367));
#38649=CARTESIAN_POINT('',(3.72730711280926,57.495,4.65970441290367));
#38650=CARTESIAN_POINT('Origin',(1.15195721078055E-12,57.495,1.15136842610855E-12));
#38651=CARTESIAN_POINT('',(4.87380761862879,51.145,5.22328778611671));
#38652=CARTESIAN_POINT('',(4.87380761862879,57.495,5.22328778611671));
#38653=CARTESIAN_POINT('',(5.22328778611671,51.145,4.87380761862879));
#38654=CARTESIAN_POINT('Origin',(1.15195721078055E-12,51.145,1.15136842610855E-12));
#38655=CARTESIAN_POINT('',(5.22328778611671,57.495,4.87380761862879));
#38656=CARTESIAN_POINT('Ctrl Pts',(4.65970441290368,57.495,3.72730711280926));
#38657=CARTESIAN_POINT('Ctrl Pts',(4.65970441290368,49.875,3.72730711280926));
#38658=CARTESIAN_POINT('Ctrl Pts',(4.66270326064961,57.495,3.72981733050576));
#38659=CARTESIAN_POINT('Ctrl Pts',(4.66270326064961,49.875,3.72981733050576));
#38660=CARTESIAN_POINT('Ctrl Pts',(4.6688153380502,57.495,3.73509073349854));
#38661=CARTESIAN_POINT('Ctrl Pts',(4.6688153380502,49.875,3.73509073349854));
#38662=CARTESIAN_POINT('Ctrl Pts',(4.67832660775297,57.495,3.7437597489088));
#38663=CARTESIAN_POINT('Ctrl Pts',(4.67832660775297,49.875,3.7437597489088));
#38664=CARTESIAN_POINT('Ctrl Pts',(4.69169578253142,57.495,3.7568389360361));
#38665=CARTESIAN_POINT('Ctrl Pts',(4.69169578253142,49.875,3.7568389360361));
#38666=CARTESIAN_POINT('Ctrl Pts',(4.70954474005187,57.495,3.77572337177426));
#38667=CARTESIAN_POINT('Ctrl Pts',(4.70954474005187,49.875,3.77572337177426));
#38668=CARTESIAN_POINT('Ctrl Pts',(4.72849227702429,57.495,3.79711783384759));
#38669=CARTESIAN_POINT('Ctrl Pts',(4.72849227702429,49.875,3.79711783384759));
#38670=CARTESIAN_POINT('Ctrl Pts',(4.74845295472311,57.495,3.82095228990398));
#38671=CARTESIAN_POINT('Ctrl Pts',(4.74845295472311,49.875,3.82095228990398));
#38672=CARTESIAN_POINT('Ctrl Pts',(4.76926976684248,57.495,3.84708445224628));
#38673=CARTESIAN_POINT('Ctrl Pts',(4.76926976684248,49.875,3.84708445224628));
#38674=CARTESIAN_POINT('Ctrl Pts',(4.79071829540097,57.495,3.87530262274579));
#38675=CARTESIAN_POINT('Ctrl Pts',(4.79071829540097,49.875,3.87530262274579));
#38676=CARTESIAN_POINT('Ctrl Pts',(4.81254694822028,57.495,3.90536636162316));
#38677=CARTESIAN_POINT('Ctrl Pts',(4.81254694822028,49.875,3.90536636162316));
#38678=CARTESIAN_POINT('Ctrl Pts',(4.83450929444277,57.495,3.93703846717723));
#38679=CARTESIAN_POINT('Ctrl Pts',(4.83450929444277,49.875,3.93703846717723));
#38680=CARTESIAN_POINT('Ctrl Pts',(4.85639607415679,57.495,3.97011673859275));
#38681=CARTESIAN_POINT('Ctrl Pts',(4.85639607415679,49.875,3.97011673859275));
#38682=CARTESIAN_POINT('Ctrl Pts',(4.87807598288661,57.495,4.00447382552398));
#38683=CARTESIAN_POINT('Ctrl Pts',(4.87807598288661,49.875,4.00447382552398));
#38684=CARTESIAN_POINT('Ctrl Pts',(4.89949292161193,57.495,4.04005493051016));
#38685=CARTESIAN_POINT('Ctrl Pts',(4.89949292161193,49.875,4.04005493051016));
#38686=CARTESIAN_POINT('Ctrl Pts',(4.92063739759527,57.495,4.07685036350543));
#38687=CARTESIAN_POINT('Ctrl Pts',(4.92063739759527,49.875,4.07685036350543));
#38688=CARTESIAN_POINT('Ctrl Pts',(4.94152548435404,57.495,4.11487510765792));
#38689=CARTESIAN_POINT('Ctrl Pts',(4.94152548435404,49.875,4.11487510765792));
#38690=CARTESIAN_POINT('Ctrl Pts',(4.9621766920072,57.495,4.15414724283855));
#38691=CARTESIAN_POINT('Ctrl Pts',(4.9621766920072,49.875,4.15414724283855));
#38692=CARTESIAN_POINT('Ctrl Pts',(4.98258807456953,57.495,4.19466216292523));
#38693=CARTESIAN_POINT('Ctrl Pts',(4.98258807456953,49.875,4.19466216292523));
#38694=CARTESIAN_POINT('Ctrl Pts',(5.00273172317852,57.495,4.23639070615327));
#38695=CARTESIAN_POINT('Ctrl Pts',(5.00273172317852,49.875,4.23639070615327));
#38696=CARTESIAN_POINT('Ctrl Pts',(5.02256507114883,57.495,4.27929023600664));
#38697=CARTESIAN_POINT('Ctrl Pts',(5.02256507114883,49.875,4.27929023600664));
#38698=CARTESIAN_POINT('Ctrl Pts',(5.04203735157409,57.495,4.32331156573186));
#38699=CARTESIAN_POINT('Ctrl Pts',(5.04203735157409,49.875,4.32331156573186));
#38700=CARTESIAN_POINT('Ctrl Pts',(5.06109712122993,57.495,4.36840670797621));
#38701=CARTESIAN_POINT('Ctrl Pts',(5.06109712122993,49.875,4.36840670797621));
#38702=CARTESIAN_POINT('Ctrl Pts',(5.07970066295481,57.495,4.41453743405689));
#38703=CARTESIAN_POINT('Ctrl Pts',(5.07970066295481,49.875,4.41453743405689));
#38704=CARTESIAN_POINT('Ctrl Pts',(5.09781475579234,57.495,4.46167734280668));
#38705=CARTESIAN_POINT('Ctrl Pts',(5.09781475579234,49.875,4.46167734280668));
#38706=CARTESIAN_POINT('Ctrl Pts',(5.11541439426219,57.495,4.50980818622117));
#38707=CARTESIAN_POINT('Ctrl Pts',(5.11541439426219,49.875,4.50980818622117));
#38708=CARTESIAN_POINT('Ctrl Pts',(5.13248213818673,57.495,4.55891761694258));
#38709=CARTESIAN_POINT('Ctrl Pts',(5.13248213818673,49.875,4.55891761694258));
#38710=CARTESIAN_POINT('Ctrl Pts',(5.14900691787061,57.495,4.60899638270436));
#38711=CARTESIAN_POINT('Ctrl Pts',(5.14900691787061,49.875,4.60899638270436));
#38712=CARTESIAN_POINT('Ctrl Pts',(5.16498334493441,57.495,4.66003509375248));
#38713=CARTESIAN_POINT('Ctrl Pts',(5.16498334493441,49.875,4.66003509375248));
#38714=CARTESIAN_POINT('Ctrl Pts',(5.1804106250073,57.495,4.71202254995837));
#38715=CARTESIAN_POINT('Ctrl Pts',(5.1804106250073,49.875,4.71202254995837));
#38716=CARTESIAN_POINT('Ctrl Pts',(5.1952907728175,57.495,4.764947890579));
#38717=CARTESIAN_POINT('Ctrl Pts',(5.1952907728175,49.875,4.764947890579));
#38718=CARTESIAN_POINT('Ctrl Pts',(5.2067598214933,57.495,4.8080309881172));
#38719=CARTESIAN_POINT('Ctrl Pts',(5.2067598214933,49.875,4.8080309881172));
#38720=CARTESIAN_POINT('Ctrl Pts',(5.21511826561693,57.495,4.84075823631811));
#38721=CARTESIAN_POINT('Ctrl Pts',(5.21511826561693,49.875,4.84075823631811));
#38722=CARTESIAN_POINT('Ctrl Pts',(5.22058260535447,57.495,4.86276047837853));
#38723=CARTESIAN_POINT('Ctrl Pts',(5.22058260535447,49.875,4.86276047837853));
#38724=CARTESIAN_POINT('Ctrl Pts',(5.22328778611671,57.495,4.87380761862879));
#38725=CARTESIAN_POINT('Ctrl Pts',(5.22328778611671,49.875,4.87380761862879));
#38726=CARTESIAN_POINT('',(4.65970441290368,51.145,3.72730711280926));
#38727=CARTESIAN_POINT('Ctrl Pts',(4.65970441290368,51.145,3.72730711280926));
#38728=CARTESIAN_POINT('Ctrl Pts',(4.66270326064961,51.145,3.72981733050576));
#38729=CARTESIAN_POINT('Ctrl Pts',(4.6688153380502,51.145,3.73509073349854));
#38730=CARTESIAN_POINT('Ctrl Pts',(4.67832660775297,51.145,3.7437597489088));
#38731=CARTESIAN_POINT('Ctrl Pts',(4.69169578253142,51.145,3.7568389360361));
#38732=CARTESIAN_POINT('Ctrl Pts',(4.70954474005187,51.145,3.77572337177426));
#38733=CARTESIAN_POINT('Ctrl Pts',(4.72849227702429,51.145,3.79711783384759));
#38734=CARTESIAN_POINT('Ctrl Pts',(4.74845295472311,51.145,3.82095228990398));
#38735=CARTESIAN_POINT('Ctrl Pts',(4.76926976684248,51.145,3.84708445224628));
#38736=CARTESIAN_POINT('Ctrl Pts',(4.79071829540097,51.145,3.87530262274579));
#38737=CARTESIAN_POINT('Ctrl Pts',(4.81254694822028,51.145,3.90536636162316));
#38738=CARTESIAN_POINT('Ctrl Pts',(4.83450929444277,51.145,3.93703846717723));
#38739=CARTESIAN_POINT('Ctrl Pts',(4.85639607415679,51.145,3.97011673859275));
#38740=CARTESIAN_POINT('Ctrl Pts',(4.87807598288661,51.145,4.00447382552398));
#38741=CARTESIAN_POINT('Ctrl Pts',(4.89949292161193,51.145,4.04005493051016));
#38742=CARTESIAN_POINT('Ctrl Pts',(4.92063739759527,51.145,4.07685036350543));
#38743=CARTESIAN_POINT('Ctrl Pts',(4.94152548435404,51.145,4.11487510765792));
#38744=CARTESIAN_POINT('Ctrl Pts',(4.9621766920072,51.145,4.15414724283855));
#38745=CARTESIAN_POINT('Ctrl Pts',(4.98258807456953,51.145,4.19466216292523));
#38746=CARTESIAN_POINT('Ctrl Pts',(5.00273172317852,51.145,4.23639070615327));
#38747=CARTESIAN_POINT('Ctrl Pts',(5.02256507114883,51.145,4.27929023600664));
#38748=CARTESIAN_POINT('Ctrl Pts',(5.04203735157409,51.145,4.32331156573186));
#38749=CARTESIAN_POINT('Ctrl Pts',(5.06109712122993,51.145,4.36840670797621));
#38750=CARTESIAN_POINT('Ctrl Pts',(5.07970066295481,51.145,4.41453743405689));
#38751=CARTESIAN_POINT('Ctrl Pts',(5.09781475579234,51.145,4.46167734280668));
#38752=CARTESIAN_POINT('Ctrl Pts',(5.11541439426219,51.145,4.50980818622117));
#38753=CARTESIAN_POINT('Ctrl Pts',(5.13248213818673,51.145,4.55891761694258));
#38754=CARTESIAN_POINT('Ctrl Pts',(5.14900691787061,51.145,4.60899638270436));
#38755=CARTESIAN_POINT('Ctrl Pts',(5.16498334493441,51.145,4.66003509375248));
#38756=CARTESIAN_POINT('Ctrl Pts',(5.1804106250073,51.145,4.71202254995837));
#38757=CARTESIAN_POINT('Ctrl Pts',(5.1952907728175,51.145,4.764947890579));
#38758=CARTESIAN_POINT('Ctrl Pts',(5.2067598214933,51.145,4.8080309881172));
#38759=CARTESIAN_POINT('Ctrl Pts',(5.21511826561693,51.145,4.84075823631811));
#38760=CARTESIAN_POINT('Ctrl Pts',(5.22058260535447,51.145,4.86276047837853));
#38761=CARTESIAN_POINT('Ctrl Pts',(5.22328778611671,51.145,4.87380761862879));
#38762=CARTESIAN_POINT('',(4.65970441290368,57.495,3.72730711280926));
#38763=CARTESIAN_POINT('Origin',(4.06695907338649,57.495,3.25316890053365));
#38764=CARTESIAN_POINT('',(4.18409499139877,51.145,3.34686616149372));
#38765=CARTESIAN_POINT('',(4.18409499139877,54.32,3.34686616149372));
#38766=CARTESIAN_POINT('',(4.06695907338649,51.145,3.25316890053365));
#38767=CARTESIAN_POINT('Ctrl Pts',(4.87380761862879,57.495,5.22328778611671));
#38768=CARTESIAN_POINT('Ctrl Pts',(4.87380761862879,49.875,5.22328778611671));
#38769=CARTESIAN_POINT('Ctrl Pts',(4.86276047837859,57.495,5.2205826053545));
#38770=CARTESIAN_POINT('Ctrl Pts',(4.86276047837859,49.875,5.2205826053545));
#38771=CARTESIAN_POINT('Ctrl Pts',(4.84075823631826,57.495,5.21511826561704));
#38772=CARTESIAN_POINT('Ctrl Pts',(4.84075823631826,49.875,5.21511826561704));
#38773=CARTESIAN_POINT('Ctrl Pts',(4.80803098811744,57.495,5.20675982149348));
#38774=CARTESIAN_POINT('Ctrl Pts',(4.80803098811744,49.875,5.20675982149348));
#38775=CARTESIAN_POINT('Ctrl Pts',(4.7649478905793,57.495,5.19529077281773));
#38776=CARTESIAN_POINT('Ctrl Pts',(4.7649478905793,49.875,5.19529077281773));
#38777=CARTESIAN_POINT('Ctrl Pts',(4.71202254995864,57.495,5.18041062500752));
#38778=CARTESIAN_POINT('Ctrl Pts',(4.71202254995864,49.875,5.18041062500752));
#38779=CARTESIAN_POINT('Ctrl Pts',(4.66003509375265,57.495,5.16498334493456));
#38780=CARTESIAN_POINT('Ctrl Pts',(4.66003509375265,49.875,5.16498334493456));
#38781=CARTESIAN_POINT('Ctrl Pts',(4.60899638270439,57.495,5.14900691787064));
#38782=CARTESIAN_POINT('Ctrl Pts',(4.60899638270439,49.875,5.14900691787064));
#38783=CARTESIAN_POINT('Ctrl Pts',(4.5589176169425,57.495,5.13248213818666));
#38784=CARTESIAN_POINT('Ctrl Pts',(4.5589176169425,49.875,5.13248213818666));
#38785=CARTESIAN_POINT('Ctrl Pts',(4.50980818622101,57.495,5.11541439426204));
#38786=CARTESIAN_POINT('Ctrl Pts',(4.50980818622101,49.875,5.11541439426204));
#38787=CARTESIAN_POINT('Ctrl Pts',(4.46167734280651,57.495,5.09781475579217));
#38788=CARTESIAN_POINT('Ctrl Pts',(4.46167734280651,49.875,5.09781475579217));
#38789=CARTESIAN_POINT('Ctrl Pts',(4.41453743405677,57.495,5.07970066295468));
#38790=CARTESIAN_POINT('Ctrl Pts',(4.41453743405677,49.875,5.07970066295468));
#38791=CARTESIAN_POINT('Ctrl Pts',(4.36840670797617,57.495,5.06109712122989));
#38792=CARTESIAN_POINT('Ctrl Pts',(4.36840670797617,49.875,5.06109712122989));
#38793=CARTESIAN_POINT('Ctrl Pts',(4.3233115657319,57.495,5.04203735157412));
#38794=CARTESIAN_POINT('Ctrl Pts',(4.3233115657319,49.875,5.04203735157412));
#38795=CARTESIAN_POINT('Ctrl Pts',(4.27929023600674,57.495,5.02256507114894));
#38796=CARTESIAN_POINT('Ctrl Pts',(4.27929023600674,49.875,5.02256507114894));
#38797=CARTESIAN_POINT('Ctrl Pts',(4.23639070615337,57.495,5.00273172317863));
#38798=CARTESIAN_POINT('Ctrl Pts',(4.23639070615337,49.875,5.00273172317863));
#38799=CARTESIAN_POINT('Ctrl Pts',(4.1946621629253,57.495,4.98258807456961));
#38800=CARTESIAN_POINT('Ctrl Pts',(4.1946621629253,49.875,4.98258807456961));
#38801=CARTESIAN_POINT('Ctrl Pts',(4.15414724283858,57.495,4.96217669200723));
#38802=CARTESIAN_POINT('Ctrl Pts',(4.15414724283858,49.875,4.96217669200723));
#38803=CARTESIAN_POINT('Ctrl Pts',(4.11487510765791,57.495,4.94152548435402));
#38804=CARTESIAN_POINT('Ctrl Pts',(4.11487510765791,49.875,4.94152548435402));
#38805=CARTESIAN_POINT('Ctrl Pts',(4.07685036350539,57.495,4.92063739759521));
#38806=CARTESIAN_POINT('Ctrl Pts',(4.07685036350539,49.875,4.92063739759521));
#38807=CARTESIAN_POINT('Ctrl Pts',(4.04005493051012,57.495,4.89949292161185));
#38808=CARTESIAN_POINT('Ctrl Pts',(4.04005493051012,49.875,4.89949292161185));
#38809=CARTESIAN_POINT('Ctrl Pts',(4.00447382552396,57.495,4.87807598288654));
#38810=CARTESIAN_POINT('Ctrl Pts',(4.00447382552396,49.875,4.87807598288654));
#38811=CARTESIAN_POINT('Ctrl Pts',(3.97011673859274,57.495,4.85639607415676));
#38812=CARTESIAN_POINT('Ctrl Pts',(3.97011673859274,49.875,4.85639607415676));
#38813=CARTESIAN_POINT('Ctrl Pts',(3.93703846717724,57.495,4.83450929444279));
#38814=CARTESIAN_POINT('Ctrl Pts',(3.93703846717724,49.875,4.83450929444279));
#38815=CARTESIAN_POINT('Ctrl Pts',(3.90536636162318,57.495,4.81254694822034));
#38816=CARTESIAN_POINT('Ctrl Pts',(3.90536636162318,49.875,4.81254694822034));
#38817=CARTESIAN_POINT('Ctrl Pts',(3.8753026227458,57.495,4.79071829540103));
#38818=CARTESIAN_POINT('Ctrl Pts',(3.8753026227458,49.875,4.79071829540103));
#38819=CARTESIAN_POINT('Ctrl Pts',(3.84708445224627,57.495,4.76926976684252));
#38820=CARTESIAN_POINT('Ctrl Pts',(3.84708445224627,49.875,4.76926976684252));
#38821=CARTESIAN_POINT('Ctrl Pts',(3.82095228990397,57.495,4.74845295472312));
#38822=CARTESIAN_POINT('Ctrl Pts',(3.82095228990397,49.875,4.74845295472312));
#38823=CARTESIAN_POINT('Ctrl Pts',(3.7971178338476,57.495,4.72849227702426));
#38824=CARTESIAN_POINT('Ctrl Pts',(3.7971178338476,49.875,4.72849227702426));
#38825=CARTESIAN_POINT('Ctrl Pts',(3.77572337177431,57.495,4.7095447400518));
#38826=CARTESIAN_POINT('Ctrl Pts',(3.77572337177431,49.875,4.7095447400518));
#38827=CARTESIAN_POINT('Ctrl Pts',(3.75683893603616,57.495,4.69169578253132));
#38828=CARTESIAN_POINT('Ctrl Pts',(3.75683893603616,49.875,4.69169578253132));
#38829=CARTESIAN_POINT('Ctrl Pts',(3.74375974890886,57.495,4.67832660775287));
#38830=CARTESIAN_POINT('Ctrl Pts',(3.74375974890886,49.875,4.67832660775287));
#38831=CARTESIAN_POINT('Ctrl Pts',(3.73509073349858,57.495,4.66881533805013));
#38832=CARTESIAN_POINT('Ctrl Pts',(3.73509073349858,49.875,4.66881533805013));
#38833=CARTESIAN_POINT('Ctrl Pts',(3.72981733050578,57.495,4.66270326064959));
#38834=CARTESIAN_POINT('Ctrl Pts',(3.72981733050578,49.875,4.66270326064959));
#38835=CARTESIAN_POINT('Ctrl Pts',(3.72730711280926,57.495,4.65970441290367));
#38836=CARTESIAN_POINT('Ctrl Pts',(3.72730711280926,49.875,4.65970441290367));
#38837=CARTESIAN_POINT('Ctrl Pts',(4.87380761862879,51.145,5.22328778611671));
#38838=CARTESIAN_POINT('Ctrl Pts',(4.86276047837859,51.145,5.2205826053545));
#38839=CARTESIAN_POINT('Ctrl Pts',(4.84075823631826,51.145,5.21511826561704));
#38840=CARTESIAN_POINT('Ctrl Pts',(4.80803098811744,51.145,5.20675982149348));
#38841=CARTESIAN_POINT('Ctrl Pts',(4.7649478905793,51.145,5.19529077281773));
#38842=CARTESIAN_POINT('Ctrl Pts',(4.71202254995864,51.145,5.18041062500752));
#38843=CARTESIAN_POINT('Ctrl Pts',(4.66003509375265,51.145,5.16498334493456));
#38844=CARTESIAN_POINT('Ctrl Pts',(4.60899638270439,51.145,5.14900691787064));
#38845=CARTESIAN_POINT('Ctrl Pts',(4.5589176169425,51.145,5.13248213818666));
#38846=CARTESIAN_POINT('Ctrl Pts',(4.50980818622101,51.145,5.11541439426204));
#38847=CARTESIAN_POINT('Ctrl Pts',(4.46167734280651,51.145,5.09781475579217));
#38848=CARTESIAN_POINT('Ctrl Pts',(4.41453743405677,51.145,5.07970066295468));
#38849=CARTESIAN_POINT('Ctrl Pts',(4.36840670797617,51.145,5.06109712122989));
#38850=CARTESIAN_POINT('Ctrl Pts',(4.3233115657319,51.145,5.04203735157412));
#38851=CARTESIAN_POINT('Ctrl Pts',(4.27929023600674,51.145,5.02256507114894));
#38852=CARTESIAN_POINT('Ctrl Pts',(4.23639070615337,51.145,5.00273172317863));
#38853=CARTESIAN_POINT('Ctrl Pts',(4.1946621629253,51.145,4.98258807456961));
#38854=CARTESIAN_POINT('Ctrl Pts',(4.15414724283858,51.145,4.96217669200723));
#38855=CARTESIAN_POINT('Ctrl Pts',(4.11487510765791,51.145,4.94152548435402));
#38856=CARTESIAN_POINT('Ctrl Pts',(4.07685036350539,51.145,4.92063739759521));
#38857=CARTESIAN_POINT('Ctrl Pts',(4.04005493051012,51.145,4.89949292161185));
#38858=CARTESIAN_POINT('Ctrl Pts',(4.00447382552396,51.145,4.87807598288654));
#38859=CARTESIAN_POINT('Ctrl Pts',(3.97011673859274,51.145,4.85639607415676));
#38860=CARTESIAN_POINT('Ctrl Pts',(3.93703846717724,51.145,4.83450929444279));
#38861=CARTESIAN_POINT('Ctrl Pts',(3.90536636162318,51.145,4.81254694822034));
#38862=CARTESIAN_POINT('Ctrl Pts',(3.8753026227458,51.145,4.79071829540103));
#38863=CARTESIAN_POINT('Ctrl Pts',(3.84708445224627,51.145,4.76926976684252));
#38864=CARTESIAN_POINT('Ctrl Pts',(3.82095228990397,51.145,4.74845295472312));
#38865=CARTESIAN_POINT('Ctrl Pts',(3.7971178338476,51.145,4.72849227702426));
#38866=CARTESIAN_POINT('Ctrl Pts',(3.77572337177431,51.145,4.7095447400518));
#38867=CARTESIAN_POINT('Ctrl Pts',(3.75683893603616,51.145,4.69169578253132));
#38868=CARTESIAN_POINT('Ctrl Pts',(3.74375974890886,51.145,4.67832660775287));
#38869=CARTESIAN_POINT('Ctrl Pts',(3.73509073349858,51.145,4.66881533805013));
#38870=CARTESIAN_POINT('Ctrl Pts',(3.72981733050578,51.145,4.66270326064959));
#38871=CARTESIAN_POINT('Ctrl Pts',(3.72730711280926,51.145,4.65970441290367));
#38872=CARTESIAN_POINT('Origin',(0.,54.32,0.));
#38873=CARTESIAN_POINT('',(4.69328497730872,51.145,2.58480949428933));
#38874=CARTESIAN_POINT('Origin',(0.,51.145,0.));
#38875=CARTESIAN_POINT('',(4.69328497730872,54.32,2.58480949428933));
#38876=CARTESIAN_POINT('Origin',(5.22677443144495,57.495,2.87862685522557));
#38877=CARTESIAN_POINT('',(5.22677443144495,51.145,2.87862685522557));
#38878=CARTESIAN_POINT('',(5.22677443144495,51.145,2.87862685522557));
#38879=CARTESIAN_POINT('',(5.22677443144495,57.495,2.87862685522557));
#38880=CARTESIAN_POINT('Origin',(1.50487931058895E-12,57.495,6.22890783902203E-13));
#38881=CARTESIAN_POINT('',(6.50167680247051,51.145,2.96056324982543));
#38882=CARTESIAN_POINT('',(6.50167680247051,57.495,2.96056324982543));
#38883=CARTESIAN_POINT('',(6.69081410619341,51.145,2.50394540602692));
#38884=CARTESIAN_POINT('Origin',(1.50487931058895E-12,51.145,6.22890783902203E-13));
#38885=CARTESIAN_POINT('',(6.69081410619341,57.495,2.50394540602692));
#38886=CARTESIAN_POINT('Ctrl Pts',(5.73138421404289,57.495,1.66039107437148));
#38887=CARTESIAN_POINT('Ctrl Pts',(5.73138421404289,49.875,1.66039107437148));
#38888=CARTESIAN_POINT('Ctrl Pts',(5.73511540682056,57.495,1.66156260377487));
#38889=CARTESIAN_POINT('Ctrl Pts',(5.73511540682056,49.875,1.66156260377487));
#38890=CARTESIAN_POINT('Ctrl Pts',(5.7427802739896,57.495,1.66409560210805));
#38891=CARTESIAN_POINT('Ctrl Pts',(5.7427802739896,49.875,1.66409560210805));
#38892=CARTESIAN_POINT('Ctrl Pts',(5.75488502996861,57.495,1.6684649226766));
#38893=CARTESIAN_POINT('Ctrl Pts',(5.75488502996861,49.875,1.6684649226766));
#38894=CARTESIAN_POINT('Ctrl Pts',(5.77224172513541,57.495,1.67543235427329));
#38895=CARTESIAN_POINT('Ctrl Pts',(5.77224172513541,49.875,1.67543235427329));
#38896=CARTESIAN_POINT('Ctrl Pts',(5.79595877235177,57.495,1.68604879760674));
#38897=CARTESIAN_POINT('Ctrl Pts',(5.79595877235177,49.875,1.68604879760674));
#38898=CARTESIAN_POINT('Ctrl Pts',(5.82165132013192,57.495,1.69856379474191));
#38899=CARTESIAN_POINT('Ctrl Pts',(5.82165132013192,49.875,1.69856379474191));
#38900=CARTESIAN_POINT('Ctrl Pts',(5.84921363316513,57.495,1.71294534020683));
#38901=CARTESIAN_POINT('Ctrl Pts',(5.84921363316513,49.875,1.71294534020683));
#38902=CARTESIAN_POINT('Ctrl Pts',(5.87844620539462,57.495,1.72912206102241));
#38903=CARTESIAN_POINT('Ctrl Pts',(5.87844620539462,49.875,1.72912206102241));
#38904=CARTESIAN_POINT('Ctrl Pts',(5.90906068827411,57.495,1.74698425466387));
#38905=CARTESIAN_POINT('Ctrl Pts',(5.90906068827411,49.875,1.74698425466387));
#38906=CARTESIAN_POINT('Ctrl Pts',(5.94073262861949,57.495,1.76640606389864));
#38907=CARTESIAN_POINT('Ctrl Pts',(5.94073262861949,49.875,1.76640606389864));
#38908=CARTESIAN_POINT('Ctrl Pts',(5.97314358084403,57.495,1.78726264793637));
#38909=CARTESIAN_POINT('Ctrl Pts',(5.97314358084403,49.875,1.78726264793637));
#38910=CARTESIAN_POINT('Ctrl Pts',(6.0060228350964,57.495,1.80944727788364));
#38911=CARTESIAN_POINT('Ctrl Pts',(6.0060228350964,49.875,1.80944727788364));
#38912=CARTESIAN_POINT('Ctrl Pts',(6.03920034699149,57.495,1.83289254541003));
#38913=CARTESIAN_POINT('Ctrl Pts',(6.03920034699149,49.875,1.83289254541003));
#38914=CARTESIAN_POINT('Ctrl Pts',(6.07260331771232,57.495,1.85756929242874));
#38915=CARTESIAN_POINT('Ctrl Pts',(6.07260331771232,49.875,1.85756929242874));
#38916=CARTESIAN_POINT('Ctrl Pts',(6.10621926889299,57.495,1.88347219921809));
#38917=CARTESIAN_POINT('Ctrl Pts',(6.10621926889299,49.875,1.88347219921809));
#38918=CARTESIAN_POINT('Ctrl Pts',(6.14006878432982,57.495,1.91060895733317));
#38919=CARTESIAN_POINT('Ctrl Pts',(6.14006878432982,49.875,1.91060895733317));
#38920=CARTESIAN_POINT('Ctrl Pts',(6.17417680788945,57.495,1.93898880419737));
#38921=CARTESIAN_POINT('Ctrl Pts',(6.17417680788945,49.875,1.93898880419737));
#38922=CARTESIAN_POINT('Ctrl Pts',(6.20853885514981,57.495,1.96860861168851));
#38923=CARTESIAN_POINT('Ctrl Pts',(6.20853885514981,49.875,1.96860861168851));
#38924=CARTESIAN_POINT('Ctrl Pts',(6.24311798195985,57.495,1.99945211810837));
#38925=CARTESIAN_POINT('Ctrl Pts',(6.24311798195985,49.875,1.99945211810837));
#38926=CARTESIAN_POINT('Ctrl Pts',(6.27785854554194,57.495,2.03149622201769));
#38927=CARTESIAN_POINT('Ctrl Pts',(6.27785854554194,49.875,2.03149622201769));
#38928=CARTESIAN_POINT('Ctrl Pts',(6.31269482043467,57.495,2.06471490843563));
#38929=CARTESIAN_POINT('Ctrl Pts',(6.31269482043467,49.875,2.06471490843563));
#38930=CARTESIAN_POINT('Ctrl Pts',(6.34756091533115,57.495,2.09908352929888));
#38931=CARTESIAN_POINT('Ctrl Pts',(6.34756091533115,49.875,2.09908352929888));
#38932=CARTESIAN_POINT('Ctrl Pts',(6.38240181135703,57.495,2.13458349574329));
#38933=CARTESIAN_POINT('Ctrl Pts',(6.38240181135703,49.875,2.13458349574329));
#38934=CARTESIAN_POINT('Ctrl Pts',(6.41717671306138,57.495,2.17120312938042));
#38935=CARTESIAN_POINT('Ctrl Pts',(6.41717671306138,49.875,2.17120312938042));
#38936=CARTESIAN_POINT('Ctrl Pts',(6.45185553518375,57.495,2.20893514043555));
#38937=CARTESIAN_POINT('Ctrl Pts',(6.45185553518375,49.875,2.20893514043555));
#38938=CARTESIAN_POINT('Ctrl Pts',(6.48641743997175,57.495,2.24777479550457));
#38939=CARTESIAN_POINT('Ctrl Pts',(6.48641743997175,49.875,2.24777479550457));
#38940=CARTESIAN_POINT('Ctrl Pts',(6.52084865967127,57.495,2.2877177827968));
#38941=CARTESIAN_POINT('Ctrl Pts',(6.52084865967127,49.875,2.2877177827968));
#38942=CARTESIAN_POINT('Ctrl Pts',(6.55514062276556,57.495,2.32875748935421));
#38943=CARTESIAN_POINT('Ctrl Pts',(6.55514062276556,49.875,2.32875748935421));
#38944=CARTESIAN_POINT('Ctrl Pts',(6.58928830924802,57.495,2.37088387159981));
#38945=CARTESIAN_POINT('Ctrl Pts',(6.58928830924802,49.875,2.37088387159981));
#38946=CARTESIAN_POINT('Ctrl Pts',(6.6232894242584,57.495,2.41408612451229));
#38947=CARTESIAN_POINT('Ctrl Pts',(6.6232894242584,49.875,2.41408612451229));
#38948=CARTESIAN_POINT('Ctrl Pts',(6.65037263123018,57.495,2.4495007016118));
#38949=CARTESIAN_POINT('Ctrl Pts',(6.65037263123018,49.875,2.4495007016118));
#38950=CARTESIAN_POINT('Ctrl Pts',(6.67061900235304,57.495,2.47653809829358));
#38951=CARTESIAN_POINT('Ctrl Pts',(6.67061900235304,49.875,2.47653809829358));
#38952=CARTESIAN_POINT('Ctrl Pts',(6.68408728750664,57.495,2.49477440711619));
#38953=CARTESIAN_POINT('Ctrl Pts',(6.68408728750664,49.875,2.49477440711619));
#38954=CARTESIAN_POINT('Ctrl Pts',(6.69081410619341,57.495,2.50394540602692));
#38955=CARTESIAN_POINT('Ctrl Pts',(6.69081410619341,49.875,2.50394540602692));
#38956=CARTESIAN_POINT('',(5.73138421404289,51.145,1.66039107437148));
#38957=CARTESIAN_POINT('Ctrl Pts',(5.73138421404289,51.145,1.66039107437148));
#38958=CARTESIAN_POINT('Ctrl Pts',(5.73511540682056,51.145,1.66156260377487));
#38959=CARTESIAN_POINT('Ctrl Pts',(5.7427802739896,51.145,1.66409560210805));
#38960=CARTESIAN_POINT('Ctrl Pts',(5.75488502996861,51.145,1.6684649226766));
#38961=CARTESIAN_POINT('Ctrl Pts',(5.77224172513541,51.145,1.67543235427329));
#38962=CARTESIAN_POINT('Ctrl Pts',(5.79595877235177,51.145,1.68604879760674));
#38963=CARTESIAN_POINT('Ctrl Pts',(5.82165132013192,51.145,1.69856379474191));
#38964=CARTESIAN_POINT('Ctrl Pts',(5.84921363316513,51.145,1.71294534020683));
#38965=CARTESIAN_POINT('Ctrl Pts',(5.87844620539462,51.145,1.72912206102241));
#38966=CARTESIAN_POINT('Ctrl Pts',(5.90906068827411,51.145,1.74698425466387));
#38967=CARTESIAN_POINT('Ctrl Pts',(5.94073262861949,51.145,1.76640606389864));
#38968=CARTESIAN_POINT('Ctrl Pts',(5.97314358084403,51.145,1.78726264793637));
#38969=CARTESIAN_POINT('Ctrl Pts',(6.0060228350964,51.145,1.80944727788364));
#38970=CARTESIAN_POINT('Ctrl Pts',(6.03920034699149,51.145,1.83289254541003));
#38971=CARTESIAN_POINT('Ctrl Pts',(6.07260331771232,51.145,1.85756929242874));
#38972=CARTESIAN_POINT('Ctrl Pts',(6.10621926889299,51.145,1.88347219921809));
#38973=CARTESIAN_POINT('Ctrl Pts',(6.14006878432982,51.145,1.91060895733317));
#38974=CARTESIAN_POINT('Ctrl Pts',(6.17417680788945,51.145,1.93898880419737));
#38975=CARTESIAN_POINT('Ctrl Pts',(6.20853885514981,51.145,1.96860861168851));
#38976=CARTESIAN_POINT('Ctrl Pts',(6.24311798195985,51.145,1.99945211810837));
#38977=CARTESIAN_POINT('Ctrl Pts',(6.27785854554194,51.145,2.03149622201769));
#38978=CARTESIAN_POINT('Ctrl Pts',(6.31269482043467,51.145,2.06471490843563));
#38979=CARTESIAN_POINT('Ctrl Pts',(6.34756091533115,51.145,2.09908352929888));
#38980=CARTESIAN_POINT('Ctrl Pts',(6.38240181135703,51.145,2.13458349574329));
#38981=CARTESIAN_POINT('Ctrl Pts',(6.41717671306138,51.145,2.17120312938042));
#38982=CARTESIAN_POINT('Ctrl Pts',(6.45185553518375,51.145,2.20893514043555));
#38983=CARTESIAN_POINT('Ctrl Pts',(6.48641743997175,51.145,2.24777479550457));
#38984=CARTESIAN_POINT('Ctrl Pts',(6.52084865967127,51.145,2.2877177827968));
#38985=CARTESIAN_POINT('Ctrl Pts',(6.55514062276556,51.145,2.32875748935421));
#38986=CARTESIAN_POINT('Ctrl Pts',(6.58928830924802,51.145,2.37088387159981));
#38987=CARTESIAN_POINT('Ctrl Pts',(6.6232894242584,51.145,2.41408612451229));
#38988=CARTESIAN_POINT('Ctrl Pts',(6.65037263123018,51.145,2.4495007016118));
#38989=CARTESIAN_POINT('Ctrl Pts',(6.67061900235304,51.145,2.47653809829358));
#38990=CARTESIAN_POINT('Ctrl Pts',(6.68408728750664,51.145,2.49477440711619));
#38991=CARTESIAN_POINT('Ctrl Pts',(6.69081410619341,51.145,2.50394540602692));
#38992=CARTESIAN_POINT('',(5.73138421404289,57.495,1.66039107437148));
#38993=CARTESIAN_POINT('Origin',(5.00231408838243,57.495,1.4491783055134));
#38994=CARTESIAN_POINT('',(5.1463899549833,51.145,1.4909173120086));
#38995=CARTESIAN_POINT('',(5.1463899549833,54.32,1.4909173120086));
#38996=CARTESIAN_POINT('',(5.00231408838243,51.145,1.4491783055134));
#38997=CARTESIAN_POINT('Ctrl Pts',(6.50167680247051,57.495,2.96056324982543));
#38998=CARTESIAN_POINT('Ctrl Pts',(6.50167680247051,49.875,2.96056324982543));
#38999=CARTESIAN_POINT('Ctrl Pts',(6.49043534784131,57.495,2.96229154623625));
#39000=CARTESIAN_POINT('Ctrl Pts',(6.49043534784131,49.875,2.96229154623625));
#39001=CARTESIAN_POINT('Ctrl Pts',(6.46801681444607,57.495,2.9656630481055));
#39002=CARTESIAN_POINT('Ctrl Pts',(6.46801681444607,49.875,2.9656630481055));
#39003=CARTESIAN_POINT('Ctrl Pts',(6.43458214159149,57.495,2.97046502832946));
#39004=CARTESIAN_POINT('Ctrl Pts',(6.43458214159149,49.875,2.97046502832946));
#39005=CARTESIAN_POINT('Ctrl Pts',(6.39038953466561,57.495,2.97635619664337));
#39006=CARTESIAN_POINT('Ctrl Pts',(6.39038953466561,49.875,2.97635619664337));
#39007=CARTESIAN_POINT('Ctrl Pts',(6.33579850967689,57.495,2.98286238364858));
#39008=CARTESIAN_POINT('Ctrl Pts',(6.33579850967689,49.875,2.98286238364858));
#39009=CARTESIAN_POINT('Ctrl Pts',(6.28186459845047,57.495,2.98850417352769));
#39010=CARTESIAN_POINT('Ctrl Pts',(6.28186459845047,49.875,2.98850417352769));
#39011=CARTESIAN_POINT('Ctrl Pts',(6.22859706400147,57.495,2.99327554868811));
#39012=CARTESIAN_POINT('Ctrl Pts',(6.22859706400147,49.875,2.99327554868811));
#39013=CARTESIAN_POINT('Ctrl Pts',(6.17600655789209,57.495,2.99717295692919));
#39014=CARTESIAN_POINT('Ctrl Pts',(6.17600655789209,49.875,2.99717295692919));
#39015=CARTESIAN_POINT('Ctrl Pts',(6.12410381716742,57.495,3.00019778316108));
#39016=CARTESIAN_POINT('Ctrl Pts',(6.12410381716742,49.875,3.00019778316108));
#39017=CARTESIAN_POINT('Ctrl Pts',(6.07290162599622,57.495,3.00235671375967));
#39018=CARTESIAN_POINT('Ctrl Pts',(6.07290162599622,49.875,3.00235671375967));
#39019=CARTESIAN_POINT('Ctrl Pts',(6.02241806591666,57.495,3.00366113621883));
#39020=CARTESIAN_POINT('Ctrl Pts',(6.02241806591666,49.875,3.00366113621883));
#39021=CARTESIAN_POINT('Ctrl Pts',(5.97267956506952,57.495,3.00412716938109));
#39022=CARTESIAN_POINT('Ctrl Pts',(5.97267956506952,49.875,3.00412716938109));
#39023=CARTESIAN_POINT('Ctrl Pts',(5.9237232280624,57.495,3.00377540211878));
#39024=CARTESIAN_POINT('Ctrl Pts',(5.9237232280624,49.875,3.00377540211878));
#39025=CARTESIAN_POINT('Ctrl Pts',(5.87560110342631,57.495,3.00263159433912));
#39026=CARTESIAN_POINT('Ctrl Pts',(5.87560110342631,49.875,3.00263159433912));
#39027=CARTESIAN_POINT('Ctrl Pts',(5.82837721216385,57.495,3.00072490941932));
#39028=CARTESIAN_POINT('Ctrl Pts',(5.82837721216385,49.875,3.00072490941932));
#39029=CARTESIAN_POINT('Ctrl Pts',(5.78211642456387,57.495,2.99808342690946));
#39030=CARTESIAN_POINT('Ctrl Pts',(5.78211642456387,49.875,2.99808342690946));
#39031=CARTESIAN_POINT('Ctrl Pts',(5.73687442119613,57.495,2.9947301570106));
#39032=CARTESIAN_POINT('Ctrl Pts',(5.73687442119613,49.875,2.9947301570106));
#39033=CARTESIAN_POINT('Ctrl Pts',(5.69268882427748,57.495,2.9906797244254));
#39034=CARTESIAN_POINT('Ctrl Pts',(5.69268882427748,49.875,2.9906797244254));
#39035=CARTESIAN_POINT('Ctrl Pts',(5.64956501668959,57.495,2.98593308820271));
#39036=CARTESIAN_POINT('Ctrl Pts',(5.64956501668959,49.875,2.98593308820271));
#39037=CARTESIAN_POINT('Ctrl Pts',(5.60747882861049,57.495,2.98047914221));
#39038=CARTESIAN_POINT('Ctrl Pts',(5.60747882861049,49.875,2.98047914221));
#39039=CARTESIAN_POINT('Ctrl Pts',(5.56641026634749,57.495,2.97430877025609));
#39040=CARTESIAN_POINT('Ctrl Pts',(5.56641026634749,49.875,2.97430877025609));
#39041=CARTESIAN_POINT('Ctrl Pts',(5.52637191504895,57.495,2.96742703426683));
#39042=CARTESIAN_POINT('Ctrl Pts',(5.52637191504895,49.875,2.96742703426683));
#39043=CARTESIAN_POINT('Ctrl Pts',(5.48743586913296,57.495,2.9598647928985));
#39044=CARTESIAN_POINT('Ctrl Pts',(5.48743586913296,49.875,2.9598647928985));
#39045=CARTESIAN_POINT('Ctrl Pts',(5.44977003302482,57.495,2.95169462080131));
#39046=CARTESIAN_POINT('Ctrl Pts',(5.44977003302482,49.875,2.95169462080131));
#39047=CARTESIAN_POINT('Ctrl Pts',(5.41364129622045,57.495,2.94303247002258));
#39048=CARTESIAN_POINT('Ctrl Pts',(5.41364129622045,49.875,2.94303247002258));
#39049=CARTESIAN_POINT('Ctrl Pts',(5.37936310952307,57.495,2.93401523982671));
#39050=CARTESIAN_POINT('Ctrl Pts',(5.37936310952307,49.875,2.93401523982671));
#39051=CARTESIAN_POINT('Ctrl Pts',(5.34725389048201,57.495,2.92478335875774));
#39052=CARTESIAN_POINT('Ctrl Pts',(5.34725389048201,49.875,2.92478335875774));
#39053=CARTESIAN_POINT('Ctrl Pts',(5.31759510370885,57.495,2.91546314862892));
#39054=CARTESIAN_POINT('Ctrl Pts',(5.31759510370885,49.875,2.91546314862892));
#39055=CARTESIAN_POINT('Ctrl Pts',(5.29057828960676,57.495,2.90614521320837));
#39056=CARTESIAN_POINT('Ctrl Pts',(5.29057828960676,49.875,2.90614521320837));
#39057=CARTESIAN_POINT('Ctrl Pts',(5.26630084561719,57.495,2.89688168736508));
#39058=CARTESIAN_POINT('Ctrl Pts',(5.26630084561719,49.875,2.89688168736508));
#39059=CARTESIAN_POINT('Ctrl Pts',(5.24910109063628,57.495,2.88953536864313));
#39060=CARTESIAN_POINT('Ctrl Pts',(5.24910109063628,49.875,2.88953536864313));
#39061=CARTESIAN_POINT('Ctrl Pts',(5.23745215939571,57.495,2.88406558980901));
#39062=CARTESIAN_POINT('Ctrl Pts',(5.23745215939571,49.875,2.88406558980901));
#39063=CARTESIAN_POINT('Ctrl Pts',(5.23024117954545,57.495,2.88043681055505));
#39064=CARTESIAN_POINT('Ctrl Pts',(5.23024117954545,49.875,2.88043681055505));
#39065=CARTESIAN_POINT('Ctrl Pts',(5.22677443144495,57.495,2.87862685522557));
#39066=CARTESIAN_POINT('Ctrl Pts',(5.22677443144495,49.875,2.87862685522557));
#39067=CARTESIAN_POINT('Ctrl Pts',(6.50167680247051,51.145,2.96056324982543));
#39068=CARTESIAN_POINT('Ctrl Pts',(6.49043534784131,51.145,2.96229154623625));
#39069=CARTESIAN_POINT('Ctrl Pts',(6.46801681444607,51.145,2.9656630481055));
#39070=CARTESIAN_POINT('Ctrl Pts',(6.43458214159149,51.145,2.97046502832946));
#39071=CARTESIAN_POINT('Ctrl Pts',(6.39038953466561,51.145,2.97635619664337));
#39072=CARTESIAN_POINT('Ctrl Pts',(6.33579850967689,51.145,2.98286238364858));
#39073=CARTESIAN_POINT('Ctrl Pts',(6.28186459845047,51.145,2.98850417352769));
#39074=CARTESIAN_POINT('Ctrl Pts',(6.22859706400147,51.145,2.99327554868811));
#39075=CARTESIAN_POINT('Ctrl Pts',(6.17600655789209,51.145,2.99717295692919));
#39076=CARTESIAN_POINT('Ctrl Pts',(6.12410381716742,51.145,3.00019778316108));
#39077=CARTESIAN_POINT('Ctrl Pts',(6.07290162599622,51.145,3.00235671375967));
#39078=CARTESIAN_POINT('Ctrl Pts',(6.02241806591666,51.145,3.00366113621883));
#39079=CARTESIAN_POINT('Ctrl Pts',(5.97267956506952,51.145,3.00412716938109));
#39080=CARTESIAN_POINT('Ctrl Pts',(5.9237232280624,51.145,3.00377540211878));
#39081=CARTESIAN_POINT('Ctrl Pts',(5.87560110342631,51.145,3.00263159433912));
#39082=CARTESIAN_POINT('Ctrl Pts',(5.82837721216385,51.145,3.00072490941932));
#39083=CARTESIAN_POINT('Ctrl Pts',(5.78211642456387,51.145,2.99808342690946));
#39084=CARTESIAN_POINT('Ctrl Pts',(5.73687442119613,51.145,2.9947301570106));
#39085=CARTESIAN_POINT('Ctrl Pts',(5.69268882427748,51.145,2.9906797244254));
#39086=CARTESIAN_POINT('Ctrl Pts',(5.64956501668959,51.145,2.98593308820271));
#39087=CARTESIAN_POINT('Ctrl Pts',(5.60747882861049,51.145,2.98047914221));
#39088=CARTESIAN_POINT('Ctrl Pts',(5.56641026634749,51.145,2.97430877025609));
#39089=CARTESIAN_POINT('Ctrl Pts',(5.52637191504895,51.145,2.96742703426683));
#39090=CARTESIAN_POINT('Ctrl Pts',(5.48743586913296,51.145,2.9598647928985));
#39091=CARTESIAN_POINT('Ctrl Pts',(5.44977003302482,51.145,2.95169462080131));
#39092=CARTESIAN_POINT('Ctrl Pts',(5.41364129622045,51.145,2.94303247002258));
#39093=CARTESIAN_POINT('Ctrl Pts',(5.37936310952307,51.145,2.93401523982671));
#39094=CARTESIAN_POINT('Ctrl Pts',(5.34725389048201,51.145,2.92478335875774));
#39095=CARTESIAN_POINT('Ctrl Pts',(5.31759510370885,51.145,2.91546314862892));
#39096=CARTESIAN_POINT('Ctrl Pts',(5.29057828960676,51.145,2.90614521320837));
#39097=CARTESIAN_POINT('Ctrl Pts',(5.26630084561719,51.145,2.89688168736508));
#39098=CARTESIAN_POINT('Ctrl Pts',(5.24910109063628,51.145,2.88953536864313));
#39099=CARTESIAN_POINT('Ctrl Pts',(5.23745215939571,51.145,2.88406558980901));
#39100=CARTESIAN_POINT('Ctrl Pts',(5.23024117954545,51.145,2.88043681055505));
#39101=CARTESIAN_POINT('Ctrl Pts',(5.22677443144495,51.145,2.87862685522557));
#39102=CARTESIAN_POINT('Origin',(0.,54.32,0.));
#39103=CARTESIAN_POINT('',(5.32519370006274,51.145,0.592010183030742));
#39104=CARTESIAN_POINT('Origin',(0.,51.145,0.));
#39105=CARTESIAN_POINT('',(5.32519370006274,54.32,0.592010183030742));
#39106=CARTESIAN_POINT('Origin',(5.93051272372135,57.495,0.659304453656786));
#39107=CARTESIAN_POINT('',(5.93051272372135,51.145,0.659304453656786));
#39108=CARTESIAN_POINT('',(5.93051272372135,51.145,0.659304453656786));
#39109=CARTESIAN_POINT('',(5.93051272372135,57.495,0.659304453656786));
#39110=CARTESIAN_POINT('Origin',(1.6286971771251E-12,57.495,-4.16333634234733E-16));
#39111=CARTESIAN_POINT('',(7.13972463098307,51.145,0.247119796320915));
#39112=CARTESIAN_POINT('',(7.13972463098307,57.495,0.247119796320915));
#39113=CARTESIAN_POINT('',(7.13972463098307,51.145,-0.247119796320921));
#39114=CARTESIAN_POINT('Origin',(1.6286971771251E-12,51.145,-4.16333634234733E-16));
#39115=CARTESIAN_POINT('',(7.13972463098307,57.495,-0.247119796320921));
#39116=CARTESIAN_POINT('Ctrl Pts',(5.93051272372135,57.495,-0.659304453656789));
#39117=CARTESIAN_POINT('Ctrl Pts',(5.93051272372135,49.875,-0.659304453656789));
#39118=CARTESIAN_POINT('Ctrl Pts',(5.9344082212537,57.495,-0.659649967278237));
#39119=CARTESIAN_POINT('Ctrl Pts',(5.9344082212537,49.875,-0.659649967278237));
#39120=CARTESIAN_POINT('Ctrl Pts',(5.94245897164691,57.495,-0.660242999639202));
#39121=CARTESIAN_POINT('Ctrl Pts',(5.94245897164691,49.875,-0.660242999639202));
#39122=CARTESIAN_POINT('Ctrl Pts',(5.95531437453424,57.495,-0.660838563360922));
#39123=CARTESIAN_POINT('Ctrl Pts',(5.95531437453424,49.875,-0.660838563360922));
#39124=CARTESIAN_POINT('Ctrl Pts',(5.97401619058907,57.495,-0.661043615595513));
#39125=CARTESIAN_POINT('Ctrl Pts',(5.97401619058907,49.875,-0.661043615595513));
#39126=CARTESIAN_POINT('Ctrl Pts',(5.99999062205823,57.495,-0.660311421925998));
#39127=CARTESIAN_POINT('Ctrl Pts',(5.99999062205823,49.875,-0.660311421925998));
#39128=CARTESIAN_POINT('Ctrl Pts',(6.0285167231501,57.495,-0.658581184594089));
#39129=CARTESIAN_POINT('Ctrl Pts',(6.0285167231501,49.875,-0.658581184594089));
#39130=CARTESIAN_POINT('Ctrl Pts',(6.05948455921138,57.495,-0.655842009648634));
#39131=CARTESIAN_POINT('Ctrl Pts',(6.05948455921138,49.875,-0.655842009648634));
#39132=CARTESIAN_POINT('Ctrl Pts',(6.09268249742298,57.495,-0.652083489461621));
#39133=CARTESIAN_POINT('Ctrl Pts',(6.09268249742298,49.875,-0.652083489461621));
#39134=CARTESIAN_POINT('Ctrl Pts',(6.12780215712604,57.495,-0.647296629738921));
#39135=CARTESIAN_POINT('Ctrl Pts',(6.12780215712604,49.875,-0.647296629738921));
#39136=CARTESIAN_POINT('Ctrl Pts',(6.16449561918676,57.495,-0.641473544543615));
#39137=CARTESIAN_POINT('Ctrl Pts',(6.16449561918676,49.875,-0.641473544543615));
#39138=CARTESIAN_POINT('Ctrl Pts',(6.20242090374318,57.495,-0.634607707876565));
#39139=CARTESIAN_POINT('Ctrl Pts',(6.20242090374318,49.875,-0.634607707876565));
#39140=CARTESIAN_POINT('Ctrl Pts',(6.24128706412515,57.495,-0.626694128202843));
#39141=CARTESIAN_POINT('Ctrl Pts',(6.24128706412515,49.875,-0.626694128202843));
#39142=CARTESIAN_POINT('Ctrl Pts',(6.2809112037544,57.495,-0.617730009530308));
#39143=CARTESIAN_POINT('Ctrl Pts',(6.2809112037544,49.875,-0.617730009530308));
#39144=CARTESIAN_POINT('Ctrl Pts',(6.32121490697716,57.495,-0.607714431517403));
#39145=CARTESIAN_POINT('Ctrl Pts',(6.32121490697716,49.875,-0.607714431517403));
#39146=CARTESIAN_POINT('Ctrl Pts',(6.36218460951727,57.495,-0.596647533682212));
#39147=CARTESIAN_POINT('Ctrl Pts',(6.36218460951727,49.875,-0.596647533682212));
#39148=CARTESIAN_POINT('Ctrl Pts',(6.40384227175352,57.495,-0.584530087032239));
#39149=CARTESIAN_POINT('Ctrl Pts',(6.40384227175352,49.875,-0.584530087032239));
#39150=CARTESIAN_POINT('Ctrl Pts',(6.44621447382266,57.495,-0.57136310290558));
#39151=CARTESIAN_POINT('Ctrl Pts',(6.44621447382266,49.875,-0.57136310290558));
#39152=CARTESIAN_POINT('Ctrl Pts',(6.4892958755784,57.495,-0.557147755196278));
#39153=CARTESIAN_POINT('Ctrl Pts',(6.4892958755784,49.875,-0.557147755196278));
#39154=CARTESIAN_POINT('Ctrl Pts',(6.53304612199323,57.495,-0.541884929839951));
#39155=CARTESIAN_POINT('Ctrl Pts',(6.53304612199323,49.875,-0.541884929839951));
#39156=CARTESIAN_POINT('Ctrl Pts',(6.57740496530571,57.495,-0.525574676214357));
#39157=CARTESIAN_POINT('Ctrl Pts',(6.57740496530571,49.875,-0.525574676214357));
#39158=CARTESIAN_POINT('Ctrl Pts',(6.62230172760513,57.495,-0.508215876982669));
#39159=CARTESIAN_POINT('Ctrl Pts',(6.62230172760513,49.875,-0.508215876982669));
#39160=CARTESIAN_POINT('Ctrl Pts',(6.66766610085618,57.495,-0.489806088474624));
#39161=CARTESIAN_POINT('Ctrl Pts',(6.66766610085618,49.875,-0.489806088474624));
#39162=CARTESIAN_POINT('Ctrl Pts',(6.71344014059664,57.495,-0.470341429749656));
#39163=CARTESIAN_POINT('Ctrl Pts',(6.71344014059664,49.875,-0.470341429749656));
#39164=CARTESIAN_POINT('Ctrl Pts',(6.75958168761858,57.495,-0.44981707848863));
#39165=CARTESIAN_POINT('Ctrl Pts',(6.75958168761858,49.875,-0.44981707848863));
#39166=CARTESIAN_POINT('Ctrl Pts',(6.80606015708966,57.495,-0.428228256434474));
#39167=CARTESIAN_POINT('Ctrl Pts',(6.80606015708966,49.875,-0.428228256434474));
#39168=CARTESIAN_POINT('Ctrl Pts',(6.85285448604159,57.495,-0.405571362419757));
#39169=CARTESIAN_POINT('Ctrl Pts',(6.85285448604159,49.875,-0.405571362419757));
#39170=CARTESIAN_POINT('Ctrl Pts',(6.89995030467727,57.495,-0.381845111328236));
#39171=CARTESIAN_POINT('Ctrl Pts',(6.89995030467727,49.875,-0.381845111328236));
#39172=CARTESIAN_POINT('Ctrl Pts',(6.94733716327837,57.495,-0.357052332559036));
#39173=CARTESIAN_POINT('Ctrl Pts',(6.94733716327837,49.875,-0.357052332559036));
#39174=CARTESIAN_POINT('Ctrl Pts',(6.99500658045299,57.495,-0.33120038409401));
#39175=CARTESIAN_POINT('Ctrl Pts',(6.99500658045299,49.875,-0.33120038409401));
#39176=CARTESIAN_POINT('Ctrl Pts',(7.0429523011241,57.495,-0.304298370266206));
#39177=CARTESIAN_POINT('Ctrl Pts',(7.0429523011241,49.875,-0.304298370266206));
#39178=CARTESIAN_POINT('Ctrl Pts',(7.0815264936403,57.495,-0.281943861934841));
#39179=CARTESIAN_POINT('Ctrl Pts',(7.0815264936403,49.875,-0.281943861934841));
#39180=CARTESIAN_POINT('Ctrl Pts',(7.11057846529273,57.495,-0.264712515322388));
#39181=CARTESIAN_POINT('Ctrl Pts',(7.11057846529273,49.875,-0.264712515322388));
#39182=CARTESIAN_POINT('Ctrl Pts',(7.13000027153808,57.495,-0.253018452443277));
#39183=CARTESIAN_POINT('Ctrl Pts',(7.13000027153808,49.875,-0.253018452443277));
#39184=CARTESIAN_POINT('Ctrl Pts',(7.13972463098307,57.495,-0.247119796320918));
#39185=CARTESIAN_POINT('Ctrl Pts',(7.13972463098307,49.875,-0.247119796320918));
#39186=CARTESIAN_POINT('',(5.93051272372135,51.145,-0.659304453656789));
#39187=CARTESIAN_POINT('Ctrl Pts',(5.93051272372135,51.145,-0.659304453656789));
#39188=CARTESIAN_POINT('Ctrl Pts',(5.9344082212537,51.145,-0.659649967278237));
#39189=CARTESIAN_POINT('Ctrl Pts',(5.94245897164691,51.145,-0.660242999639202));
#39190=CARTESIAN_POINT('Ctrl Pts',(5.95531437453424,51.145,-0.660838563360922));
#39191=CARTESIAN_POINT('Ctrl Pts',(5.97401619058907,51.145,-0.661043615595513));
#39192=CARTESIAN_POINT('Ctrl Pts',(5.99999062205823,51.145,-0.660311421925998));
#39193=CARTESIAN_POINT('Ctrl Pts',(6.0285167231501,51.145,-0.658581184594089));
#39194=CARTESIAN_POINT('Ctrl Pts',(6.05948455921138,51.145,-0.655842009648634));
#39195=CARTESIAN_POINT('Ctrl Pts',(6.09268249742298,51.145,-0.652083489461621));
#39196=CARTESIAN_POINT('Ctrl Pts',(6.12780215712604,51.145,-0.647296629738921));
#39197=CARTESIAN_POINT('Ctrl Pts',(6.16449561918676,51.145,-0.641473544543615));
#39198=CARTESIAN_POINT('Ctrl Pts',(6.20242090374318,51.145,-0.634607707876565));
#39199=CARTESIAN_POINT('Ctrl Pts',(6.24128706412515,51.145,-0.626694128202843));
#39200=CARTESIAN_POINT('Ctrl Pts',(6.2809112037544,51.145,-0.617730009530308));
#39201=CARTESIAN_POINT('Ctrl Pts',(6.32121490697716,51.145,-0.607714431517403));
#39202=CARTESIAN_POINT('Ctrl Pts',(6.36218460951727,51.145,-0.596647533682212));
#39203=CARTESIAN_POINT('Ctrl Pts',(6.40384227175352,51.145,-0.584530087032239));
#39204=CARTESIAN_POINT('Ctrl Pts',(6.44621447382266,51.145,-0.57136310290558));
#39205=CARTESIAN_POINT('Ctrl Pts',(6.4892958755784,51.145,-0.557147755196278));
#39206=CARTESIAN_POINT('Ctrl Pts',(6.53304612199323,51.145,-0.541884929839951));
#39207=CARTESIAN_POINT('Ctrl Pts',(6.57740496530571,51.145,-0.525574676214357));
#39208=CARTESIAN_POINT('Ctrl Pts',(6.62230172760513,51.145,-0.508215876982669));
#39209=CARTESIAN_POINT('Ctrl Pts',(6.66766610085618,51.145,-0.489806088474624));
#39210=CARTESIAN_POINT('Ctrl Pts',(6.71344014059664,51.145,-0.470341429749656));
#39211=CARTESIAN_POINT('Ctrl Pts',(6.75958168761858,51.145,-0.44981707848863));
#39212=CARTESIAN_POINT('Ctrl Pts',(6.80606015708966,51.145,-0.428228256434474));
#39213=CARTESIAN_POINT('Ctrl Pts',(6.85285448604159,51.145,-0.405571362419757));
#39214=CARTESIAN_POINT('Ctrl Pts',(6.89995030467727,51.145,-0.381845111328236));
#39215=CARTESIAN_POINT('Ctrl Pts',(6.94733716327837,51.145,-0.357052332559036));
#39216=CARTESIAN_POINT('Ctrl Pts',(6.99500658045299,51.145,-0.33120038409401));
#39217=CARTESIAN_POINT('Ctrl Pts',(7.0429523011241,51.145,-0.304298370266206));
#39218=CARTESIAN_POINT('Ctrl Pts',(7.0815264936403,51.145,-0.281943861934841));
#39219=CARTESIAN_POINT('Ctrl Pts',(7.11057846529273,51.145,-0.264712515322388));
#39220=CARTESIAN_POINT('Ctrl Pts',(7.13000027153808,51.145,-0.253018452443277));
#39221=CARTESIAN_POINT('Ctrl Pts',(7.13972463098307,51.145,-0.247119796320918));
#39222=CARTESIAN_POINT('',(5.93051272372135,57.495,-0.659304453656789));
#39223=CARTESIAN_POINT('Origin',(5.17611212951227,57.495,-0.575436549687219));
#39224=CARTESIAN_POINT('',(5.32519370006274,51.145,-0.592010183030745));
#39225=CARTESIAN_POINT('',(5.32519370006274,54.32,-0.592010183030745));
#39226=CARTESIAN_POINT('',(5.17611212951227,51.145,-0.575436549687219));
#39227=CARTESIAN_POINT('Ctrl Pts',(7.13972463098307,57.495,0.247119796320915));
#39228=CARTESIAN_POINT('Ctrl Pts',(7.13972463098307,49.875,0.247119796320915));
#39229=CARTESIAN_POINT('Ctrl Pts',(7.13000027153814,57.495,0.253018452443265));
#39230=CARTESIAN_POINT('Ctrl Pts',(7.13000027153814,49.875,0.253018452443265));
#39231=CARTESIAN_POINT('Ctrl Pts',(7.1105784652929,57.495,0.264712515322363));
#39232=CARTESIAN_POINT('Ctrl Pts',(7.1105784652929,49.875,0.264712515322363));
#39233=CARTESIAN_POINT('Ctrl Pts',(7.0815264936406,57.495,0.281943861934802));
#39234=CARTESIAN_POINT('Ctrl Pts',(7.0815264936406,49.875,0.281943861934802));
#39235=CARTESIAN_POINT('Ctrl Pts',(7.04295230112448,57.495,0.304298370266161));
#39236=CARTESIAN_POINT('Ctrl Pts',(7.04295230112448,49.875,0.304298370266161));
#39237=CARTESIAN_POINT('Ctrl Pts',(6.99500658045334,57.495,0.331200384093974));
#39238=CARTESIAN_POINT('Ctrl Pts',(6.99500658045334,49.875,0.331200384093974));
#39239=CARTESIAN_POINT('Ctrl Pts',(6.94733716327859,57.495,0.357052332559016));
#39240=CARTESIAN_POINT('Ctrl Pts',(6.94733716327859,49.875,0.357052332559016));
#39241=CARTESIAN_POINT('Ctrl Pts',(6.89995030467732,57.495,0.38184511132823));
#39242=CARTESIAN_POINT('Ctrl Pts',(6.89995030467732,49.875,0.38184511132823));
#39243=CARTESIAN_POINT('Ctrl Pts',(6.85285448604147,57.495,0.405571362419761));
#39244=CARTESIAN_POINT('Ctrl Pts',(6.85285448604147,49.875,0.405571362419761));
#39245=CARTESIAN_POINT('Ctrl Pts',(6.80606015708944,57.495,0.42822825643448));
#39246=CARTESIAN_POINT('Ctrl Pts',(6.80606015708944,49.875,0.42822825643448));
#39247=CARTESIAN_POINT('Ctrl Pts',(6.75958168761835,57.495,0.449817078488633));
#39248=CARTESIAN_POINT('Ctrl Pts',(6.75958168761835,49.875,0.449817078488633));
#39249=CARTESIAN_POINT('Ctrl Pts',(6.71344014059646,57.495,0.470341429749655));
#39250=CARTESIAN_POINT('Ctrl Pts',(6.71344014059646,49.875,0.470341429749655));
#39251=CARTESIAN_POINT('Ctrl Pts',(6.66766610085612,57.495,0.489806088474619));
#39252=CARTESIAN_POINT('Ctrl Pts',(6.66766610085612,49.875,0.489806088474619));
#39253=CARTESIAN_POINT('Ctrl Pts',(6.62230172760518,57.495,0.508215876982666));
#39254=CARTESIAN_POINT('Ctrl Pts',(6.62230172760518,49.875,0.508215876982666));
#39255=CARTESIAN_POINT('Ctrl Pts',(6.57740496530586,57.495,0.525574676214359));
#39256=CARTESIAN_POINT('Ctrl Pts',(6.57740496530586,49.875,0.525574676214359));
#39257=CARTESIAN_POINT('Ctrl Pts',(6.53304612199338,57.495,0.541884929839957));
#39258=CARTESIAN_POINT('Ctrl Pts',(6.53304612199338,49.875,0.541884929839957));
#39259=CARTESIAN_POINT('Ctrl Pts',(6.48929587557851,57.495,0.557147755196286));
#39260=CARTESIAN_POINT('Ctrl Pts',(6.48929587557851,49.875,0.557147755196286));
#39261=CARTESIAN_POINT('Ctrl Pts',(6.4462144738227,57.495,0.571363102905584));
#39262=CARTESIAN_POINT('Ctrl Pts',(6.4462144738227,49.875,0.571363102905584));
#39263=CARTESIAN_POINT('Ctrl Pts',(6.40384227175349,57.495,0.584530087032232));
#39264=CARTESIAN_POINT('Ctrl Pts',(6.40384227175349,49.875,0.584530087032232));
#39265=CARTESIAN_POINT('Ctrl Pts',(6.36218460951721,57.495,0.596647533682194));
#39266=CARTESIAN_POINT('Ctrl Pts',(6.36218460951721,49.875,0.596647533682194));
#39267=CARTESIAN_POINT('Ctrl Pts',(6.32121490697708,57.495,0.607714431517377));
#39268=CARTESIAN_POINT('Ctrl Pts',(6.32121490697708,49.875,0.607714431517377));
#39269=CARTESIAN_POINT('Ctrl Pts',(6.28091120375433,57.495,0.617730009530282));
#39270=CARTESIAN_POINT('Ctrl Pts',(6.28091120375433,49.875,0.617730009530282));
#39271=CARTESIAN_POINT('Ctrl Pts',(6.24128706412512,57.495,0.626694128202827));
#39272=CARTESIAN_POINT('Ctrl Pts',(6.24128706412512,49.875,0.626694128202827));
#39273=CARTESIAN_POINT('Ctrl Pts',(6.2024209037432,57.495,0.634607707876569));
#39274=CARTESIAN_POINT('Ctrl Pts',(6.2024209037432,49.875,0.634607707876569));
#39275=CARTESIAN_POINT('Ctrl Pts',(6.16449561918681,57.495,0.641473544543642));
#39276=CARTESIAN_POINT('Ctrl Pts',(6.16449561918681,49.875,0.641473544543642));
#39277=CARTESIAN_POINT('Ctrl Pts',(6.12780215712609,57.495,0.647296629738963));
#39278=CARTESIAN_POINT('Ctrl Pts',(6.12780215712609,49.875,0.647296629738963));
#39279=CARTESIAN_POINT('Ctrl Pts',(6.092682497423,57.495,0.652083489461662));
#39280=CARTESIAN_POINT('Ctrl Pts',(6.092682497423,49.875,0.652083489461662));
#39281=CARTESIAN_POINT('Ctrl Pts',(6.05948455921138,57.495,0.655842009648653));
#39282=CARTESIAN_POINT('Ctrl Pts',(6.05948455921138,49.875,0.655842009648653));
#39283=CARTESIAN_POINT('Ctrl Pts',(6.02851672315009,57.495,0.658581184594064));
#39284=CARTESIAN_POINT('Ctrl Pts',(6.02851672315009,49.875,0.658581184594064));
#39285=CARTESIAN_POINT('Ctrl Pts',(5.99999062205821,57.495,0.660311421925918));
#39286=CARTESIAN_POINT('Ctrl Pts',(5.99999062205821,49.875,0.660311421925918));
#39287=CARTESIAN_POINT('Ctrl Pts',(5.97401619058905,57.495,0.661043615595394));
#39288=CARTESIAN_POINT('Ctrl Pts',(5.97401619058905,49.875,0.661043615595394));
#39289=CARTESIAN_POINT('Ctrl Pts',(5.95531437453421,57.495,0.660838563360811));
#39290=CARTESIAN_POINT('Ctrl Pts',(5.95531437453421,49.875,0.660838563360811));
#39291=CARTESIAN_POINT('Ctrl Pts',(5.94245897164689,57.495,0.66024299963913));
#39292=CARTESIAN_POINT('Ctrl Pts',(5.94245897164689,49.875,0.66024299963913));
#39293=CARTESIAN_POINT('Ctrl Pts',(5.93440822125369,57.495,0.659649967278209));
#39294=CARTESIAN_POINT('Ctrl Pts',(5.93440822125369,49.875,0.659649967278209));
#39295=CARTESIAN_POINT('Ctrl Pts',(5.93051272372135,57.495,0.659304453656786));
#39296=CARTESIAN_POINT('Ctrl Pts',(5.93051272372135,49.875,0.659304453656786));
#39297=CARTESIAN_POINT('Ctrl Pts',(7.13972463098307,51.145,0.247119796320915));
#39298=CARTESIAN_POINT('Ctrl Pts',(7.13000027153814,51.145,0.253018452443265));
#39299=CARTESIAN_POINT('Ctrl Pts',(7.1105784652929,51.145,0.264712515322363));
#39300=CARTESIAN_POINT('Ctrl Pts',(7.0815264936406,51.145,0.281943861934802));
#39301=CARTESIAN_POINT('Ctrl Pts',(7.04295230112448,51.145,0.304298370266161));
#39302=CARTESIAN_POINT('Ctrl Pts',(6.99500658045334,51.145,0.331200384093974));
#39303=CARTESIAN_POINT('Ctrl Pts',(6.94733716327859,51.145,0.357052332559016));
#39304=CARTESIAN_POINT('Ctrl Pts',(6.89995030467732,51.145,0.38184511132823));
#39305=CARTESIAN_POINT('Ctrl Pts',(6.85285448604147,51.145,0.405571362419761));
#39306=CARTESIAN_POINT('Ctrl Pts',(6.80606015708944,51.145,0.42822825643448));
#39307=CARTESIAN_POINT('Ctrl Pts',(6.75958168761835,51.145,0.449817078488633));
#39308=CARTESIAN_POINT('Ctrl Pts',(6.71344014059646,51.145,0.470341429749655));
#39309=CARTESIAN_POINT('Ctrl Pts',(6.66766610085612,51.145,0.489806088474619));
#39310=CARTESIAN_POINT('Ctrl Pts',(6.62230172760518,51.145,0.508215876982666));
#39311=CARTESIAN_POINT('Ctrl Pts',(6.57740496530586,51.145,0.525574676214359));
#39312=CARTESIAN_POINT('Ctrl Pts',(6.53304612199338,51.145,0.541884929839957));
#39313=CARTESIAN_POINT('Ctrl Pts',(6.48929587557851,51.145,0.557147755196286));
#39314=CARTESIAN_POINT('Ctrl Pts',(6.4462144738227,51.145,0.571363102905584));
#39315=CARTESIAN_POINT('Ctrl Pts',(6.40384227175349,51.145,0.584530087032232));
#39316=CARTESIAN_POINT('Ctrl Pts',(6.36218460951721,51.145,0.596647533682194));
#39317=CARTESIAN_POINT('Ctrl Pts',(6.32121490697708,51.145,0.607714431517377));
#39318=CARTESIAN_POINT('Ctrl Pts',(6.28091120375433,51.145,0.617730009530282));
#39319=CARTESIAN_POINT('Ctrl Pts',(6.24128706412512,51.145,0.626694128202827));
#39320=CARTESIAN_POINT('Ctrl Pts',(6.2024209037432,51.145,0.634607707876569));
#39321=CARTESIAN_POINT('Ctrl Pts',(6.16449561918681,51.145,0.641473544543642));
#39322=CARTESIAN_POINT('Ctrl Pts',(6.12780215712609,51.145,0.647296629738963));
#39323=CARTESIAN_POINT('Ctrl Pts',(6.092682497423,51.145,0.652083489461662));
#39324=CARTESIAN_POINT('Ctrl Pts',(6.05948455921138,51.145,0.655842009648653));
#39325=CARTESIAN_POINT('Ctrl Pts',(6.02851672315009,51.145,0.658581184594064));
#39326=CARTESIAN_POINT('Ctrl Pts',(5.99999062205821,51.145,0.660311421925918));
#39327=CARTESIAN_POINT('Ctrl Pts',(5.97401619058905,51.145,0.661043615595394));
#39328=CARTESIAN_POINT('Ctrl Pts',(5.95531437453421,51.145,0.660838563360811));
#39329=CARTESIAN_POINT('Ctrl Pts',(5.94245897164689,51.145,0.66024299963913));
#39330=CARTESIAN_POINT('Ctrl Pts',(5.93440822125369,51.145,0.659649967278209));
#39331=CARTESIAN_POINT('Ctrl Pts',(5.93051272372135,51.145,0.659304453656786));
#39332=CARTESIAN_POINT('Origin',(0.,54.32,0.));
#39333=CARTESIAN_POINT('',(5.1463899549833,51.145,-1.4909173120086));
#39334=CARTESIAN_POINT('Origin',(0.,51.145,0.));
#39335=CARTESIAN_POINT('',(5.1463899549833,54.32,-1.4909173120086));
#39336=CARTESIAN_POINT('Origin',(5.73138421404289,57.495,-1.66039107437149));
#39337=CARTESIAN_POINT('',(5.73138421404289,51.145,-1.66039107437149));
#39338=CARTESIAN_POINT('',(5.73138421404289,51.145,-1.66039107437149));
#39339=CARTESIAN_POINT('',(5.73138421404289,57.495,-1.66039107437149));
#39340=CARTESIAN_POINT('Origin',(1.50456066262064E-12,57.495,-6.23660068148934E-13));
#39341=CARTESIAN_POINT('',(6.6908141061934,51.145,-2.50394540602693));
#39342=CARTESIAN_POINT('',(6.6908141061934,57.495,-2.50394540602693));
#39343=CARTESIAN_POINT('',(6.5016768024705,51.145,-2.96056324982543));
#39344=CARTESIAN_POINT('Origin',(1.50456066262064E-12,51.145,-6.23660068148934E-13));
#39345=CARTESIAN_POINT('',(6.5016768024705,57.495,-2.96056324982543));
#39346=CARTESIAN_POINT('Ctrl Pts',(5.22677443144495,57.495,-2.87862685522557));
#39347=CARTESIAN_POINT('Ctrl Pts',(5.22677443144495,49.875,-2.87862685522557));
#39348=CARTESIAN_POINT('Ctrl Pts',(5.23024117954544,57.495,-2.88043681055508));
#39349=CARTESIAN_POINT('Ctrl Pts',(5.23024117954544,49.875,-2.88043681055508));
#39350=CARTESIAN_POINT('Ctrl Pts',(5.2374521593957,57.495,-2.88406558980908));
#39351=CARTESIAN_POINT('Ctrl Pts',(5.2374521593957,49.875,-2.88406558980908));
#39352=CARTESIAN_POINT('Ctrl Pts',(5.24910109063627,57.495,-2.88953536864324));
#39353=CARTESIAN_POINT('Ctrl Pts',(5.24910109063627,49.875,-2.88953536864324));
#39354=CARTESIAN_POINT('Ctrl Pts',(5.26630084561717,57.495,-2.8968816873652));
#39355=CARTESIAN_POINT('Ctrl Pts',(5.26630084561717,49.875,-2.8968816873652));
#39356=CARTESIAN_POINT('Ctrl Pts',(5.29057828960674,57.495,-2.90614521320845));
#39357=CARTESIAN_POINT('Ctrl Pts',(5.29057828960674,49.875,-2.90614521320845));
#39358=CARTESIAN_POINT('Ctrl Pts',(5.31759510370885,57.495,-2.91546314862894));
#39359=CARTESIAN_POINT('Ctrl Pts',(5.31759510370885,49.875,-2.91546314862894));
#39360=CARTESIAN_POINT('Ctrl Pts',(5.34725389048201,57.495,-2.92478335875772));
#39361=CARTESIAN_POINT('Ctrl Pts',(5.34725389048201,49.875,-2.92478335875772));
#39362=CARTESIAN_POINT('Ctrl Pts',(5.37936310952306,57.495,-2.93401523982667));
#39363=CARTESIAN_POINT('Ctrl Pts',(5.37936310952306,49.875,-2.93401523982667));
#39364=CARTESIAN_POINT('Ctrl Pts',(5.41364129622042,57.495,-2.94303247002252));
#39365=CARTESIAN_POINT('Ctrl Pts',(5.41364129622042,49.875,-2.94303247002252));
#39366=CARTESIAN_POINT('Ctrl Pts',(5.44977003302479,57.495,-2.95169462080126));
#39367=CARTESIAN_POINT('Ctrl Pts',(5.44977003302479,49.875,-2.95169462080126));
#39368=CARTESIAN_POINT('Ctrl Pts',(5.48743586913294,57.495,-2.95986479289849));
#39369=CARTESIAN_POINT('Ctrl Pts',(5.48743586913294,49.875,-2.95986479289849));
#39370=CARTESIAN_POINT('Ctrl Pts',(5.52637191504897,57.495,-2.96742703426686));
#39371=CARTESIAN_POINT('Ctrl Pts',(5.52637191504897,49.875,-2.96742703426686));
#39372=CARTESIAN_POINT('Ctrl Pts',(5.56641026634754,57.495,-2.97430877025614));
#39373=CARTESIAN_POINT('Ctrl Pts',(5.56641026634754,49.875,-2.97430877025614));
#39374=CARTESIAN_POINT('Ctrl Pts',(5.60747882861056,57.495,-2.98047914221006));
#39375=CARTESIAN_POINT('Ctrl Pts',(5.60747882861056,49.875,-2.98047914221006));
#39376=CARTESIAN_POINT('Ctrl Pts',(5.64956501668965,57.495,-2.98593308820275));
#39377=CARTESIAN_POINT('Ctrl Pts',(5.64956501668965,49.875,-2.98593308820275));
#39378=CARTESIAN_POINT('Ctrl Pts',(5.6926888242775,57.495,-2.99067972442542));
#39379=CARTESIAN_POINT('Ctrl Pts',(5.6926888242775,49.875,-2.99067972442542));
#39380=CARTESIAN_POINT('Ctrl Pts',(5.73687442119609,57.495,-2.99473015701059));
#39381=CARTESIAN_POINT('Ctrl Pts',(5.73687442119609,49.875,-2.99473015701059));
#39382=CARTESIAN_POINT('Ctrl Pts',(5.78211642456377,57.495,-2.99808342690941));
#39383=CARTESIAN_POINT('Ctrl Pts',(5.78211642456377,49.875,-2.99808342690941));
#39384=CARTESIAN_POINT('Ctrl Pts',(5.82837721216371,57.495,-3.00072490941926));
#39385=CARTESIAN_POINT('Ctrl Pts',(5.82837721216371,49.875,-3.00072490941926));
#39386=CARTESIAN_POINT('Ctrl Pts',(5.87560110342618,57.495,-3.00263159433907));
#39387=CARTESIAN_POINT('Ctrl Pts',(5.87560110342618,49.875,-3.00263159433907));
#39388=CARTESIAN_POINT('Ctrl Pts',(5.92372322806235,57.495,-3.00377540211876));
#39389=CARTESIAN_POINT('Ctrl Pts',(5.92372322806235,49.875,-3.00377540211876));
#39390=CARTESIAN_POINT('Ctrl Pts',(5.97267956506957,57.495,-3.00412716938112));
#39391=CARTESIAN_POINT('Ctrl Pts',(5.97267956506957,49.875,-3.00412716938112));
#39392=CARTESIAN_POINT('Ctrl Pts',(6.02241806591682,57.495,-3.0036611362189));
#39393=CARTESIAN_POINT('Ctrl Pts',(6.02241806591682,49.875,-3.0036611362189));
#39394=CARTESIAN_POINT('Ctrl Pts',(6.07290162599645,57.495,-3.00235671375976));
#39395=CARTESIAN_POINT('Ctrl Pts',(6.07290162599645,49.875,-3.00235671375976));
#39396=CARTESIAN_POINT('Ctrl Pts',(6.12410381716763,57.495,-3.00019778316116));
#39397=CARTESIAN_POINT('Ctrl Pts',(6.12410381716763,49.875,-3.00019778316116));
#39398=CARTESIAN_POINT('Ctrl Pts',(6.17600655789219,57.495,-2.99717295692923));
#39399=CARTESIAN_POINT('Ctrl Pts',(6.17600655789219,49.875,-2.99717295692923));
#39400=CARTESIAN_POINT('Ctrl Pts',(6.22859706400143,57.495,-2.9932755486881));
#39401=CARTESIAN_POINT('Ctrl Pts',(6.22859706400143,49.875,-2.9932755486881));
#39402=CARTESIAN_POINT('Ctrl Pts',(6.28186459845025,57.495,-2.98850417352762));
#39403=CARTESIAN_POINT('Ctrl Pts',(6.28186459845025,49.875,-2.98850417352762));
#39404=CARTESIAN_POINT('Ctrl Pts',(6.33579850967655,57.495,-2.98286238364848));
#39405=CARTESIAN_POINT('Ctrl Pts',(6.33579850967655,49.875,-2.98286238364848));
#39406=CARTESIAN_POINT('Ctrl Pts',(6.39038953466525,57.495,-2.97635619664327));
#39407=CARTESIAN_POINT('Ctrl Pts',(6.39038953466525,49.875,-2.97635619664327));
#39408=CARTESIAN_POINT('Ctrl Pts',(6.43458214159119,57.495,-2.97046502832938));
#39409=CARTESIAN_POINT('Ctrl Pts',(6.43458214159119,49.875,-2.97046502832938));
#39410=CARTESIAN_POINT('Ctrl Pts',(6.4680168144459,57.495,-2.96566304810545));
#39411=CARTESIAN_POINT('Ctrl Pts',(6.4680168144459,49.875,-2.96566304810545));
#39412=CARTESIAN_POINT('Ctrl Pts',(6.49043534784125,57.495,-2.96229154623624));
#39413=CARTESIAN_POINT('Ctrl Pts',(6.49043534784125,49.875,-2.96229154623624));
#39414=CARTESIAN_POINT('Ctrl Pts',(6.5016768024705,57.495,-2.96056324982543));
#39415=CARTESIAN_POINT('Ctrl Pts',(6.5016768024705,49.875,-2.96056324982543));
#39416=CARTESIAN_POINT('',(5.22677443144495,51.145,-2.87862685522557));
#39417=CARTESIAN_POINT('Ctrl Pts',(5.22677443144495,51.145,-2.87862685522557));
#39418=CARTESIAN_POINT('Ctrl Pts',(5.23024117954544,51.145,-2.88043681055508));
#39419=CARTESIAN_POINT('Ctrl Pts',(5.2374521593957,51.145,-2.88406558980908));
#39420=CARTESIAN_POINT('Ctrl Pts',(5.24910109063627,51.145,-2.88953536864324));
#39421=CARTESIAN_POINT('Ctrl Pts',(5.26630084561717,51.145,-2.8968816873652));
#39422=CARTESIAN_POINT('Ctrl Pts',(5.29057828960674,51.145,-2.90614521320845));
#39423=CARTESIAN_POINT('Ctrl Pts',(5.31759510370885,51.145,-2.91546314862894));
#39424=CARTESIAN_POINT('Ctrl Pts',(5.34725389048201,51.145,-2.92478335875772));
#39425=CARTESIAN_POINT('Ctrl Pts',(5.37936310952306,51.145,-2.93401523982667));
#39426=CARTESIAN_POINT('Ctrl Pts',(5.41364129622042,51.145,-2.94303247002252));
#39427=CARTESIAN_POINT('Ctrl Pts',(5.44977003302479,51.145,-2.95169462080126));
#39428=CARTESIAN_POINT('Ctrl Pts',(5.48743586913294,51.145,-2.95986479289849));
#39429=CARTESIAN_POINT('Ctrl Pts',(5.52637191504897,51.145,-2.96742703426686));
#39430=CARTESIAN_POINT('Ctrl Pts',(5.56641026634754,51.145,-2.97430877025614));
#39431=CARTESIAN_POINT('Ctrl Pts',(5.60747882861056,51.145,-2.98047914221006));
#39432=CARTESIAN_POINT('Ctrl Pts',(5.64956501668965,51.145,-2.98593308820275));
#39433=CARTESIAN_POINT('Ctrl Pts',(5.6926888242775,51.145,-2.99067972442542));
#39434=CARTESIAN_POINT('Ctrl Pts',(5.73687442119609,51.145,-2.99473015701059));
#39435=CARTESIAN_POINT('Ctrl Pts',(5.78211642456377,51.145,-2.99808342690941));
#39436=CARTESIAN_POINT('Ctrl Pts',(5.82837721216371,51.145,-3.00072490941926));
#39437=CARTESIAN_POINT('Ctrl Pts',(5.87560110342618,51.145,-3.00263159433907));
#39438=CARTESIAN_POINT('Ctrl Pts',(5.92372322806235,51.145,-3.00377540211876));
#39439=CARTESIAN_POINT('Ctrl Pts',(5.97267956506957,51.145,-3.00412716938112));
#39440=CARTESIAN_POINT('Ctrl Pts',(6.02241806591682,51.145,-3.0036611362189));
#39441=CARTESIAN_POINT('Ctrl Pts',(6.07290162599645,51.145,-3.00235671375976));
#39442=CARTESIAN_POINT('Ctrl Pts',(6.12410381716763,51.145,-3.00019778316116));
#39443=CARTESIAN_POINT('Ctrl Pts',(6.17600655789219,51.145,-2.99717295692923));
#39444=CARTESIAN_POINT('Ctrl Pts',(6.22859706400143,51.145,-2.9932755486881));
#39445=CARTESIAN_POINT('Ctrl Pts',(6.28186459845025,51.145,-2.98850417352762));
#39446=CARTESIAN_POINT('Ctrl Pts',(6.33579850967655,51.145,-2.98286238364848));
#39447=CARTESIAN_POINT('Ctrl Pts',(6.39038953466525,51.145,-2.97635619664327));
#39448=CARTESIAN_POINT('Ctrl Pts',(6.43458214159119,51.145,-2.97046502832938));
#39449=CARTESIAN_POINT('Ctrl Pts',(6.4680168144459,51.145,-2.96566304810545));
#39450=CARTESIAN_POINT('Ctrl Pts',(6.49043534784125,51.145,-2.96229154623624));
#39451=CARTESIAN_POINT('Ctrl Pts',(6.5016768024705,51.145,-2.96056324982543));
#39452=CARTESIAN_POINT('',(5.22677443144495,57.495,-2.87862685522557));
#39453=CARTESIAN_POINT('Origin',(4.56189402049717,57.495,-2.51244640654327));
#39454=CARTESIAN_POINT('',(4.69328497730872,51.145,-2.58480949428933));
#39455=CARTESIAN_POINT('',(4.69328497730872,54.32,-2.58480949428933));
#39456=CARTESIAN_POINT('',(4.56189402049717,51.145,-2.51244640654327));
#39457=CARTESIAN_POINT('Ctrl Pts',(6.6908141061934,57.495,-2.50394540602693));
#39458=CARTESIAN_POINT('Ctrl Pts',(6.6908141061934,49.875,-2.50394540602693));
#39459=CARTESIAN_POINT('Ctrl Pts',(6.6840872875067,57.495,-2.49477440711623));
#39460=CARTESIAN_POINT('Ctrl Pts',(6.6840872875067,49.875,-2.49477440711623));
#39461=CARTESIAN_POINT('Ctrl Pts',(6.67061900235319,57.495,-2.47653809829367));
#39462=CARTESIAN_POINT('Ctrl Pts',(6.67061900235319,49.875,-2.47653809829367));
#39463=CARTESIAN_POINT('Ctrl Pts',(6.65037263123044,57.495,-2.44950070161195));
#39464=CARTESIAN_POINT('Ctrl Pts',(6.65037263123044,49.875,-2.44950070161195));
#39465=CARTESIAN_POINT('Ctrl Pts',(6.62328942425873,57.495,-2.41408612451248));
#39466=CARTESIAN_POINT('Ctrl Pts',(6.62328942425873,49.875,-2.41408612451248));
#39467=CARTESIAN_POINT('Ctrl Pts',(6.58928830924832,57.495,-2.37088387159998));
#39468=CARTESIAN_POINT('Ctrl Pts',(6.58928830924832,49.875,-2.37088387159998));
#39469=CARTESIAN_POINT('Ctrl Pts',(6.55514062276576,57.495,-2.32875748935431));
#39470=CARTESIAN_POINT('Ctrl Pts',(6.55514062276576,49.875,-2.32875748935431));
#39471=CARTESIAN_POINT('Ctrl Pts',(6.52084865967131,57.495,-2.28771778279682));
#39472=CARTESIAN_POINT('Ctrl Pts',(6.52084865967131,49.875,-2.28771778279682));
#39473=CARTESIAN_POINT('Ctrl Pts',(6.48641743997165,57.495,-2.24777479550452));
#39474=CARTESIAN_POINT('Ctrl Pts',(6.48641743997165,49.875,-2.24777479550452));
#39475=CARTESIAN_POINT('Ctrl Pts',(6.45185553518355,57.495,-2.20893514043546));
#39476=CARTESIAN_POINT('Ctrl Pts',(6.45185553518355,49.875,-2.20893514043546));
#39477=CARTESIAN_POINT('Ctrl Pts',(6.41717671306116,57.495,-2.17120312938033));
#39478=CARTESIAN_POINT('Ctrl Pts',(6.41717671306116,49.875,-2.17120312938033));
#39479=CARTESIAN_POINT('Ctrl Pts',(6.38240181135686,57.495,-2.13458349574322));
#39480=CARTESIAN_POINT('Ctrl Pts',(6.38240181135686,49.875,-2.13458349574322));
#39481=CARTESIAN_POINT('Ctrl Pts',(6.34756091533109,57.495,-2.09908352929886));
#39482=CARTESIAN_POINT('Ctrl Pts',(6.34756091533109,49.875,-2.09908352929886));
#39483=CARTESIAN_POINT('Ctrl Pts',(6.31269482043472,57.495,-2.06471490843566));
#39484=CARTESIAN_POINT('Ctrl Pts',(6.31269482043472,49.875,-2.06471490843566));
#39485=CARTESIAN_POINT('Ctrl Pts',(6.27785854554207,57.495,-2.03149622201774));
#39486=CARTESIAN_POINT('Ctrl Pts',(6.27785854554207,49.875,-2.03149622201774));
#39487=CARTESIAN_POINT('Ctrl Pts',(6.24311798195999,57.495,-1.99945211810842));
#39488=CARTESIAN_POINT('Ctrl Pts',(6.24311798195999,49.875,-1.99945211810842));
#39489=CARTESIAN_POINT('Ctrl Pts',(6.20853885514991,57.495,-1.96860861168855));
#39490=CARTESIAN_POINT('Ctrl Pts',(6.20853885514991,49.875,-1.96860861168855));
#39491=CARTESIAN_POINT('Ctrl Pts',(6.17417680788948,57.495,-1.93898880419739));
#39492=CARTESIAN_POINT('Ctrl Pts',(6.17417680788948,49.875,-1.93898880419739));
#39493=CARTESIAN_POINT('Ctrl Pts',(6.14006878432979,57.495,-1.91060895733316));
#39494=CARTESIAN_POINT('Ctrl Pts',(6.14006878432979,49.875,-1.91060895733316));
#39495=CARTESIAN_POINT('Ctrl Pts',(6.10621926889293,57.495,-1.88347219921808));
#39496=CARTESIAN_POINT('Ctrl Pts',(6.10621926889293,49.875,-1.88347219921808));
#39497=CARTESIAN_POINT('Ctrl Pts',(6.07260331771223,57.495,-1.85756929242873));
#39498=CARTESIAN_POINT('Ctrl Pts',(6.07260331771223,49.875,-1.85756929242873));
#39499=CARTESIAN_POINT('Ctrl Pts',(6.03920034699142,57.495,-1.83289254541003));
#39500=CARTESIAN_POINT('Ctrl Pts',(6.03920034699142,49.875,-1.83289254541003));
#39501=CARTESIAN_POINT('Ctrl Pts',(6.00602283509636,57.495,-1.80944727788364));
#39502=CARTESIAN_POINT('Ctrl Pts',(6.00602283509636,49.875,-1.80944727788364));
#39503=CARTESIAN_POINT('Ctrl Pts',(5.97314358084405,57.495,-1.78726264793637));
#39504=CARTESIAN_POINT('Ctrl Pts',(5.97314358084405,49.875,-1.78726264793637));
#39505=CARTESIAN_POINT('Ctrl Pts',(5.94073262861954,57.495,-1.76640606389863));
#39506=CARTESIAN_POINT('Ctrl Pts',(5.94073262861954,49.875,-1.76640606389863));
#39507=CARTESIAN_POINT('Ctrl Pts',(5.90906068827417,57.495,-1.74698425466385));
#39508=CARTESIAN_POINT('Ctrl Pts',(5.90906068827417,49.875,-1.74698425466385));
#39509=CARTESIAN_POINT('Ctrl Pts',(5.87844620539466,57.495,-1.72912206102238));
#39510=CARTESIAN_POINT('Ctrl Pts',(5.87844620539466,49.875,-1.72912206102238));
#39511=CARTESIAN_POINT('Ctrl Pts',(5.84921363316514,57.495,-1.71294534020682));
#39512=CARTESIAN_POINT('Ctrl Pts',(5.84921363316514,49.875,-1.71294534020682));
#39513=CARTESIAN_POINT('Ctrl Pts',(5.8216513201319,57.495,-1.69856379474193));
#39514=CARTESIAN_POINT('Ctrl Pts',(5.8216513201319,49.875,-1.69856379474193));
#39515=CARTESIAN_POINT('Ctrl Pts',(5.79595877235173,57.495,-1.68604879760681));
#39516=CARTESIAN_POINT('Ctrl Pts',(5.79595877235173,49.875,-1.68604879760681));
#39517=CARTESIAN_POINT('Ctrl Pts',(5.77224172513534,57.495,-1.67543235427339));
#39518=CARTESIAN_POINT('Ctrl Pts',(5.77224172513534,49.875,-1.67543235427339));
#39519=CARTESIAN_POINT('Ctrl Pts',(5.75488502996854,57.495,-1.6684649226767));
#39520=CARTESIAN_POINT('Ctrl Pts',(5.75488502996854,49.875,-1.6684649226767));
#39521=CARTESIAN_POINT('Ctrl Pts',(5.74278027398956,57.495,-1.66409560210811));
#39522=CARTESIAN_POINT('Ctrl Pts',(5.74278027398956,49.875,-1.66409560210811));
#39523=CARTESIAN_POINT('Ctrl Pts',(5.73511540682054,57.495,-1.66156260377489));
#39524=CARTESIAN_POINT('Ctrl Pts',(5.73511540682054,49.875,-1.66156260377489));
#39525=CARTESIAN_POINT('Ctrl Pts',(5.73138421404289,57.495,-1.66039107437149));
#39526=CARTESIAN_POINT('Ctrl Pts',(5.73138421404289,49.875,-1.66039107437149));
#39527=CARTESIAN_POINT('Ctrl Pts',(6.6908141061934,51.145,-2.50394540602693));
#39528=CARTESIAN_POINT('Ctrl Pts',(6.6840872875067,51.145,-2.49477440711623));
#39529=CARTESIAN_POINT('Ctrl Pts',(6.67061900235319,51.145,-2.47653809829367));
#39530=CARTESIAN_POINT('Ctrl Pts',(6.65037263123044,51.145,-2.44950070161195));
#39531=CARTESIAN_POINT('Ctrl Pts',(6.62328942425873,51.145,-2.41408612451248));
#39532=CARTESIAN_POINT('Ctrl Pts',(6.58928830924832,51.145,-2.37088387159998));
#39533=CARTESIAN_POINT('Ctrl Pts',(6.55514062276576,51.145,-2.32875748935431));
#39534=CARTESIAN_POINT('Ctrl Pts',(6.52084865967131,51.145,-2.28771778279682));
#39535=CARTESIAN_POINT('Ctrl Pts',(6.48641743997165,51.145,-2.24777479550452));
#39536=CARTESIAN_POINT('Ctrl Pts',(6.45185553518355,51.145,-2.20893514043546));
#39537=CARTESIAN_POINT('Ctrl Pts',(6.41717671306116,51.145,-2.17120312938033));
#39538=CARTESIAN_POINT('Ctrl Pts',(6.38240181135686,51.145,-2.13458349574322));
#39539=CARTESIAN_POINT('Ctrl Pts',(6.34756091533109,51.145,-2.09908352929886));
#39540=CARTESIAN_POINT('Ctrl Pts',(6.31269482043472,51.145,-2.06471490843566));
#39541=CARTESIAN_POINT('Ctrl Pts',(6.27785854554207,51.145,-2.03149622201774));
#39542=CARTESIAN_POINT('Ctrl Pts',(6.24311798195999,51.145,-1.99945211810842));
#39543=CARTESIAN_POINT('Ctrl Pts',(6.20853885514991,51.145,-1.96860861168855));
#39544=CARTESIAN_POINT('Ctrl Pts',(6.17417680788948,51.145,-1.93898880419739));
#39545=CARTESIAN_POINT('Ctrl Pts',(6.14006878432979,51.145,-1.91060895733316));
#39546=CARTESIAN_POINT('Ctrl Pts',(6.10621926889293,51.145,-1.88347219921808));
#39547=CARTESIAN_POINT('Ctrl Pts',(6.07260331771223,51.145,-1.85756929242873));
#39548=CARTESIAN_POINT('Ctrl Pts',(6.03920034699142,51.145,-1.83289254541003));
#39549=CARTESIAN_POINT('Ctrl Pts',(6.00602283509636,51.145,-1.80944727788364));
#39550=CARTESIAN_POINT('Ctrl Pts',(5.97314358084405,51.145,-1.78726264793637));
#39551=CARTESIAN_POINT('Ctrl Pts',(5.94073262861954,51.145,-1.76640606389863));
#39552=CARTESIAN_POINT('Ctrl Pts',(5.90906068827417,51.145,-1.74698425466385));
#39553=CARTESIAN_POINT('Ctrl Pts',(5.87844620539466,51.145,-1.72912206102238));
#39554=CARTESIAN_POINT('Ctrl Pts',(5.84921363316514,51.145,-1.71294534020682));
#39555=CARTESIAN_POINT('Ctrl Pts',(5.8216513201319,51.145,-1.69856379474193));
#39556=CARTESIAN_POINT('Ctrl Pts',(5.79595877235173,51.145,-1.68604879760681));
#39557=CARTESIAN_POINT('Ctrl Pts',(5.77224172513534,51.145,-1.67543235427339));
#39558=CARTESIAN_POINT('Ctrl Pts',(5.75488502996854,51.145,-1.6684649226767));
#39559=CARTESIAN_POINT('Ctrl Pts',(5.74278027398956,51.145,-1.66409560210811));
#39560=CARTESIAN_POINT('Ctrl Pts',(5.73511540682054,51.145,-1.66156260377489));
#39561=CARTESIAN_POINT('Ctrl Pts',(5.73138421404289,51.145,-1.66039107437149));
#39562=CARTESIAN_POINT('Origin',(0.,54.32,0.));
#39563=CARTESIAN_POINT('',(4.18409499139877,51.145,-3.34686616149372));
#39564=CARTESIAN_POINT('Origin',(0.,51.145,0.));
#39565=CARTESIAN_POINT('',(4.18409499139877,54.32,-3.34686616149372));
#39566=CARTESIAN_POINT('Origin',(4.65970441290367,57.495,-3.72730711280926));
#39567=CARTESIAN_POINT('',(4.65970441290367,51.145,-3.72730711280926));
#39568=CARTESIAN_POINT('',(4.65970441290367,51.145,-3.72730711280926));
#39569=CARTESIAN_POINT('',(4.65970441290367,57.495,-3.72730711280926));
#39570=CARTESIAN_POINT('Origin',(1.15136842610855E-12,57.495,-1.15195721078055E-12));
#39571=CARTESIAN_POINT('',(5.22328778611671,51.145,-4.87380761862879));
#39572=CARTESIAN_POINT('',(5.22328778611671,57.495,-4.87380761862879));
#39573=CARTESIAN_POINT('',(4.87380761862879,51.145,-5.22328778611671));
#39574=CARTESIAN_POINT('Origin',(1.15136842610855E-12,51.145,-1.15195721078055E-12));
#39575=CARTESIAN_POINT('',(4.87380761862879,57.495,-5.22328778611671));
#39576=CARTESIAN_POINT('Ctrl Pts',(3.72730711280926,57.495,-4.65970441290368));
#39577=CARTESIAN_POINT('Ctrl Pts',(3.72730711280926,49.875,-4.65970441290368));
#39578=CARTESIAN_POINT('Ctrl Pts',(3.72981733050576,57.495,-4.66270326064961));
#39579=CARTESIAN_POINT('Ctrl Pts',(3.72981733050576,49.875,-4.66270326064961));
#39580=CARTESIAN_POINT('Ctrl Pts',(3.73509073349854,57.495,-4.6688153380502));
#39581=CARTESIAN_POINT('Ctrl Pts',(3.73509073349854,49.875,-4.6688153380502));
#39582=CARTESIAN_POINT('Ctrl Pts',(3.7437597489088,57.495,-4.67832660775297));
#39583=CARTESIAN_POINT('Ctrl Pts',(3.7437597489088,49.875,-4.67832660775297));
#39584=CARTESIAN_POINT('Ctrl Pts',(3.7568389360361,57.495,-4.69169578253142));
#39585=CARTESIAN_POINT('Ctrl Pts',(3.7568389360361,49.875,-4.69169578253142));
#39586=CARTESIAN_POINT('Ctrl Pts',(3.77572337177426,57.495,-4.70954474005187));
#39587=CARTESIAN_POINT('Ctrl Pts',(3.77572337177426,49.875,-4.70954474005187));
#39588=CARTESIAN_POINT('Ctrl Pts',(3.79711783384759,57.495,-4.72849227702429));
#39589=CARTESIAN_POINT('Ctrl Pts',(3.79711783384759,49.875,-4.72849227702429));
#39590=CARTESIAN_POINT('Ctrl Pts',(3.82095228990398,57.495,-4.74845295472311));
#39591=CARTESIAN_POINT('Ctrl Pts',(3.82095228990398,49.875,-4.74845295472311));
#39592=CARTESIAN_POINT('Ctrl Pts',(3.84708445224628,57.495,-4.76926976684248));
#39593=CARTESIAN_POINT('Ctrl Pts',(3.84708445224628,49.875,-4.76926976684248));
#39594=CARTESIAN_POINT('Ctrl Pts',(3.87530262274579,57.495,-4.79071829540097));
#39595=CARTESIAN_POINT('Ctrl Pts',(3.87530262274579,49.875,-4.79071829540097));
#39596=CARTESIAN_POINT('Ctrl Pts',(3.90536636162316,57.495,-4.81254694822028));
#39597=CARTESIAN_POINT('Ctrl Pts',(3.90536636162316,49.875,-4.81254694822028));
#39598=CARTESIAN_POINT('Ctrl Pts',(3.93703846717723,57.495,-4.83450929444277));
#39599=CARTESIAN_POINT('Ctrl Pts',(3.93703846717723,49.875,-4.83450929444277));
#39600=CARTESIAN_POINT('Ctrl Pts',(3.97011673859275,57.495,-4.85639607415679));
#39601=CARTESIAN_POINT('Ctrl Pts',(3.97011673859275,49.875,-4.85639607415679));
#39602=CARTESIAN_POINT('Ctrl Pts',(4.00447382552398,57.495,-4.87807598288661));
#39603=CARTESIAN_POINT('Ctrl Pts',(4.00447382552398,49.875,-4.87807598288661));
#39604=CARTESIAN_POINT('Ctrl Pts',(4.04005493051016,57.495,-4.89949292161193));
#39605=CARTESIAN_POINT('Ctrl Pts',(4.04005493051016,49.875,-4.89949292161193));
#39606=CARTESIAN_POINT('Ctrl Pts',(4.07685036350543,57.495,-4.92063739759527));
#39607=CARTESIAN_POINT('Ctrl Pts',(4.07685036350543,49.875,-4.92063739759527));
#39608=CARTESIAN_POINT('Ctrl Pts',(4.11487510765792,57.495,-4.94152548435404));
#39609=CARTESIAN_POINT('Ctrl Pts',(4.11487510765792,49.875,-4.94152548435404));
#39610=CARTESIAN_POINT('Ctrl Pts',(4.15414724283855,57.495,-4.9621766920072));
#39611=CARTESIAN_POINT('Ctrl Pts',(4.15414724283855,49.875,-4.9621766920072));
#39612=CARTESIAN_POINT('Ctrl Pts',(4.19466216292523,57.495,-4.98258807456953));
#39613=CARTESIAN_POINT('Ctrl Pts',(4.19466216292523,49.875,-4.98258807456953));
#39614=CARTESIAN_POINT('Ctrl Pts',(4.23639070615327,57.495,-5.00273172317852));
#39615=CARTESIAN_POINT('Ctrl Pts',(4.23639070615327,49.875,-5.00273172317852));
#39616=CARTESIAN_POINT('Ctrl Pts',(4.27929023600664,57.495,-5.02256507114883));
#39617=CARTESIAN_POINT('Ctrl Pts',(4.27929023600664,49.875,-5.02256507114883));
#39618=CARTESIAN_POINT('Ctrl Pts',(4.32331156573186,57.495,-5.04203735157409));
#39619=CARTESIAN_POINT('Ctrl Pts',(4.32331156573186,49.875,-5.04203735157409));
#39620=CARTESIAN_POINT('Ctrl Pts',(4.36840670797621,57.495,-5.06109712122993));
#39621=CARTESIAN_POINT('Ctrl Pts',(4.36840670797621,49.875,-5.06109712122993));
#39622=CARTESIAN_POINT('Ctrl Pts',(4.41453743405689,57.495,-5.07970066295481));
#39623=CARTESIAN_POINT('Ctrl Pts',(4.41453743405689,49.875,-5.07970066295481));
#39624=CARTESIAN_POINT('Ctrl Pts',(4.46167734280668,57.495,-5.09781475579234));
#39625=CARTESIAN_POINT('Ctrl Pts',(4.46167734280668,49.875,-5.09781475579234));
#39626=CARTESIAN_POINT('Ctrl Pts',(4.50980818622117,57.495,-5.11541439426219));
#39627=CARTESIAN_POINT('Ctrl Pts',(4.50980818622117,49.875,-5.11541439426219));
#39628=CARTESIAN_POINT('Ctrl Pts',(4.55891761694258,57.495,-5.13248213818673));
#39629=CARTESIAN_POINT('Ctrl Pts',(4.55891761694258,49.875,-5.13248213818673));
#39630=CARTESIAN_POINT('Ctrl Pts',(4.60899638270436,57.495,-5.14900691787061));
#39631=CARTESIAN_POINT('Ctrl Pts',(4.60899638270436,49.875,-5.14900691787061));
#39632=CARTESIAN_POINT('Ctrl Pts',(4.66003509375248,57.495,-5.16498334493441));
#39633=CARTESIAN_POINT('Ctrl Pts',(4.66003509375248,49.875,-5.16498334493441));
#39634=CARTESIAN_POINT('Ctrl Pts',(4.71202254995837,57.495,-5.1804106250073));
#39635=CARTESIAN_POINT('Ctrl Pts',(4.71202254995837,49.875,-5.1804106250073));
#39636=CARTESIAN_POINT('Ctrl Pts',(4.764947890579,57.495,-5.1952907728175));
#39637=CARTESIAN_POINT('Ctrl Pts',(4.764947890579,49.875,-5.1952907728175));
#39638=CARTESIAN_POINT('Ctrl Pts',(4.8080309881172,57.495,-5.2067598214933));
#39639=CARTESIAN_POINT('Ctrl Pts',(4.8080309881172,49.875,-5.2067598214933));
#39640=CARTESIAN_POINT('Ctrl Pts',(4.84075823631811,57.495,-5.21511826561693));
#39641=CARTESIAN_POINT('Ctrl Pts',(4.84075823631811,49.875,-5.21511826561693));
#39642=CARTESIAN_POINT('Ctrl Pts',(4.86276047837853,57.495,-5.22058260535447));
#39643=CARTESIAN_POINT('Ctrl Pts',(4.86276047837853,49.875,-5.22058260535447));
#39644=CARTESIAN_POINT('Ctrl Pts',(4.87380761862879,57.495,-5.22328778611671));
#39645=CARTESIAN_POINT('Ctrl Pts',(4.87380761862879,49.875,-5.22328778611671));
#39646=CARTESIAN_POINT('',(3.72730711280926,51.145,-4.65970441290368));
#39647=CARTESIAN_POINT('Ctrl Pts',(3.72730711280926,51.145,-4.65970441290368));
#39648=CARTESIAN_POINT('Ctrl Pts',(3.72981733050576,51.145,-4.66270326064961));
#39649=CARTESIAN_POINT('Ctrl Pts',(3.73509073349854,51.145,-4.6688153380502));
#39650=CARTESIAN_POINT('Ctrl Pts',(3.7437597489088,51.145,-4.67832660775297));
#39651=CARTESIAN_POINT('Ctrl Pts',(3.7568389360361,51.145,-4.69169578253142));
#39652=CARTESIAN_POINT('Ctrl Pts',(3.77572337177426,51.145,-4.70954474005187));
#39653=CARTESIAN_POINT('Ctrl Pts',(3.79711783384759,51.145,-4.72849227702429));
#39654=CARTESIAN_POINT('Ctrl Pts',(3.82095228990398,51.145,-4.74845295472311));
#39655=CARTESIAN_POINT('Ctrl Pts',(3.84708445224628,51.145,-4.76926976684248));
#39656=CARTESIAN_POINT('Ctrl Pts',(3.87530262274579,51.145,-4.79071829540097));
#39657=CARTESIAN_POINT('Ctrl Pts',(3.90536636162316,51.145,-4.81254694822028));
#39658=CARTESIAN_POINT('Ctrl Pts',(3.93703846717723,51.145,-4.83450929444277));
#39659=CARTESIAN_POINT('Ctrl Pts',(3.97011673859275,51.145,-4.85639607415679));
#39660=CARTESIAN_POINT('Ctrl Pts',(4.00447382552398,51.145,-4.87807598288661));
#39661=CARTESIAN_POINT('Ctrl Pts',(4.04005493051016,51.145,-4.89949292161193));
#39662=CARTESIAN_POINT('Ctrl Pts',(4.07685036350543,51.145,-4.92063739759527));
#39663=CARTESIAN_POINT('Ctrl Pts',(4.11487510765792,51.145,-4.94152548435404));
#39664=CARTESIAN_POINT('Ctrl Pts',(4.15414724283855,51.145,-4.9621766920072));
#39665=CARTESIAN_POINT('Ctrl Pts',(4.19466216292523,51.145,-4.98258807456953));
#39666=CARTESIAN_POINT('Ctrl Pts',(4.23639070615327,51.145,-5.00273172317852));
#39667=CARTESIAN_POINT('Ctrl Pts',(4.27929023600664,51.145,-5.02256507114883));
#39668=CARTESIAN_POINT('Ctrl Pts',(4.32331156573186,51.145,-5.04203735157409));
#39669=CARTESIAN_POINT('Ctrl Pts',(4.36840670797621,51.145,-5.06109712122993));
#39670=CARTESIAN_POINT('Ctrl Pts',(4.41453743405689,51.145,-5.07970066295481));
#39671=CARTESIAN_POINT('Ctrl Pts',(4.46167734280668,51.145,-5.09781475579234));
#39672=CARTESIAN_POINT('Ctrl Pts',(4.50980818622117,51.145,-5.11541439426219));
#39673=CARTESIAN_POINT('Ctrl Pts',(4.55891761694258,51.145,-5.13248213818673));
#39674=CARTESIAN_POINT('Ctrl Pts',(4.60899638270436,51.145,-5.14900691787061));
#39675=CARTESIAN_POINT('Ctrl Pts',(4.66003509375248,51.145,-5.16498334493441));
#39676=CARTESIAN_POINT('Ctrl Pts',(4.71202254995837,51.145,-5.1804106250073));
#39677=CARTESIAN_POINT('Ctrl Pts',(4.764947890579,51.145,-5.1952907728175));
#39678=CARTESIAN_POINT('Ctrl Pts',(4.8080309881172,51.145,-5.2067598214933));
#39679=CARTESIAN_POINT('Ctrl Pts',(4.84075823631811,51.145,-5.21511826561693));
#39680=CARTESIAN_POINT('Ctrl Pts',(4.86276047837853,51.145,-5.22058260535447));
#39681=CARTESIAN_POINT('Ctrl Pts',(4.87380761862879,51.145,-5.22328778611671));
#39682=CARTESIAN_POINT('',(3.72730711280926,57.495,-4.65970441290368));
#39683=CARTESIAN_POINT('Origin',(3.25316890053365,57.495,-4.06695907338649));
#39684=CARTESIAN_POINT('',(3.34686616149372,51.145,-4.18409499139877));
#39685=CARTESIAN_POINT('',(3.34686616149372,54.32,-4.18409499139877));
#39686=CARTESIAN_POINT('',(3.25316890053365,51.145,-4.06695907338649));
#39687=CARTESIAN_POINT('Ctrl Pts',(5.22328778611671,57.495,-4.87380761862879));
#39688=CARTESIAN_POINT('Ctrl Pts',(5.22328778611671,49.875,-4.87380761862879));
#39689=CARTESIAN_POINT('Ctrl Pts',(5.2205826053545,57.495,-4.86276047837859));
#39690=CARTESIAN_POINT('Ctrl Pts',(5.2205826053545,49.875,-4.86276047837859));
#39691=CARTESIAN_POINT('Ctrl Pts',(5.21511826561704,57.495,-4.84075823631826));
#39692=CARTESIAN_POINT('Ctrl Pts',(5.21511826561704,49.875,-4.84075823631826));
#39693=CARTESIAN_POINT('Ctrl Pts',(5.20675982149348,57.495,-4.80803098811744));
#39694=CARTESIAN_POINT('Ctrl Pts',(5.20675982149348,49.875,-4.80803098811744));
#39695=CARTESIAN_POINT('Ctrl Pts',(5.19529077281773,57.495,-4.7649478905793));
#39696=CARTESIAN_POINT('Ctrl Pts',(5.19529077281773,49.875,-4.7649478905793));
#39697=CARTESIAN_POINT('Ctrl Pts',(5.18041062500752,57.495,-4.71202254995864));
#39698=CARTESIAN_POINT('Ctrl Pts',(5.18041062500752,49.875,-4.71202254995864));
#39699=CARTESIAN_POINT('Ctrl Pts',(5.16498334493456,57.495,-4.66003509375265));
#39700=CARTESIAN_POINT('Ctrl Pts',(5.16498334493456,49.875,-4.66003509375265));
#39701=CARTESIAN_POINT('Ctrl Pts',(5.14900691787064,57.495,-4.60899638270439));
#39702=CARTESIAN_POINT('Ctrl Pts',(5.14900691787064,49.875,-4.60899638270439));
#39703=CARTESIAN_POINT('Ctrl Pts',(5.13248213818666,57.495,-4.5589176169425));
#39704=CARTESIAN_POINT('Ctrl Pts',(5.13248213818666,49.875,-4.5589176169425));
#39705=CARTESIAN_POINT('Ctrl Pts',(5.11541439426204,57.495,-4.50980818622101));
#39706=CARTESIAN_POINT('Ctrl Pts',(5.11541439426204,49.875,-4.50980818622101));
#39707=CARTESIAN_POINT('Ctrl Pts',(5.09781475579217,57.495,-4.46167734280651));
#39708=CARTESIAN_POINT('Ctrl Pts',(5.09781475579217,49.875,-4.46167734280651));
#39709=CARTESIAN_POINT('Ctrl Pts',(5.07970066295468,57.495,-4.41453743405677));
#39710=CARTESIAN_POINT('Ctrl Pts',(5.07970066295468,49.875,-4.41453743405677));
#39711=CARTESIAN_POINT('Ctrl Pts',(5.06109712122989,57.495,-4.36840670797617));
#39712=CARTESIAN_POINT('Ctrl Pts',(5.06109712122989,49.875,-4.36840670797617));
#39713=CARTESIAN_POINT('Ctrl Pts',(5.04203735157413,57.495,-4.3233115657319));
#39714=CARTESIAN_POINT('Ctrl Pts',(5.04203735157413,49.875,-4.3233115657319));
#39715=CARTESIAN_POINT('Ctrl Pts',(5.02256507114894,57.495,-4.27929023600674));
#39716=CARTESIAN_POINT('Ctrl Pts',(5.02256507114894,49.875,-4.27929023600674));
#39717=CARTESIAN_POINT('Ctrl Pts',(5.00273172317863,57.495,-4.23639070615337));
#39718=CARTESIAN_POINT('Ctrl Pts',(5.00273172317863,49.875,-4.23639070615337));
#39719=CARTESIAN_POINT('Ctrl Pts',(4.98258807456962,57.495,-4.1946621629253));
#39720=CARTESIAN_POINT('Ctrl Pts',(4.98258807456962,49.875,-4.1946621629253));
#39721=CARTESIAN_POINT('Ctrl Pts',(4.96217669200723,57.495,-4.15414724283858));
#39722=CARTESIAN_POINT('Ctrl Pts',(4.96217669200723,49.875,-4.15414724283858));
#39723=CARTESIAN_POINT('Ctrl Pts',(4.94152548435402,57.495,-4.11487510765791));
#39724=CARTESIAN_POINT('Ctrl Pts',(4.94152548435402,49.875,-4.11487510765791));
#39725=CARTESIAN_POINT('Ctrl Pts',(4.92063739759521,57.495,-4.07685036350539));
#39726=CARTESIAN_POINT('Ctrl Pts',(4.92063739759521,49.875,-4.07685036350539));
#39727=CARTESIAN_POINT('Ctrl Pts',(4.89949292161185,57.495,-4.04005493051012));
#39728=CARTESIAN_POINT('Ctrl Pts',(4.89949292161185,49.875,-4.04005493051012));
#39729=CARTESIAN_POINT('Ctrl Pts',(4.87807598288654,57.495,-4.00447382552396));
#39730=CARTESIAN_POINT('Ctrl Pts',(4.87807598288654,49.875,-4.00447382552396));
#39731=CARTESIAN_POINT('Ctrl Pts',(4.85639607415676,57.495,-3.97011673859274));
#39732=CARTESIAN_POINT('Ctrl Pts',(4.85639607415676,49.875,-3.97011673859274));
#39733=CARTESIAN_POINT('Ctrl Pts',(4.83450929444279,57.495,-3.93703846717724));
#39734=CARTESIAN_POINT('Ctrl Pts',(4.83450929444279,49.875,-3.93703846717724));
#39735=CARTESIAN_POINT('Ctrl Pts',(4.81254694822034,57.495,-3.90536636162318));
#39736=CARTESIAN_POINT('Ctrl Pts',(4.81254694822034,49.875,-3.90536636162318));
#39737=CARTESIAN_POINT('Ctrl Pts',(4.79071829540103,57.495,-3.8753026227458));
#39738=CARTESIAN_POINT('Ctrl Pts',(4.79071829540103,49.875,-3.8753026227458));
#39739=CARTESIAN_POINT('Ctrl Pts',(4.76926976684252,57.495,-3.84708445224627));
#39740=CARTESIAN_POINT('Ctrl Pts',(4.76926976684252,49.875,-3.84708445224627));
#39741=CARTESIAN_POINT('Ctrl Pts',(4.74845295472312,57.495,-3.82095228990397));
#39742=CARTESIAN_POINT('Ctrl Pts',(4.74845295472312,49.875,-3.82095228990397));
#39743=CARTESIAN_POINT('Ctrl Pts',(4.72849227702427,57.495,-3.7971178338476));
#39744=CARTESIAN_POINT('Ctrl Pts',(4.72849227702427,49.875,-3.7971178338476));
#39745=CARTESIAN_POINT('Ctrl Pts',(4.7095447400518,57.495,-3.77572337177431));
#39746=CARTESIAN_POINT('Ctrl Pts',(4.7095447400518,49.875,-3.77572337177431));
#39747=CARTESIAN_POINT('Ctrl Pts',(4.69169578253132,57.495,-3.75683893603616));
#39748=CARTESIAN_POINT('Ctrl Pts',(4.69169578253132,49.875,-3.75683893603616));
#39749=CARTESIAN_POINT('Ctrl Pts',(4.67832660775287,57.495,-3.74375974890886));
#39750=CARTESIAN_POINT('Ctrl Pts',(4.67832660775287,49.875,-3.74375974890886));
#39751=CARTESIAN_POINT('Ctrl Pts',(4.66881533805013,57.495,-3.73509073349858));
#39752=CARTESIAN_POINT('Ctrl Pts',(4.66881533805013,49.875,-3.73509073349858));
#39753=CARTESIAN_POINT('Ctrl Pts',(4.66270326064959,57.495,-3.72981733050578));
#39754=CARTESIAN_POINT('Ctrl Pts',(4.66270326064959,49.875,-3.72981733050578));
#39755=CARTESIAN_POINT('Ctrl Pts',(4.65970441290367,57.495,-3.72730711280926));
#39756=CARTESIAN_POINT('Ctrl Pts',(4.65970441290367,49.875,-3.72730711280926));
#39757=CARTESIAN_POINT('Ctrl Pts',(5.22328778611671,51.145,-4.87380761862879));
#39758=CARTESIAN_POINT('Ctrl Pts',(5.2205826053545,51.145,-4.86276047837859));
#39759=CARTESIAN_POINT('Ctrl Pts',(5.21511826561704,51.145,-4.84075823631826));
#39760=CARTESIAN_POINT('Ctrl Pts',(5.20675982149348,51.145,-4.80803098811744));
#39761=CARTESIAN_POINT('Ctrl Pts',(5.19529077281773,51.145,-4.7649478905793));
#39762=CARTESIAN_POINT('Ctrl Pts',(5.18041062500752,51.145,-4.71202254995864));
#39763=CARTESIAN_POINT('Ctrl Pts',(5.16498334493456,51.145,-4.66003509375265));
#39764=CARTESIAN_POINT('Ctrl Pts',(5.14900691787064,51.145,-4.60899638270439));
#39765=CARTESIAN_POINT('Ctrl Pts',(5.13248213818666,51.145,-4.5589176169425));
#39766=CARTESIAN_POINT('Ctrl Pts',(5.11541439426204,51.145,-4.50980818622101));
#39767=CARTESIAN_POINT('Ctrl Pts',(5.09781475579217,51.145,-4.46167734280651));
#39768=CARTESIAN_POINT('Ctrl Pts',(5.07970066295468,51.145,-4.41453743405677));
#39769=CARTESIAN_POINT('Ctrl Pts',(5.06109712122989,51.145,-4.36840670797617));
#39770=CARTESIAN_POINT('Ctrl Pts',(5.04203735157413,51.145,-4.3233115657319));
#39771=CARTESIAN_POINT('Ctrl Pts',(5.02256507114894,51.145,-4.27929023600674));
#39772=CARTESIAN_POINT('Ctrl Pts',(5.00273172317863,51.145,-4.23639070615337));
#39773=CARTESIAN_POINT('Ctrl Pts',(4.98258807456962,51.145,-4.1946621629253));
#39774=CARTESIAN_POINT('Ctrl Pts',(4.96217669200723,51.145,-4.15414724283858));
#39775=CARTESIAN_POINT('Ctrl Pts',(4.94152548435402,51.145,-4.11487510765791));
#39776=CARTESIAN_POINT('Ctrl Pts',(4.92063739759521,51.145,-4.07685036350539));
#39777=CARTESIAN_POINT('Ctrl Pts',(4.89949292161185,51.145,-4.04005493051012));
#39778=CARTESIAN_POINT('Ctrl Pts',(4.87807598288654,51.145,-4.00447382552396));
#39779=CARTESIAN_POINT('Ctrl Pts',(4.85639607415676,51.145,-3.97011673859274));
#39780=CARTESIAN_POINT('Ctrl Pts',(4.83450929444279,51.145,-3.93703846717724));
#39781=CARTESIAN_POINT('Ctrl Pts',(4.81254694822034,51.145,-3.90536636162318));
#39782=CARTESIAN_POINT('Ctrl Pts',(4.79071829540103,51.145,-3.8753026227458));
#39783=CARTESIAN_POINT('Ctrl Pts',(4.76926976684252,51.145,-3.84708445224627));
#39784=CARTESIAN_POINT('Ctrl Pts',(4.74845295472312,51.145,-3.82095228990397));
#39785=CARTESIAN_POINT('Ctrl Pts',(4.72849227702427,51.145,-3.7971178338476));
#39786=CARTESIAN_POINT('Ctrl Pts',(4.7095447400518,51.145,-3.77572337177431));
#39787=CARTESIAN_POINT('Ctrl Pts',(4.69169578253132,51.145,-3.75683893603616));
#39788=CARTESIAN_POINT('Ctrl Pts',(4.67832660775287,51.145,-3.74375974890886));
#39789=CARTESIAN_POINT('Ctrl Pts',(4.66881533805013,51.145,-3.73509073349858));
#39790=CARTESIAN_POINT('Ctrl Pts',(4.66270326064959,51.145,-3.72981733050578));
#39791=CARTESIAN_POINT('Ctrl Pts',(4.65970441290367,51.145,-3.72730711280926));
#39792=CARTESIAN_POINT('Origin',(0.,54.32,0.));
#39793=CARTESIAN_POINT('',(2.58480949428932,51.145,-4.69328497730873));
#39794=CARTESIAN_POINT('Origin',(0.,51.145,0.));
#39795=CARTESIAN_POINT('',(2.58480949428932,54.32,-4.69328497730873));
#39796=CARTESIAN_POINT('Origin',(2.87862685522556,57.495,-5.22677443144495));
#39797=CARTESIAN_POINT('',(2.87862685522556,51.145,-5.22677443144495));
#39798=CARTESIAN_POINT('',(2.87862685522556,51.145,-5.22677443144495));
#39799=CARTESIAN_POINT('',(2.87862685522556,57.495,-5.22677443144495));
#39800=CARTESIAN_POINT('Origin',(6.22890783902202E-13,57.495,-1.50487931058895E-12));
#39801=CARTESIAN_POINT('',(2.96056324982543,51.145,-6.50167680247051));
#39802=CARTESIAN_POINT('',(2.96056324982543,57.495,-6.50167680247051));
#39803=CARTESIAN_POINT('',(2.50394540602692,51.145,-6.69081410619341));
#39804=CARTESIAN_POINT('Origin',(6.22890783902202E-13,51.145,-1.50487931058895E-12));
#39805=CARTESIAN_POINT('',(2.50394540602692,57.495,-6.69081410619341));
#39806=CARTESIAN_POINT('Ctrl Pts',(1.66039107437148,57.495,-5.73138421404289));
#39807=CARTESIAN_POINT('Ctrl Pts',(1.66039107437148,49.875,-5.73138421404289));
#39808=CARTESIAN_POINT('Ctrl Pts',(1.66156260377487,57.495,-5.73511540682056));
#39809=CARTESIAN_POINT('Ctrl Pts',(1.66156260377487,49.875,-5.73511540682056));
#39810=CARTESIAN_POINT('Ctrl Pts',(1.66409560210805,57.495,-5.7427802739896));
#39811=CARTESIAN_POINT('Ctrl Pts',(1.66409560210805,49.875,-5.7427802739896));
#39812=CARTESIAN_POINT('Ctrl Pts',(1.6684649226766,57.495,-5.75488502996861));
#39813=CARTESIAN_POINT('Ctrl Pts',(1.6684649226766,49.875,-5.75488502996861));
#39814=CARTESIAN_POINT('Ctrl Pts',(1.67543235427329,57.495,-5.77224172513541));
#39815=CARTESIAN_POINT('Ctrl Pts',(1.67543235427329,49.875,-5.77224172513541));
#39816=CARTESIAN_POINT('Ctrl Pts',(1.68604879760674,57.495,-5.79595877235177));
#39817=CARTESIAN_POINT('Ctrl Pts',(1.68604879760674,49.875,-5.79595877235177));
#39818=CARTESIAN_POINT('Ctrl Pts',(1.69856379474191,57.495,-5.82165132013192));
#39819=CARTESIAN_POINT('Ctrl Pts',(1.69856379474191,49.875,-5.82165132013192));
#39820=CARTESIAN_POINT('Ctrl Pts',(1.71294534020683,57.495,-5.84921363316513));
#39821=CARTESIAN_POINT('Ctrl Pts',(1.71294534020683,49.875,-5.84921363316513));
#39822=CARTESIAN_POINT('Ctrl Pts',(1.7291220610224,57.495,-5.87844620539462));
#39823=CARTESIAN_POINT('Ctrl Pts',(1.7291220610224,49.875,-5.87844620539462));
#39824=CARTESIAN_POINT('Ctrl Pts',(1.74698425466387,57.495,-5.90906068827411));
#39825=CARTESIAN_POINT('Ctrl Pts',(1.74698425466387,49.875,-5.90906068827411));
#39826=CARTESIAN_POINT('Ctrl Pts',(1.76640606389864,57.495,-5.94073262861949));
#39827=CARTESIAN_POINT('Ctrl Pts',(1.76640606389864,49.875,-5.94073262861949));
#39828=CARTESIAN_POINT('Ctrl Pts',(1.78726264793636,57.495,-5.97314358084403));
#39829=CARTESIAN_POINT('Ctrl Pts',(1.78726264793636,49.875,-5.97314358084403));
#39830=CARTESIAN_POINT('Ctrl Pts',(1.80944727788364,57.495,-6.00602283509639));
#39831=CARTESIAN_POINT('Ctrl Pts',(1.80944727788364,49.875,-6.00602283509639));
#39832=CARTESIAN_POINT('Ctrl Pts',(1.83289254541003,57.495,-6.03920034699149));
#39833=CARTESIAN_POINT('Ctrl Pts',(1.83289254541003,49.875,-6.03920034699149));
#39834=CARTESIAN_POINT('Ctrl Pts',(1.85756929242873,57.495,-6.07260331771232));
#39835=CARTESIAN_POINT('Ctrl Pts',(1.85756929242873,49.875,-6.07260331771232));
#39836=CARTESIAN_POINT('Ctrl Pts',(1.88347219921808,57.495,-6.106219268893));
#39837=CARTESIAN_POINT('Ctrl Pts',(1.88347219921808,49.875,-6.106219268893));
#39838=CARTESIAN_POINT('Ctrl Pts',(1.91060895733316,57.495,-6.14006878432982));
#39839=CARTESIAN_POINT('Ctrl Pts',(1.91060895733316,49.875,-6.14006878432982));
#39840=CARTESIAN_POINT('Ctrl Pts',(1.93898880419737,57.495,-6.17417680788945));
#39841=CARTESIAN_POINT('Ctrl Pts',(1.93898880419737,49.875,-6.17417680788945));
#39842=CARTESIAN_POINT('Ctrl Pts',(1.96860861168851,57.495,-6.20853885514981));
#39843=CARTESIAN_POINT('Ctrl Pts',(1.96860861168851,49.875,-6.20853885514981));
#39844=CARTESIAN_POINT('Ctrl Pts',(1.99945211810836,57.495,-6.24311798195985));
#39845=CARTESIAN_POINT('Ctrl Pts',(1.99945211810836,49.875,-6.24311798195985));
#39846=CARTESIAN_POINT('Ctrl Pts',(2.03149622201768,57.495,-6.27785854554194));
#39847=CARTESIAN_POINT('Ctrl Pts',(2.03149622201768,49.875,-6.27785854554194));
#39848=CARTESIAN_POINT('Ctrl Pts',(2.06471490843563,57.495,-6.31269482043467));
#39849=CARTESIAN_POINT('Ctrl Pts',(2.06471490843563,49.875,-6.31269482043467));
#39850=CARTESIAN_POINT('Ctrl Pts',(2.09908352929888,57.495,-6.34756091533115));
#39851=CARTESIAN_POINT('Ctrl Pts',(2.09908352929888,49.875,-6.34756091533115));
#39852=CARTESIAN_POINT('Ctrl Pts',(2.13458349574329,57.495,-6.38240181135703));
#39853=CARTESIAN_POINT('Ctrl Pts',(2.13458349574329,49.875,-6.38240181135703));
#39854=CARTESIAN_POINT('Ctrl Pts',(2.17120312938042,57.495,-6.41717671306138));
#39855=CARTESIAN_POINT('Ctrl Pts',(2.17120312938042,49.875,-6.41717671306138));
#39856=CARTESIAN_POINT('Ctrl Pts',(2.20893514043555,57.495,-6.45185553518375));
#39857=CARTESIAN_POINT('Ctrl Pts',(2.20893514043555,49.875,-6.45185553518375));
#39858=CARTESIAN_POINT('Ctrl Pts',(2.24777479550457,57.495,-6.48641743997175));
#39859=CARTESIAN_POINT('Ctrl Pts',(2.24777479550457,49.875,-6.48641743997175));
#39860=CARTESIAN_POINT('Ctrl Pts',(2.2877177827968,57.495,-6.52084865967127));
#39861=CARTESIAN_POINT('Ctrl Pts',(2.2877177827968,49.875,-6.52084865967127));
#39862=CARTESIAN_POINT('Ctrl Pts',(2.3287574893542,57.495,-6.55514062276556));
#39863=CARTESIAN_POINT('Ctrl Pts',(2.3287574893542,49.875,-6.55514062276556));
#39864=CARTESIAN_POINT('Ctrl Pts',(2.37088387159981,57.495,-6.58928830924802));
#39865=CARTESIAN_POINT('Ctrl Pts',(2.37088387159981,49.875,-6.58928830924802));
#39866=CARTESIAN_POINT('Ctrl Pts',(2.41408612451229,57.495,-6.6232894242584));
#39867=CARTESIAN_POINT('Ctrl Pts',(2.41408612451229,49.875,-6.6232894242584));
#39868=CARTESIAN_POINT('Ctrl Pts',(2.4495007016118,57.495,-6.65037263123018));
#39869=CARTESIAN_POINT('Ctrl Pts',(2.4495007016118,49.875,-6.65037263123018));
#39870=CARTESIAN_POINT('Ctrl Pts',(2.47653809829358,57.495,-6.67061900235304));
#39871=CARTESIAN_POINT('Ctrl Pts',(2.47653809829358,49.875,-6.67061900235304));
#39872=CARTESIAN_POINT('Ctrl Pts',(2.49477440711619,57.495,-6.68408728750665));
#39873=CARTESIAN_POINT('Ctrl Pts',(2.49477440711619,49.875,-6.68408728750665));
#39874=CARTESIAN_POINT('Ctrl Pts',(2.50394540602692,57.495,-6.69081410619341));
#39875=CARTESIAN_POINT('Ctrl Pts',(2.50394540602692,49.875,-6.69081410619341));
#39876=CARTESIAN_POINT('',(1.66039107437148,51.145,-5.73138421404289));
#39877=CARTESIAN_POINT('Ctrl Pts',(1.66039107437148,51.145,-5.73138421404289));
#39878=CARTESIAN_POINT('Ctrl Pts',(1.66156260377487,51.145,-5.73511540682056));
#39879=CARTESIAN_POINT('Ctrl Pts',(1.66409560210805,51.145,-5.7427802739896));
#39880=CARTESIAN_POINT('Ctrl Pts',(1.6684649226766,51.145,-5.75488502996861));
#39881=CARTESIAN_POINT('Ctrl Pts',(1.67543235427329,51.145,-5.77224172513541));
#39882=CARTESIAN_POINT('Ctrl Pts',(1.68604879760674,51.145,-5.79595877235177));
#39883=CARTESIAN_POINT('Ctrl Pts',(1.69856379474191,51.145,-5.82165132013192));
#39884=CARTESIAN_POINT('Ctrl Pts',(1.71294534020683,51.145,-5.84921363316513));
#39885=CARTESIAN_POINT('Ctrl Pts',(1.7291220610224,51.145,-5.87844620539462));
#39886=CARTESIAN_POINT('Ctrl Pts',(1.74698425466387,51.145,-5.90906068827411));
#39887=CARTESIAN_POINT('Ctrl Pts',(1.76640606389864,51.145,-5.94073262861949));
#39888=CARTESIAN_POINT('Ctrl Pts',(1.78726264793636,51.145,-5.97314358084403));
#39889=CARTESIAN_POINT('Ctrl Pts',(1.80944727788364,51.145,-6.00602283509639));
#39890=CARTESIAN_POINT('Ctrl Pts',(1.83289254541003,51.145,-6.03920034699149));
#39891=CARTESIAN_POINT('Ctrl Pts',(1.85756929242873,51.145,-6.07260331771232));
#39892=CARTESIAN_POINT('Ctrl Pts',(1.88347219921808,51.145,-6.106219268893));
#39893=CARTESIAN_POINT('Ctrl Pts',(1.91060895733316,51.145,-6.14006878432982));
#39894=CARTESIAN_POINT('Ctrl Pts',(1.93898880419737,51.145,-6.17417680788945));
#39895=CARTESIAN_POINT('Ctrl Pts',(1.96860861168851,51.145,-6.20853885514981));
#39896=CARTESIAN_POINT('Ctrl Pts',(1.99945211810836,51.145,-6.24311798195985));
#39897=CARTESIAN_POINT('Ctrl Pts',(2.03149622201768,51.145,-6.27785854554194));
#39898=CARTESIAN_POINT('Ctrl Pts',(2.06471490843563,51.145,-6.31269482043467));
#39899=CARTESIAN_POINT('Ctrl Pts',(2.09908352929888,51.145,-6.34756091533115));
#39900=CARTESIAN_POINT('Ctrl Pts',(2.13458349574329,51.145,-6.38240181135703));
#39901=CARTESIAN_POINT('Ctrl Pts',(2.17120312938042,51.145,-6.41717671306138));
#39902=CARTESIAN_POINT('Ctrl Pts',(2.20893514043555,51.145,-6.45185553518375));
#39903=CARTESIAN_POINT('Ctrl Pts',(2.24777479550457,51.145,-6.48641743997175));
#39904=CARTESIAN_POINT('Ctrl Pts',(2.2877177827968,51.145,-6.52084865967127));
#39905=CARTESIAN_POINT('Ctrl Pts',(2.3287574893542,51.145,-6.55514062276556));
#39906=CARTESIAN_POINT('Ctrl Pts',(2.37088387159981,51.145,-6.58928830924802));
#39907=CARTESIAN_POINT('Ctrl Pts',(2.41408612451229,51.145,-6.6232894242584));
#39908=CARTESIAN_POINT('Ctrl Pts',(2.4495007016118,51.145,-6.65037263123018));
#39909=CARTESIAN_POINT('Ctrl Pts',(2.47653809829358,51.145,-6.67061900235304));
#39910=CARTESIAN_POINT('Ctrl Pts',(2.49477440711619,51.145,-6.68408728750665));
#39911=CARTESIAN_POINT('Ctrl Pts',(2.50394540602692,51.145,-6.69081410619341));
#39912=CARTESIAN_POINT('',(1.66039107437148,57.495,-5.73138421404289));
#39913=CARTESIAN_POINT('Origin',(1.44917830551339,57.495,-5.00231408838243));
#39914=CARTESIAN_POINT('',(1.4909173120086,51.145,-5.1463899549833));
#39915=CARTESIAN_POINT('',(1.4909173120086,54.32,-5.1463899549833));
#39916=CARTESIAN_POINT('',(1.44917830551339,51.145,-5.00231408838243));
#39917=CARTESIAN_POINT('Ctrl Pts',(2.96056324982543,57.495,-6.50167680247051));
#39918=CARTESIAN_POINT('Ctrl Pts',(2.96056324982543,49.875,-6.50167680247051));
#39919=CARTESIAN_POINT('Ctrl Pts',(2.96229154623625,57.495,-6.49043534784131));
#39920=CARTESIAN_POINT('Ctrl Pts',(2.96229154623625,49.875,-6.49043534784131));
#39921=CARTESIAN_POINT('Ctrl Pts',(2.96566304810549,57.495,-6.46801681444607));
#39922=CARTESIAN_POINT('Ctrl Pts',(2.96566304810549,49.875,-6.46801681444607));
#39923=CARTESIAN_POINT('Ctrl Pts',(2.97046502832945,57.495,-6.43458214159149));
#39924=CARTESIAN_POINT('Ctrl Pts',(2.97046502832945,49.875,-6.43458214159149));
#39925=CARTESIAN_POINT('Ctrl Pts',(2.97635619664337,57.495,-6.39038953466561));
#39926=CARTESIAN_POINT('Ctrl Pts',(2.97635619664337,49.875,-6.39038953466561));
#39927=CARTESIAN_POINT('Ctrl Pts',(2.98286238364857,57.495,-6.33579850967689));
#39928=CARTESIAN_POINT('Ctrl Pts',(2.98286238364857,49.875,-6.33579850967689));
#39929=CARTESIAN_POINT('Ctrl Pts',(2.98850417352769,57.495,-6.28186459845047));
#39930=CARTESIAN_POINT('Ctrl Pts',(2.98850417352769,49.875,-6.28186459845047));
#39931=CARTESIAN_POINT('Ctrl Pts',(2.99327554868811,57.495,-6.22859706400148));
#39932=CARTESIAN_POINT('Ctrl Pts',(2.99327554868811,49.875,-6.22859706400148));
#39933=CARTESIAN_POINT('Ctrl Pts',(2.99717295692919,57.495,-6.17600655789209));
#39934=CARTESIAN_POINT('Ctrl Pts',(2.99717295692919,49.875,-6.17600655789209));
#39935=CARTESIAN_POINT('Ctrl Pts',(3.00019778316108,57.495,-6.12410381716742));
#39936=CARTESIAN_POINT('Ctrl Pts',(3.00019778316108,49.875,-6.12410381716742));
#39937=CARTESIAN_POINT('Ctrl Pts',(3.00235671375967,57.495,-6.07290162599622));
#39938=CARTESIAN_POINT('Ctrl Pts',(3.00235671375967,49.875,-6.07290162599622));
#39939=CARTESIAN_POINT('Ctrl Pts',(3.00366113621882,57.495,-6.02241806591666));
#39940=CARTESIAN_POINT('Ctrl Pts',(3.00366113621882,49.875,-6.02241806591666));
#39941=CARTESIAN_POINT('Ctrl Pts',(3.00412716938109,57.495,-5.97267956506952));
#39942=CARTESIAN_POINT('Ctrl Pts',(3.00412716938109,49.875,-5.97267956506952));
#39943=CARTESIAN_POINT('Ctrl Pts',(3.00377540211877,57.495,-5.9237232280624));
#39944=CARTESIAN_POINT('Ctrl Pts',(3.00377540211877,49.875,-5.9237232280624));
#39945=CARTESIAN_POINT('Ctrl Pts',(3.00263159433912,57.495,-5.87560110342631));
#39946=CARTESIAN_POINT('Ctrl Pts',(3.00263159433912,49.875,-5.87560110342631));
#39947=CARTESIAN_POINT('Ctrl Pts',(3.00072490941932,57.495,-5.82837721216385));
#39948=CARTESIAN_POINT('Ctrl Pts',(3.00072490941932,49.875,-5.82837721216385));
#39949=CARTESIAN_POINT('Ctrl Pts',(2.99808342690946,57.495,-5.78211642456387));
#39950=CARTESIAN_POINT('Ctrl Pts',(2.99808342690946,49.875,-5.78211642456387));
#39951=CARTESIAN_POINT('Ctrl Pts',(2.9947301570106,57.495,-5.73687442119613));
#39952=CARTESIAN_POINT('Ctrl Pts',(2.9947301570106,49.875,-5.73687442119613));
#39953=CARTESIAN_POINT('Ctrl Pts',(2.9906797244254,57.495,-5.69268882427748));
#39954=CARTESIAN_POINT('Ctrl Pts',(2.9906797244254,49.875,-5.69268882427748));
#39955=CARTESIAN_POINT('Ctrl Pts',(2.98593308820271,57.495,-5.64956501668959));
#39956=CARTESIAN_POINT('Ctrl Pts',(2.98593308820271,49.875,-5.64956501668959));
#39957=CARTESIAN_POINT('Ctrl Pts',(2.98047914221,57.495,-5.6074788286105));
#39958=CARTESIAN_POINT('Ctrl Pts',(2.98047914221,49.875,-5.6074788286105));
#39959=CARTESIAN_POINT('Ctrl Pts',(2.97430877025608,57.495,-5.56641026634749));
#39960=CARTESIAN_POINT('Ctrl Pts',(2.97430877025608,49.875,-5.56641026634749));
#39961=CARTESIAN_POINT('Ctrl Pts',(2.96742703426683,57.495,-5.52637191504895));
#39962=CARTESIAN_POINT('Ctrl Pts',(2.96742703426683,49.875,-5.52637191504895));
#39963=CARTESIAN_POINT('Ctrl Pts',(2.95986479289849,57.495,-5.48743586913296));
#39964=CARTESIAN_POINT('Ctrl Pts',(2.95986479289849,49.875,-5.48743586913296));
#39965=CARTESIAN_POINT('Ctrl Pts',(2.95169462080131,57.495,-5.44977003302482));
#39966=CARTESIAN_POINT('Ctrl Pts',(2.95169462080131,49.875,-5.44977003302482));
#39967=CARTESIAN_POINT('Ctrl Pts',(2.94303247002258,57.495,-5.41364129622045));
#39968=CARTESIAN_POINT('Ctrl Pts',(2.94303247002258,49.875,-5.41364129622045));
#39969=CARTESIAN_POINT('Ctrl Pts',(2.93401523982671,57.495,-5.37936310952307));
#39970=CARTESIAN_POINT('Ctrl Pts',(2.93401523982671,49.875,-5.37936310952307));
#39971=CARTESIAN_POINT('Ctrl Pts',(2.92478335875774,57.495,-5.34725389048201));
#39972=CARTESIAN_POINT('Ctrl Pts',(2.92478335875774,49.875,-5.34725389048201));
#39973=CARTESIAN_POINT('Ctrl Pts',(2.91546314862891,57.495,-5.31759510370886));
#39974=CARTESIAN_POINT('Ctrl Pts',(2.91546314862891,49.875,-5.31759510370886));
#39975=CARTESIAN_POINT('Ctrl Pts',(2.90614521320837,57.495,-5.29057828960676));
#39976=CARTESIAN_POINT('Ctrl Pts',(2.90614521320837,49.875,-5.29057828960676));
#39977=CARTESIAN_POINT('Ctrl Pts',(2.89688168736508,57.495,-5.26630084561719));
#39978=CARTESIAN_POINT('Ctrl Pts',(2.89688168736508,49.875,-5.26630084561719));
#39979=CARTESIAN_POINT('Ctrl Pts',(2.88953536864313,57.495,-5.24910109063628));
#39980=CARTESIAN_POINT('Ctrl Pts',(2.88953536864313,49.875,-5.24910109063628));
#39981=CARTESIAN_POINT('Ctrl Pts',(2.884065589809,57.495,-5.23745215939571));
#39982=CARTESIAN_POINT('Ctrl Pts',(2.884065589809,49.875,-5.23745215939571));
#39983=CARTESIAN_POINT('Ctrl Pts',(2.88043681055505,57.495,-5.23024117954545));
#39984=CARTESIAN_POINT('Ctrl Pts',(2.88043681055505,49.875,-5.23024117954545));
#39985=CARTESIAN_POINT('Ctrl Pts',(2.87862685522556,57.495,-5.22677443144495));
#39986=CARTESIAN_POINT('Ctrl Pts',(2.87862685522556,49.875,-5.22677443144495));
#39987=CARTESIAN_POINT('Ctrl Pts',(2.96056324982543,51.145,-6.50167680247051));
#39988=CARTESIAN_POINT('Ctrl Pts',(2.96229154623625,51.145,-6.49043534784131));
#39989=CARTESIAN_POINT('Ctrl Pts',(2.96566304810549,51.145,-6.46801681444607));
#39990=CARTESIAN_POINT('Ctrl Pts',(2.97046502832945,51.145,-6.43458214159149));
#39991=CARTESIAN_POINT('Ctrl Pts',(2.97635619664337,51.145,-6.39038953466561));
#39992=CARTESIAN_POINT('Ctrl Pts',(2.98286238364857,51.145,-6.33579850967689));
#39993=CARTESIAN_POINT('Ctrl Pts',(2.98850417352769,51.145,-6.28186459845047));
#39994=CARTESIAN_POINT('Ctrl Pts',(2.99327554868811,51.145,-6.22859706400148));
#39995=CARTESIAN_POINT('Ctrl Pts',(2.99717295692919,51.145,-6.17600655789209));
#39996=CARTESIAN_POINT('Ctrl Pts',(3.00019778316108,51.145,-6.12410381716742));
#39997=CARTESIAN_POINT('Ctrl Pts',(3.00235671375967,51.145,-6.07290162599622));
#39998=CARTESIAN_POINT('Ctrl Pts',(3.00366113621882,51.145,-6.02241806591666));
#39999=CARTESIAN_POINT('Ctrl Pts',(3.00412716938109,51.145,-5.97267956506952));
#40000=CARTESIAN_POINT('Ctrl Pts',(3.00377540211877,51.145,-5.9237232280624));
#40001=CARTESIAN_POINT('Ctrl Pts',(3.00263159433912,51.145,-5.87560110342631));
#40002=CARTESIAN_POINT('Ctrl Pts',(3.00072490941932,51.145,-5.82837721216385));
#40003=CARTESIAN_POINT('Ctrl Pts',(2.99808342690946,51.145,-5.78211642456387));
#40004=CARTESIAN_POINT('Ctrl Pts',(2.9947301570106,51.145,-5.73687442119613));
#40005=CARTESIAN_POINT('Ctrl Pts',(2.9906797244254,51.145,-5.69268882427748));
#40006=CARTESIAN_POINT('Ctrl Pts',(2.98593308820271,51.145,-5.64956501668959));
#40007=CARTESIAN_POINT('Ctrl Pts',(2.98047914221,51.145,-5.6074788286105));
#40008=CARTESIAN_POINT('Ctrl Pts',(2.97430877025608,51.145,-5.56641026634749));
#40009=CARTESIAN_POINT('Ctrl Pts',(2.96742703426683,51.145,-5.52637191504895));
#40010=CARTESIAN_POINT('Ctrl Pts',(2.95986479289849,51.145,-5.48743586913296));
#40011=CARTESIAN_POINT('Ctrl Pts',(2.95169462080131,51.145,-5.44977003302482));
#40012=CARTESIAN_POINT('Ctrl Pts',(2.94303247002258,51.145,-5.41364129622045));
#40013=CARTESIAN_POINT('Ctrl Pts',(2.93401523982671,51.145,-5.37936310952307));
#40014=CARTESIAN_POINT('Ctrl Pts',(2.92478335875774,51.145,-5.34725389048201));
#40015=CARTESIAN_POINT('Ctrl Pts',(2.91546314862891,51.145,-5.31759510370886));
#40016=CARTESIAN_POINT('Ctrl Pts',(2.90614521320837,51.145,-5.29057828960676));
#40017=CARTESIAN_POINT('Ctrl Pts',(2.89688168736508,51.145,-5.26630084561719));
#40018=CARTESIAN_POINT('Ctrl Pts',(2.88953536864313,51.145,-5.24910109063628));
#40019=CARTESIAN_POINT('Ctrl Pts',(2.884065589809,51.145,-5.23745215939571));
#40020=CARTESIAN_POINT('Ctrl Pts',(2.88043681055505,51.145,-5.23024117954545));
#40021=CARTESIAN_POINT('Ctrl Pts',(2.87862685522556,51.145,-5.22677443144495));
#40022=CARTESIAN_POINT('Origin',(0.,54.32,0.));
#40023=CARTESIAN_POINT('',(0.592010183030743,51.145,-5.32519370006274));
#40024=CARTESIAN_POINT('Origin',(0.,51.145,0.));
#40025=CARTESIAN_POINT('',(0.592010183030743,54.32,-5.32519370006274));
#40026=CARTESIAN_POINT('Origin',(0.659304453656786,57.495,-5.93051272372135));
#40027=CARTESIAN_POINT('',(0.659304453656786,51.145,-5.93051272372135));
#40028=CARTESIAN_POINT('',(0.659304453656786,51.145,-5.93051272372135));
#40029=CARTESIAN_POINT('',(0.659304453656786,57.495,-5.93051272372135));
#40030=CARTESIAN_POINT('Origin',(-4.16333634234633E-16,57.495,-1.6286971771251E-12));
#40031=CARTESIAN_POINT('',(0.247119796320915,51.145,-7.13972463098307));
#40032=CARTESIAN_POINT('',(0.247119796320915,57.495,-7.13972463098307));
#40033=CARTESIAN_POINT('',(-0.247119796320921,51.145,-7.13972463098307));
#40034=CARTESIAN_POINT('Origin',(-4.16333634234633E-16,51.145,-1.6286971771251E-12));
#40035=CARTESIAN_POINT('',(-0.247119796320921,57.495,-7.13972463098307));
#40036=CARTESIAN_POINT('Ctrl Pts',(-0.659304453656788,57.495,-5.93051272372135));
#40037=CARTESIAN_POINT('Ctrl Pts',(-0.659304453656788,49.875,-5.93051272372135));
#40038=CARTESIAN_POINT('Ctrl Pts',(-0.659649967278237,57.495,-5.9344082212537));
#40039=CARTESIAN_POINT('Ctrl Pts',(-0.659649967278237,49.875,-5.9344082212537));
#40040=CARTESIAN_POINT('Ctrl Pts',(-0.660242999639202,57.495,-5.94245897164691));
#40041=CARTESIAN_POINT('Ctrl Pts',(-0.660242999639202,49.875,-5.94245897164691));
#40042=CARTESIAN_POINT('Ctrl Pts',(-0.660838563360922,57.495,-5.95531437453424));
#40043=CARTESIAN_POINT('Ctrl Pts',(-0.660838563360922,49.875,-5.95531437453424));
#40044=CARTESIAN_POINT('Ctrl Pts',(-0.661043615595512,57.495,-5.97401619058907));
#40045=CARTESIAN_POINT('Ctrl Pts',(-0.661043615595512,49.875,-5.97401619058907));
#40046=CARTESIAN_POINT('Ctrl Pts',(-0.660311421925998,57.495,-5.99999062205823));
#40047=CARTESIAN_POINT('Ctrl Pts',(-0.660311421925998,49.875,-5.99999062205823));
#40048=CARTESIAN_POINT('Ctrl Pts',(-0.658581184594089,57.495,-6.0285167231501));
#40049=CARTESIAN_POINT('Ctrl Pts',(-0.658581184594089,49.875,-6.0285167231501));
#40050=CARTESIAN_POINT('Ctrl Pts',(-0.655842009648634,57.495,-6.05948455921138));
#40051=CARTESIAN_POINT('Ctrl Pts',(-0.655842009648634,49.875,-6.05948455921138));
#40052=CARTESIAN_POINT('Ctrl Pts',(-0.65208348946162,57.495,-6.09268249742298));
#40053=CARTESIAN_POINT('Ctrl Pts',(-0.65208348946162,49.875,-6.09268249742298));
#40054=CARTESIAN_POINT('Ctrl Pts',(-0.647296629738921,57.495,-6.12780215712604));
#40055=CARTESIAN_POINT('Ctrl Pts',(-0.647296629738921,49.875,-6.12780215712604));
#40056=CARTESIAN_POINT('Ctrl Pts',(-0.641473544543615,57.495,-6.16449561918676));
#40057=CARTESIAN_POINT('Ctrl Pts',(-0.641473544543615,49.875,-6.16449561918676));
#40058=CARTESIAN_POINT('Ctrl Pts',(-0.634607707876565,57.495,-6.20242090374318));
#40059=CARTESIAN_POINT('Ctrl Pts',(-0.634607707876565,49.875,-6.20242090374318));
#40060=CARTESIAN_POINT('Ctrl Pts',(-0.626694128202842,57.495,-6.24128706412515));
#40061=CARTESIAN_POINT('Ctrl Pts',(-0.626694128202842,49.875,-6.24128706412515));
#40062=CARTESIAN_POINT('Ctrl Pts',(-0.617730009530307,57.495,-6.2809112037544));
#40063=CARTESIAN_POINT('Ctrl Pts',(-0.617730009530307,49.875,-6.2809112037544));
#40064=CARTESIAN_POINT('Ctrl Pts',(-0.607714431517402,57.495,-6.32121490697716));
#40065=CARTESIAN_POINT('Ctrl Pts',(-0.607714431517402,49.875,-6.32121490697716));
#40066=CARTESIAN_POINT('Ctrl Pts',(-0.596647533682212,57.495,-6.36218460951727));
#40067=CARTESIAN_POINT('Ctrl Pts',(-0.596647533682212,49.875,-6.36218460951727));
#40068=CARTESIAN_POINT('Ctrl Pts',(-0.584530087032238,57.495,-6.40384227175352));
#40069=CARTESIAN_POINT('Ctrl Pts',(-0.584530087032238,49.875,-6.40384227175352));
#40070=CARTESIAN_POINT('Ctrl Pts',(-0.57136310290558,57.495,-6.44621447382266));
#40071=CARTESIAN_POINT('Ctrl Pts',(-0.57136310290558,49.875,-6.44621447382266));
#40072=CARTESIAN_POINT('Ctrl Pts',(-0.557147755196278,57.495,-6.4892958755784));
#40073=CARTESIAN_POINT('Ctrl Pts',(-0.557147755196278,49.875,-6.4892958755784));
#40074=CARTESIAN_POINT('Ctrl Pts',(-0.54188492983995,57.495,-6.53304612199323));
#40075=CARTESIAN_POINT('Ctrl Pts',(-0.54188492983995,49.875,-6.53304612199323));
#40076=CARTESIAN_POINT('Ctrl Pts',(-0.525574676214357,57.495,-6.57740496530571));
#40077=CARTESIAN_POINT('Ctrl Pts',(-0.525574676214357,49.875,-6.57740496530571));
#40078=CARTESIAN_POINT('Ctrl Pts',(-0.508215876982669,57.495,-6.62230172760513));
#40079=CARTESIAN_POINT('Ctrl Pts',(-0.508215876982669,49.875,-6.62230172760513));
#40080=CARTESIAN_POINT('Ctrl Pts',(-0.489806088474623,57.495,-6.66766610085618));
#40081=CARTESIAN_POINT('Ctrl Pts',(-0.489806088474623,49.875,-6.66766610085618));
#40082=CARTESIAN_POINT('Ctrl Pts',(-0.470341429749656,57.495,-6.71344014059664));
#40083=CARTESIAN_POINT('Ctrl Pts',(-0.470341429749656,49.875,-6.71344014059664));
#40084=CARTESIAN_POINT('Ctrl Pts',(-0.44981707848863,57.495,-6.75958168761858));
#40085=CARTESIAN_POINT('Ctrl Pts',(-0.44981707848863,49.875,-6.75958168761858));
#40086=CARTESIAN_POINT('Ctrl Pts',(-0.428228256434474,57.495,-6.80606015708966));
#40087=CARTESIAN_POINT('Ctrl Pts',(-0.428228256434474,49.875,-6.80606015708966));
#40088=CARTESIAN_POINT('Ctrl Pts',(-0.405571362419757,57.495,-6.85285448604159));
#40089=CARTESIAN_POINT('Ctrl Pts',(-0.405571362419757,49.875,-6.85285448604159));
#40090=CARTESIAN_POINT('Ctrl Pts',(-0.381845111328235,57.495,-6.89995030467727));
#40091=CARTESIAN_POINT('Ctrl Pts',(-0.381845111328235,49.875,-6.89995030467727));
#40092=CARTESIAN_POINT('Ctrl Pts',(-0.357052332559036,57.495,-6.94733716327837));
#40093=CARTESIAN_POINT('Ctrl Pts',(-0.357052332559036,49.875,-6.94733716327837));
#40094=CARTESIAN_POINT('Ctrl Pts',(-0.331200384094009,57.495,-6.99500658045299));
#40095=CARTESIAN_POINT('Ctrl Pts',(-0.331200384094009,49.875,-6.99500658045299));
#40096=CARTESIAN_POINT('Ctrl Pts',(-0.304298370266205,57.495,-7.0429523011241));
#40097=CARTESIAN_POINT('Ctrl Pts',(-0.304298370266205,49.875,-7.0429523011241));
#40098=CARTESIAN_POINT('Ctrl Pts',(-0.281943861934841,57.495,-7.0815264936403));
#40099=CARTESIAN_POINT('Ctrl Pts',(-0.281943861934841,49.875,-7.0815264936403));
#40100=CARTESIAN_POINT('Ctrl Pts',(-0.264712515322388,57.495,-7.11057846529273));
#40101=CARTESIAN_POINT('Ctrl Pts',(-0.264712515322388,49.875,-7.11057846529273));
#40102=CARTESIAN_POINT('Ctrl Pts',(-0.253018452443276,57.495,-7.13000027153808));
#40103=CARTESIAN_POINT('Ctrl Pts',(-0.253018452443276,49.875,-7.13000027153808));
#40104=CARTESIAN_POINT('Ctrl Pts',(-0.247119796320918,57.495,-7.13972463098307));
#40105=CARTESIAN_POINT('Ctrl Pts',(-0.247119796320918,49.875,-7.13972463098307));
#40106=CARTESIAN_POINT('',(-0.659304453656788,51.145,-5.93051272372135));
#40107=CARTESIAN_POINT('Ctrl Pts',(-0.659304453656788,51.145,-5.93051272372135));
#40108=CARTESIAN_POINT('Ctrl Pts',(-0.659649967278237,51.145,-5.9344082212537));
#40109=CARTESIAN_POINT('Ctrl Pts',(-0.660242999639202,51.145,-5.94245897164691));
#40110=CARTESIAN_POINT('Ctrl Pts',(-0.660838563360922,51.145,-5.95531437453424));
#40111=CARTESIAN_POINT('Ctrl Pts',(-0.661043615595512,51.145,-5.97401619058907));
#40112=CARTESIAN_POINT('Ctrl Pts',(-0.660311421925998,51.145,-5.99999062205823));
#40113=CARTESIAN_POINT('Ctrl Pts',(-0.658581184594089,51.145,-6.0285167231501));
#40114=CARTESIAN_POINT('Ctrl Pts',(-0.655842009648634,51.145,-6.05948455921138));
#40115=CARTESIAN_POINT('Ctrl Pts',(-0.65208348946162,51.145,-6.09268249742298));
#40116=CARTESIAN_POINT('Ctrl Pts',(-0.647296629738921,51.145,-6.12780215712604));
#40117=CARTESIAN_POINT('Ctrl Pts',(-0.641473544543615,51.145,-6.16449561918676));
#40118=CARTESIAN_POINT('Ctrl Pts',(-0.634607707876565,51.145,-6.20242090374318));
#40119=CARTESIAN_POINT('Ctrl Pts',(-0.626694128202842,51.145,-6.24128706412515));
#40120=CARTESIAN_POINT('Ctrl Pts',(-0.617730009530307,51.145,-6.2809112037544));
#40121=CARTESIAN_POINT('Ctrl Pts',(-0.607714431517402,51.145,-6.32121490697716));
#40122=CARTESIAN_POINT('Ctrl Pts',(-0.596647533682212,51.145,-6.36218460951727));
#40123=CARTESIAN_POINT('Ctrl Pts',(-0.584530087032238,51.145,-6.40384227175352));
#40124=CARTESIAN_POINT('Ctrl Pts',(-0.57136310290558,51.145,-6.44621447382266));
#40125=CARTESIAN_POINT('Ctrl Pts',(-0.557147755196278,51.145,-6.4892958755784));
#40126=CARTESIAN_POINT('Ctrl Pts',(-0.54188492983995,51.145,-6.53304612199323));
#40127=CARTESIAN_POINT('Ctrl Pts',(-0.525574676214357,51.145,-6.57740496530571));
#40128=CARTESIAN_POINT('Ctrl Pts',(-0.508215876982669,51.145,-6.62230172760513));
#40129=CARTESIAN_POINT('Ctrl Pts',(-0.489806088474623,51.145,-6.66766610085618));
#40130=CARTESIAN_POINT('Ctrl Pts',(-0.470341429749656,51.145,-6.71344014059664));
#40131=CARTESIAN_POINT('Ctrl Pts',(-0.44981707848863,51.145,-6.75958168761858));
#40132=CARTESIAN_POINT('Ctrl Pts',(-0.428228256434474,51.145,-6.80606015708966));
#40133=CARTESIAN_POINT('Ctrl Pts',(-0.405571362419757,51.145,-6.85285448604159));
#40134=CARTESIAN_POINT('Ctrl Pts',(-0.381845111328235,51.145,-6.89995030467727));
#40135=CARTESIAN_POINT('Ctrl Pts',(-0.357052332559036,51.145,-6.94733716327837));
#40136=CARTESIAN_POINT('Ctrl Pts',(-0.331200384094009,51.145,-6.99500658045299));
#40137=CARTESIAN_POINT('Ctrl Pts',(-0.304298370266205,51.145,-7.0429523011241));
#40138=CARTESIAN_POINT('Ctrl Pts',(-0.281943861934841,51.145,-7.0815264936403));
#40139=CARTESIAN_POINT('Ctrl Pts',(-0.264712515322388,51.145,-7.11057846529273));
#40140=CARTESIAN_POINT('Ctrl Pts',(-0.253018452443276,51.145,-7.13000027153808));
#40141=CARTESIAN_POINT('Ctrl Pts',(-0.247119796320918,51.145,-7.13972463098307));
#40142=CARTESIAN_POINT('',(-0.659304453656788,57.495,-5.93051272372135));
#40143=CARTESIAN_POINT('Origin',(-0.575436549687219,57.495,-5.17611212951227));
#40144=CARTESIAN_POINT('',(-0.592010183030745,51.145,-5.32519370006274));
#40145=CARTESIAN_POINT('',(-0.592010183030745,54.32,-5.32519370006274));
#40146=CARTESIAN_POINT('',(-0.575436549687219,51.145,-5.17611212951227));
#40147=CARTESIAN_POINT('Ctrl Pts',(0.247119796320915,57.495,-7.13972463098307));
#40148=CARTESIAN_POINT('Ctrl Pts',(0.247119796320915,49.875,-7.13972463098307));
#40149=CARTESIAN_POINT('Ctrl Pts',(0.253018452443265,57.495,-7.13000027153814));
#40150=CARTESIAN_POINT('Ctrl Pts',(0.253018452443265,49.875,-7.13000027153814));
#40151=CARTESIAN_POINT('Ctrl Pts',(0.264712515322363,57.495,-7.1105784652929));
#40152=CARTESIAN_POINT('Ctrl Pts',(0.264712515322363,49.875,-7.1105784652929));
#40153=CARTESIAN_POINT('Ctrl Pts',(0.281943861934803,57.495,-7.0815264936406));
#40154=CARTESIAN_POINT('Ctrl Pts',(0.281943861934803,49.875,-7.0815264936406));
#40155=CARTESIAN_POINT('Ctrl Pts',(0.304298370266162,57.495,-7.04295230112448));
#40156=CARTESIAN_POINT('Ctrl Pts',(0.304298370266162,49.875,-7.04295230112448));
#40157=CARTESIAN_POINT('Ctrl Pts',(0.331200384093974,57.495,-6.99500658045334));
#40158=CARTESIAN_POINT('Ctrl Pts',(0.331200384093974,49.875,-6.99500658045334));
#40159=CARTESIAN_POINT('Ctrl Pts',(0.357052332559016,57.495,-6.94733716327859));
#40160=CARTESIAN_POINT('Ctrl Pts',(0.357052332559016,49.875,-6.94733716327859));
#40161=CARTESIAN_POINT('Ctrl Pts',(0.38184511132823,57.495,-6.89995030467732));
#40162=CARTESIAN_POINT('Ctrl Pts',(0.38184511132823,49.875,-6.89995030467732));
#40163=CARTESIAN_POINT('Ctrl Pts',(0.405571362419761,57.495,-6.85285448604147));
#40164=CARTESIAN_POINT('Ctrl Pts',(0.405571362419761,49.875,-6.85285448604147));
#40165=CARTESIAN_POINT('Ctrl Pts',(0.428228256434481,57.495,-6.80606015708944));
#40166=CARTESIAN_POINT('Ctrl Pts',(0.428228256434481,49.875,-6.80606015708944));
#40167=CARTESIAN_POINT('Ctrl Pts',(0.449817078488634,57.495,-6.75958168761835));
#40168=CARTESIAN_POINT('Ctrl Pts',(0.449817078488634,49.875,-6.75958168761835));
#40169=CARTESIAN_POINT('Ctrl Pts',(0.470341429749655,57.495,-6.71344014059646));
#40170=CARTESIAN_POINT('Ctrl Pts',(0.470341429749655,49.875,-6.71344014059646));
#40171=CARTESIAN_POINT('Ctrl Pts',(0.489806088474619,57.495,-6.66766610085612));
#40172=CARTESIAN_POINT('Ctrl Pts',(0.489806088474619,49.875,-6.66766610085612));
#40173=CARTESIAN_POINT('Ctrl Pts',(0.508215876982667,57.495,-6.62230172760518));
#40174=CARTESIAN_POINT('Ctrl Pts',(0.508215876982667,49.875,-6.62230172760518));
#40175=CARTESIAN_POINT('Ctrl Pts',(0.525574676214359,57.495,-6.57740496530586));
#40176=CARTESIAN_POINT('Ctrl Pts',(0.525574676214359,49.875,-6.57740496530586));
#40177=CARTESIAN_POINT('Ctrl Pts',(0.541884929839957,57.495,-6.53304612199338));
#40178=CARTESIAN_POINT('Ctrl Pts',(0.541884929839957,49.875,-6.53304612199338));
#40179=CARTESIAN_POINT('Ctrl Pts',(0.557147755196286,57.495,-6.48929587557851));
#40180=CARTESIAN_POINT('Ctrl Pts',(0.557147755196286,49.875,-6.48929587557851));
#40181=CARTESIAN_POINT('Ctrl Pts',(0.571363102905584,57.495,-6.4462144738227));
#40182=CARTESIAN_POINT('Ctrl Pts',(0.571363102905584,49.875,-6.4462144738227));
#40183=CARTESIAN_POINT('Ctrl Pts',(0.584530087032233,57.495,-6.40384227175349));
#40184=CARTESIAN_POINT('Ctrl Pts',(0.584530087032233,49.875,-6.40384227175349));
#40185=CARTESIAN_POINT('Ctrl Pts',(0.596647533682195,57.495,-6.36218460951721));
#40186=CARTESIAN_POINT('Ctrl Pts',(0.596647533682195,49.875,-6.36218460951721));
#40187=CARTESIAN_POINT('Ctrl Pts',(0.607714431517377,57.495,-6.32121490697708));
#40188=CARTESIAN_POINT('Ctrl Pts',(0.607714431517377,49.875,-6.32121490697708));
#40189=CARTESIAN_POINT('Ctrl Pts',(0.617730009530282,57.495,-6.28091120375433));
#40190=CARTESIAN_POINT('Ctrl Pts',(0.617730009530282,49.875,-6.28091120375433));
#40191=CARTESIAN_POINT('Ctrl Pts',(0.626694128202827,57.495,-6.24128706412512));
#40192=CARTESIAN_POINT('Ctrl Pts',(0.626694128202827,49.875,-6.24128706412512));
#40193=CARTESIAN_POINT('Ctrl Pts',(0.63460770787657,57.495,-6.2024209037432));
#40194=CARTESIAN_POINT('Ctrl Pts',(0.63460770787657,49.875,-6.2024209037432));
#40195=CARTESIAN_POINT('Ctrl Pts',(0.641473544543642,57.495,-6.16449561918681));
#40196=CARTESIAN_POINT('Ctrl Pts',(0.641473544543642,49.875,-6.16449561918681));
#40197=CARTESIAN_POINT('Ctrl Pts',(0.647296629738964,57.495,-6.12780215712609));
#40198=CARTESIAN_POINT('Ctrl Pts',(0.647296629738964,49.875,-6.12780215712609));
#40199=CARTESIAN_POINT('Ctrl Pts',(0.652083489461663,57.495,-6.092682497423));
#40200=CARTESIAN_POINT('Ctrl Pts',(0.652083489461663,49.875,-6.092682497423));
#40201=CARTESIAN_POINT('Ctrl Pts',(0.655842009648654,57.495,-6.05948455921138));
#40202=CARTESIAN_POINT('Ctrl Pts',(0.655842009648654,49.875,-6.05948455921138));
#40203=CARTESIAN_POINT('Ctrl Pts',(0.658581184594064,57.495,-6.02851672315009));
#40204=CARTESIAN_POINT('Ctrl Pts',(0.658581184594064,49.875,-6.02851672315009));
#40205=CARTESIAN_POINT('Ctrl Pts',(0.660311421925919,57.495,-5.99999062205821));
#40206=CARTESIAN_POINT('Ctrl Pts',(0.660311421925919,49.875,-5.99999062205821));
#40207=CARTESIAN_POINT('Ctrl Pts',(0.661043615595394,57.495,-5.97401619058905));
#40208=CARTESIAN_POINT('Ctrl Pts',(0.661043615595394,49.875,-5.97401619058905));
#40209=CARTESIAN_POINT('Ctrl Pts',(0.660838563360811,57.495,-5.95531437453421));
#40210=CARTESIAN_POINT('Ctrl Pts',(0.660838563360811,49.875,-5.95531437453421));
#40211=CARTESIAN_POINT('Ctrl Pts',(0.660242999639131,57.495,-5.94245897164689));
#40212=CARTESIAN_POINT('Ctrl Pts',(0.660242999639131,49.875,-5.94245897164689));
#40213=CARTESIAN_POINT('Ctrl Pts',(0.659649967278209,57.495,-5.93440822125369));
#40214=CARTESIAN_POINT('Ctrl Pts',(0.659649967278209,49.875,-5.93440822125369));
#40215=CARTESIAN_POINT('Ctrl Pts',(0.659304453656786,57.495,-5.93051272372135));
#40216=CARTESIAN_POINT('Ctrl Pts',(0.659304453656786,49.875,-5.93051272372135));
#40217=CARTESIAN_POINT('Ctrl Pts',(0.247119796320915,51.145,-7.13972463098307));
#40218=CARTESIAN_POINT('Ctrl Pts',(0.253018452443265,51.145,-7.13000027153814));
#40219=CARTESIAN_POINT('Ctrl Pts',(0.264712515322363,51.145,-7.1105784652929));
#40220=CARTESIAN_POINT('Ctrl Pts',(0.281943861934803,51.145,-7.0815264936406));
#40221=CARTESIAN_POINT('Ctrl Pts',(0.304298370266162,51.145,-7.04295230112448));
#40222=CARTESIAN_POINT('Ctrl Pts',(0.331200384093974,51.145,-6.99500658045334));
#40223=CARTESIAN_POINT('Ctrl Pts',(0.357052332559016,51.145,-6.94733716327859));
#40224=CARTESIAN_POINT('Ctrl Pts',(0.38184511132823,51.145,-6.89995030467732));
#40225=CARTESIAN_POINT('Ctrl Pts',(0.405571362419761,51.145,-6.85285448604147));
#40226=CARTESIAN_POINT('Ctrl Pts',(0.428228256434481,51.145,-6.80606015708944));
#40227=CARTESIAN_POINT('Ctrl Pts',(0.449817078488634,51.145,-6.75958168761835));
#40228=CARTESIAN_POINT('Ctrl Pts',(0.470341429749655,51.145,-6.71344014059646));
#40229=CARTESIAN_POINT('Ctrl Pts',(0.489806088474619,51.145,-6.66766610085612));
#40230=CARTESIAN_POINT('Ctrl Pts',(0.508215876982667,51.145,-6.62230172760518));
#40231=CARTESIAN_POINT('Ctrl Pts',(0.525574676214359,51.145,-6.57740496530586));
#40232=CARTESIAN_POINT('Ctrl Pts',(0.541884929839957,51.145,-6.53304612199338));
#40233=CARTESIAN_POINT('Ctrl Pts',(0.557147755196286,51.145,-6.48929587557851));
#40234=CARTESIAN_POINT('Ctrl Pts',(0.571363102905584,51.145,-6.4462144738227));
#40235=CARTESIAN_POINT('Ctrl Pts',(0.584530087032233,51.145,-6.40384227175349));
#40236=CARTESIAN_POINT('Ctrl Pts',(0.596647533682195,51.145,-6.36218460951721));
#40237=CARTESIAN_POINT('Ctrl Pts',(0.607714431517377,51.145,-6.32121490697708));
#40238=CARTESIAN_POINT('Ctrl Pts',(0.617730009530282,51.145,-6.28091120375433));
#40239=CARTESIAN_POINT('Ctrl Pts',(0.626694128202827,51.145,-6.24128706412512));
#40240=CARTESIAN_POINT('Ctrl Pts',(0.63460770787657,51.145,-6.2024209037432));
#40241=CARTESIAN_POINT('Ctrl Pts',(0.641473544543642,51.145,-6.16449561918681));
#40242=CARTESIAN_POINT('Ctrl Pts',(0.647296629738964,51.145,-6.12780215712609));
#40243=CARTESIAN_POINT('Ctrl Pts',(0.652083489461663,51.145,-6.092682497423));
#40244=CARTESIAN_POINT('Ctrl Pts',(0.655842009648654,51.145,-6.05948455921138));
#40245=CARTESIAN_POINT('Ctrl Pts',(0.658581184594064,51.145,-6.02851672315009));
#40246=CARTESIAN_POINT('Ctrl Pts',(0.660311421925919,51.145,-5.99999062205821));
#40247=CARTESIAN_POINT('Ctrl Pts',(0.661043615595394,51.145,-5.97401619058905));
#40248=CARTESIAN_POINT('Ctrl Pts',(0.660838563360811,51.145,-5.95531437453421));
#40249=CARTESIAN_POINT('Ctrl Pts',(0.660242999639131,51.145,-5.94245897164689));
#40250=CARTESIAN_POINT('Ctrl Pts',(0.659649967278209,51.145,-5.93440822125369));
#40251=CARTESIAN_POINT('Ctrl Pts',(0.659304453656786,51.145,-5.93051272372135));
#40252=CARTESIAN_POINT('Origin',(0.,54.32,0.));
#40253=CARTESIAN_POINT('',(-1.4909173120086,51.145,-5.1463899549833));
#40254=CARTESIAN_POINT('Origin',(0.,51.145,0.));
#40255=CARTESIAN_POINT('',(-1.4909173120086,54.32,-5.1463899549833));
#40256=CARTESIAN_POINT('Origin',(-1.66039107437148,57.495,-5.73138421404289));
#40257=CARTESIAN_POINT('',(-1.66039107437148,51.145,-5.73138421404289));
#40258=CARTESIAN_POINT('',(-1.66039107437148,51.145,-5.73138421404289));
#40259=CARTESIAN_POINT('',(-1.66039107437148,57.495,-5.73138421404289));
#40260=CARTESIAN_POINT('Origin',(-6.23660068148933E-13,57.495,-1.50456066262064E-12));
#40261=CARTESIAN_POINT('',(-2.50394540602692,51.145,-6.69081410619341));
#40262=CARTESIAN_POINT('',(-2.50394540602692,57.495,-6.69081410619341));
#40263=CARTESIAN_POINT('',(-2.96056324982543,51.145,-6.5016768024705));
#40264=CARTESIAN_POINT('Origin',(-6.23660068148933E-13,51.145,-1.50456066262064E-12));
#40265=CARTESIAN_POINT('',(-2.96056324982543,57.495,-6.5016768024705));
#40266=CARTESIAN_POINT('Ctrl Pts',(-2.87862685522557,57.495,-5.22677443144495));
#40267=CARTESIAN_POINT('Ctrl Pts',(-2.87862685522557,49.875,-5.22677443144495));
#40268=CARTESIAN_POINT('Ctrl Pts',(-2.88043681055508,57.495,-5.23024117954545));
#40269=CARTESIAN_POINT('Ctrl Pts',(-2.88043681055508,49.875,-5.23024117954545));
#40270=CARTESIAN_POINT('Ctrl Pts',(-2.88406558980908,57.495,-5.2374521593957));
#40271=CARTESIAN_POINT('Ctrl Pts',(-2.88406558980908,49.875,-5.2374521593957));
#40272=CARTESIAN_POINT('Ctrl Pts',(-2.88953536864324,57.495,-5.24910109063627));
#40273=CARTESIAN_POINT('Ctrl Pts',(-2.88953536864324,49.875,-5.24910109063627));
#40274=CARTESIAN_POINT('Ctrl Pts',(-2.8968816873652,57.495,-5.26630084561717));
#40275=CARTESIAN_POINT('Ctrl Pts',(-2.8968816873652,49.875,-5.26630084561717));
#40276=CARTESIAN_POINT('Ctrl Pts',(-2.90614521320845,57.495,-5.29057828960674));
#40277=CARTESIAN_POINT('Ctrl Pts',(-2.90614521320845,49.875,-5.29057828960674));
#40278=CARTESIAN_POINT('Ctrl Pts',(-2.91546314862894,57.495,-5.31759510370885));
#40279=CARTESIAN_POINT('Ctrl Pts',(-2.91546314862894,49.875,-5.31759510370885));
#40280=CARTESIAN_POINT('Ctrl Pts',(-2.92478335875772,57.495,-5.34725389048201));
#40281=CARTESIAN_POINT('Ctrl Pts',(-2.92478335875772,49.875,-5.34725389048201));
#40282=CARTESIAN_POINT('Ctrl Pts',(-2.93401523982666,57.495,-5.37936310952307));
#40283=CARTESIAN_POINT('Ctrl Pts',(-2.93401523982666,49.875,-5.37936310952307));
#40284=CARTESIAN_POINT('Ctrl Pts',(-2.94303247002252,57.495,-5.41364129622042));
#40285=CARTESIAN_POINT('Ctrl Pts',(-2.94303247002252,49.875,-5.41364129622042));
#40286=CARTESIAN_POINT('Ctrl Pts',(-2.95169462080126,57.495,-5.44977003302479));
#40287=CARTESIAN_POINT('Ctrl Pts',(-2.95169462080126,49.875,-5.44977003302479));
#40288=CARTESIAN_POINT('Ctrl Pts',(-2.95986479289848,57.495,-5.48743586913294));
#40289=CARTESIAN_POINT('Ctrl Pts',(-2.95986479289848,49.875,-5.48743586913294));
#40290=CARTESIAN_POINT('Ctrl Pts',(-2.96742703426686,57.495,-5.52637191504897));
#40291=CARTESIAN_POINT('Ctrl Pts',(-2.96742703426686,49.875,-5.52637191504897));
#40292=CARTESIAN_POINT('Ctrl Pts',(-2.97430877025613,57.495,-5.56641026634754));
#40293=CARTESIAN_POINT('Ctrl Pts',(-2.97430877025613,49.875,-5.56641026634754));
#40294=CARTESIAN_POINT('Ctrl Pts',(-2.98047914221005,57.495,-5.60747882861056));
#40295=CARTESIAN_POINT('Ctrl Pts',(-2.98047914221005,49.875,-5.60747882861056));
#40296=CARTESIAN_POINT('Ctrl Pts',(-2.98593308820275,57.495,-5.64956501668965));
#40297=CARTESIAN_POINT('Ctrl Pts',(-2.98593308820275,49.875,-5.64956501668965));
#40298=CARTESIAN_POINT('Ctrl Pts',(-2.99067972442542,57.495,-5.6926888242775));
#40299=CARTESIAN_POINT('Ctrl Pts',(-2.99067972442542,49.875,-5.6926888242775));
#40300=CARTESIAN_POINT('Ctrl Pts',(-2.99473015701058,57.495,-5.7368744211961));
#40301=CARTESIAN_POINT('Ctrl Pts',(-2.99473015701058,49.875,-5.7368744211961));
#40302=CARTESIAN_POINT('Ctrl Pts',(-2.99808342690941,57.495,-5.78211642456377));
#40303=CARTESIAN_POINT('Ctrl Pts',(-2.99808342690941,49.875,-5.78211642456377));
#40304=CARTESIAN_POINT('Ctrl Pts',(-3.00072490941925,57.495,-5.82837721216372));
#40305=CARTESIAN_POINT('Ctrl Pts',(-3.00072490941925,49.875,-5.82837721216372));
#40306=CARTESIAN_POINT('Ctrl Pts',(-3.00263159433907,57.495,-5.87560110342618));
#40307=CARTESIAN_POINT('Ctrl Pts',(-3.00263159433907,49.875,-5.87560110342618));
#40308=CARTESIAN_POINT('Ctrl Pts',(-3.00377540211876,57.495,-5.92372322806235));
#40309=CARTESIAN_POINT('Ctrl Pts',(-3.00377540211876,49.875,-5.92372322806235));
#40310=CARTESIAN_POINT('Ctrl Pts',(-3.00412716938111,57.495,-5.97267956506957));
#40311=CARTESIAN_POINT('Ctrl Pts',(-3.00412716938111,49.875,-5.97267956506957));
#40312=CARTESIAN_POINT('Ctrl Pts',(-3.00366113621889,57.495,-6.02241806591683));
#40313=CARTESIAN_POINT('Ctrl Pts',(-3.00366113621889,49.875,-6.02241806591683));
#40314=CARTESIAN_POINT('Ctrl Pts',(-3.00235671375975,57.495,-6.07290162599645));
#40315=CARTESIAN_POINT('Ctrl Pts',(-3.00235671375975,49.875,-6.07290162599645));
#40316=CARTESIAN_POINT('Ctrl Pts',(-3.00019778316116,57.495,-6.12410381716763));
#40317=CARTESIAN_POINT('Ctrl Pts',(-3.00019778316116,49.875,-6.12410381716763));
#40318=CARTESIAN_POINT('Ctrl Pts',(-2.99717295692923,57.495,-6.1760065578922));
#40319=CARTESIAN_POINT('Ctrl Pts',(-2.99717295692923,49.875,-6.1760065578922));
#40320=CARTESIAN_POINT('Ctrl Pts',(-2.9932755486881,57.495,-6.22859706400143));
#40321=CARTESIAN_POINT('Ctrl Pts',(-2.9932755486881,49.875,-6.22859706400143));
#40322=CARTESIAN_POINT('Ctrl Pts',(-2.98850417352762,57.495,-6.28186459845025));
#40323=CARTESIAN_POINT('Ctrl Pts',(-2.98850417352762,49.875,-6.28186459845025));
#40324=CARTESIAN_POINT('Ctrl Pts',(-2.98286238364847,57.495,-6.33579850967655));
#40325=CARTESIAN_POINT('Ctrl Pts',(-2.98286238364847,49.875,-6.33579850967655));
#40326=CARTESIAN_POINT('Ctrl Pts',(-2.97635619664327,57.495,-6.39038953466525));
#40327=CARTESIAN_POINT('Ctrl Pts',(-2.97635619664327,49.875,-6.39038953466525));
#40328=CARTESIAN_POINT('Ctrl Pts',(-2.97046502832937,57.495,-6.43458214159119));
#40329=CARTESIAN_POINT('Ctrl Pts',(-2.97046502832937,49.875,-6.43458214159119));
#40330=CARTESIAN_POINT('Ctrl Pts',(-2.96566304810545,57.495,-6.4680168144459));
#40331=CARTESIAN_POINT('Ctrl Pts',(-2.96566304810545,49.875,-6.4680168144459));
#40332=CARTESIAN_POINT('Ctrl Pts',(-2.96229154623624,57.495,-6.49043534784125));
#40333=CARTESIAN_POINT('Ctrl Pts',(-2.96229154623624,49.875,-6.49043534784125));
#40334=CARTESIAN_POINT('Ctrl Pts',(-2.96056324982543,57.495,-6.5016768024705));
#40335=CARTESIAN_POINT('Ctrl Pts',(-2.96056324982543,49.875,-6.5016768024705));
#40336=CARTESIAN_POINT('',(-2.87862685522557,51.145,-5.22677443144495));
#40337=CARTESIAN_POINT('Ctrl Pts',(-2.87862685522557,51.145,-5.22677443144495));
#40338=CARTESIAN_POINT('Ctrl Pts',(-2.88043681055508,51.145,-5.23024117954545));
#40339=CARTESIAN_POINT('Ctrl Pts',(-2.88406558980908,51.145,-5.2374521593957));
#40340=CARTESIAN_POINT('Ctrl Pts',(-2.88953536864324,51.145,-5.24910109063627));
#40341=CARTESIAN_POINT('Ctrl Pts',(-2.8968816873652,51.145,-5.26630084561717));
#40342=CARTESIAN_POINT('Ctrl Pts',(-2.90614521320845,51.145,-5.29057828960674));
#40343=CARTESIAN_POINT('Ctrl Pts',(-2.91546314862894,51.145,-5.31759510370885));
#40344=CARTESIAN_POINT('Ctrl Pts',(-2.92478335875772,51.145,-5.34725389048201));
#40345=CARTESIAN_POINT('Ctrl Pts',(-2.93401523982666,51.145,-5.37936310952307));
#40346=CARTESIAN_POINT('Ctrl Pts',(-2.94303247002252,51.145,-5.41364129622042));
#40347=CARTESIAN_POINT('Ctrl Pts',(-2.95169462080126,51.145,-5.44977003302479));
#40348=CARTESIAN_POINT('Ctrl Pts',(-2.95986479289848,51.145,-5.48743586913294));
#40349=CARTESIAN_POINT('Ctrl Pts',(-2.96742703426686,51.145,-5.52637191504897));
#40350=CARTESIAN_POINT('Ctrl Pts',(-2.97430877025613,51.145,-5.56641026634754));
#40351=CARTESIAN_POINT('Ctrl Pts',(-2.98047914221005,51.145,-5.60747882861056));
#40352=CARTESIAN_POINT('Ctrl Pts',(-2.98593308820275,51.145,-5.64956501668965));
#40353=CARTESIAN_POINT('Ctrl Pts',(-2.99067972442542,51.145,-5.6926888242775));
#40354=CARTESIAN_POINT('Ctrl Pts',(-2.99473015701058,51.145,-5.7368744211961));
#40355=CARTESIAN_POINT('Ctrl Pts',(-2.99808342690941,51.145,-5.78211642456377));
#40356=CARTESIAN_POINT('Ctrl Pts',(-3.00072490941925,51.145,-5.82837721216372));
#40357=CARTESIAN_POINT('Ctrl Pts',(-3.00263159433907,51.145,-5.87560110342618));
#40358=CARTESIAN_POINT('Ctrl Pts',(-3.00377540211876,51.145,-5.92372322806235));
#40359=CARTESIAN_POINT('Ctrl Pts',(-3.00412716938111,51.145,-5.97267956506957));
#40360=CARTESIAN_POINT('Ctrl Pts',(-3.00366113621889,51.145,-6.02241806591683));
#40361=CARTESIAN_POINT('Ctrl Pts',(-3.00235671375975,51.145,-6.07290162599645));
#40362=CARTESIAN_POINT('Ctrl Pts',(-3.00019778316116,51.145,-6.12410381716763));
#40363=CARTESIAN_POINT('Ctrl Pts',(-2.99717295692923,51.145,-6.1760065578922));
#40364=CARTESIAN_POINT('Ctrl Pts',(-2.9932755486881,51.145,-6.22859706400143));
#40365=CARTESIAN_POINT('Ctrl Pts',(-2.98850417352762,51.145,-6.28186459845025));
#40366=CARTESIAN_POINT('Ctrl Pts',(-2.98286238364847,51.145,-6.33579850967655));
#40367=CARTESIAN_POINT('Ctrl Pts',(-2.97635619664327,51.145,-6.39038953466525));
#40368=CARTESIAN_POINT('Ctrl Pts',(-2.97046502832937,51.145,-6.43458214159119));
#40369=CARTESIAN_POINT('Ctrl Pts',(-2.96566304810545,51.145,-6.4680168144459));
#40370=CARTESIAN_POINT('Ctrl Pts',(-2.96229154623624,51.145,-6.49043534784125));
#40371=CARTESIAN_POINT('Ctrl Pts',(-2.96056324982543,51.145,-6.5016768024705));
#40372=CARTESIAN_POINT('',(-2.87862685522557,57.495,-5.22677443144495));
#40373=CARTESIAN_POINT('Origin',(-2.51244640654327,57.495,-4.56189402049717));
#40374=CARTESIAN_POINT('',(-2.58480949428933,51.145,-4.69328497730872));
#40375=CARTESIAN_POINT('',(-2.58480949428933,54.32,-4.69328497730872));
#40376=CARTESIAN_POINT('',(-2.51244640654327,51.145,-4.56189402049717));
#40377=CARTESIAN_POINT('Ctrl Pts',(-2.50394540602692,57.495,-6.69081410619341));
#40378=CARTESIAN_POINT('Ctrl Pts',(-2.50394540602692,49.875,-6.69081410619341));
#40379=CARTESIAN_POINT('Ctrl Pts',(-2.49477440711622,57.495,-6.6840872875067));
#40380=CARTESIAN_POINT('Ctrl Pts',(-2.49477440711622,49.875,-6.6840872875067));
#40381=CARTESIAN_POINT('Ctrl Pts',(-2.47653809829367,57.495,-6.67061900235319));
#40382=CARTESIAN_POINT('Ctrl Pts',(-2.47653809829367,49.875,-6.67061900235319));
#40383=CARTESIAN_POINT('Ctrl Pts',(-2.44950070161195,57.495,-6.65037263123044));
#40384=CARTESIAN_POINT('Ctrl Pts',(-2.44950070161195,49.875,-6.65037263123044));
#40385=CARTESIAN_POINT('Ctrl Pts',(-2.41408612451247,57.495,-6.62328942425873));
#40386=CARTESIAN_POINT('Ctrl Pts',(-2.41408612451247,49.875,-6.62328942425873));
#40387=CARTESIAN_POINT('Ctrl Pts',(-2.37088387159997,57.495,-6.58928830924833));
#40388=CARTESIAN_POINT('Ctrl Pts',(-2.37088387159997,49.875,-6.58928830924833));
#40389=CARTESIAN_POINT('Ctrl Pts',(-2.32875748935431,57.495,-6.55514062276576));
#40390=CARTESIAN_POINT('Ctrl Pts',(-2.32875748935431,49.875,-6.55514062276576));
#40391=CARTESIAN_POINT('Ctrl Pts',(-2.28771778279682,57.495,-6.52084865967131));
#40392=CARTESIAN_POINT('Ctrl Pts',(-2.28771778279682,49.875,-6.52084865967131));
#40393=CARTESIAN_POINT('Ctrl Pts',(-2.24777479550452,57.495,-6.48641743997165));
#40394=CARTESIAN_POINT('Ctrl Pts',(-2.24777479550452,49.875,-6.48641743997165));
#40395=CARTESIAN_POINT('Ctrl Pts',(-2.20893514043546,57.495,-6.45185553518355));
#40396=CARTESIAN_POINT('Ctrl Pts',(-2.20893514043546,49.875,-6.45185553518355));
#40397=CARTESIAN_POINT('Ctrl Pts',(-2.17120312938032,57.495,-6.41717671306116));
#40398=CARTESIAN_POINT('Ctrl Pts',(-2.17120312938032,49.875,-6.41717671306116));
#40399=CARTESIAN_POINT('Ctrl Pts',(-2.13458349574322,57.495,-6.38240181135686));
#40400=CARTESIAN_POINT('Ctrl Pts',(-2.13458349574322,49.875,-6.38240181135686));
#40401=CARTESIAN_POINT('Ctrl Pts',(-2.09908352929886,57.495,-6.34756091533109));
#40402=CARTESIAN_POINT('Ctrl Pts',(-2.09908352929886,49.875,-6.34756091533109));
#40403=CARTESIAN_POINT('Ctrl Pts',(-2.06471490843566,57.495,-6.31269482043472));
#40404=CARTESIAN_POINT('Ctrl Pts',(-2.06471490843566,49.875,-6.31269482043472));
#40405=CARTESIAN_POINT('Ctrl Pts',(-2.03149622201774,57.495,-6.27785854554207));
#40406=CARTESIAN_POINT('Ctrl Pts',(-2.03149622201774,49.875,-6.27785854554207));
#40407=CARTESIAN_POINT('Ctrl Pts',(-1.99945211810842,57.495,-6.24311798195999));
#40408=CARTESIAN_POINT('Ctrl Pts',(-1.99945211810842,49.875,-6.24311798195999));
#40409=CARTESIAN_POINT('Ctrl Pts',(-1.96860861168855,57.495,-6.20853885514991));
#40410=CARTESIAN_POINT('Ctrl Pts',(-1.96860861168855,49.875,-6.20853885514991));
#40411=CARTESIAN_POINT('Ctrl Pts',(-1.93898880419738,57.495,-6.17417680788948));
#40412=CARTESIAN_POINT('Ctrl Pts',(-1.93898880419738,49.875,-6.17417680788948));
#40413=CARTESIAN_POINT('Ctrl Pts',(-1.91060895733316,57.495,-6.14006878432979));
#40414=CARTESIAN_POINT('Ctrl Pts',(-1.91060895733316,49.875,-6.14006878432979));
#40415=CARTESIAN_POINT('Ctrl Pts',(-1.88347219921807,57.495,-6.10621926889293));
#40416=CARTESIAN_POINT('Ctrl Pts',(-1.88347219921807,49.875,-6.10621926889293));
#40417=CARTESIAN_POINT('Ctrl Pts',(-1.85756929242873,57.495,-6.07260331771224));
#40418=CARTESIAN_POINT('Ctrl Pts',(-1.85756929242873,49.875,-6.07260331771224));
#40419=CARTESIAN_POINT('Ctrl Pts',(-1.83289254541003,57.495,-6.03920034699142));
#40420=CARTESIAN_POINT('Ctrl Pts',(-1.83289254541003,49.875,-6.03920034699142));
#40421=CARTESIAN_POINT('Ctrl Pts',(-1.80944727788364,57.495,-6.00602283509636));
#40422=CARTESIAN_POINT('Ctrl Pts',(-1.80944727788364,49.875,-6.00602283509636));
#40423=CARTESIAN_POINT('Ctrl Pts',(-1.78726264793637,57.495,-5.97314358084405));
#40424=CARTESIAN_POINT('Ctrl Pts',(-1.78726264793637,49.875,-5.97314358084405));
#40425=CARTESIAN_POINT('Ctrl Pts',(-1.76640606389863,57.495,-5.94073262861954));
#40426=CARTESIAN_POINT('Ctrl Pts',(-1.76640606389863,49.875,-5.94073262861954));
#40427=CARTESIAN_POINT('Ctrl Pts',(-1.74698425466385,57.495,-5.90906068827417));
#40428=CARTESIAN_POINT('Ctrl Pts',(-1.74698425466385,49.875,-5.90906068827417));
#40429=CARTESIAN_POINT('Ctrl Pts',(-1.72912206102237,57.495,-5.87844620539466));
#40430=CARTESIAN_POINT('Ctrl Pts',(-1.72912206102237,49.875,-5.87844620539466));
#40431=CARTESIAN_POINT('Ctrl Pts',(-1.71294534020681,57.495,-5.84921363316514));
#40432=CARTESIAN_POINT('Ctrl Pts',(-1.71294534020681,49.875,-5.84921363316514));
#40433=CARTESIAN_POINT('Ctrl Pts',(-1.69856379474193,57.495,-5.8216513201319));
#40434=CARTESIAN_POINT('Ctrl Pts',(-1.69856379474193,49.875,-5.8216513201319));
#40435=CARTESIAN_POINT('Ctrl Pts',(-1.68604879760681,57.495,-5.79595877235173));
#40436=CARTESIAN_POINT('Ctrl Pts',(-1.68604879760681,49.875,-5.79595877235173));
#40437=CARTESIAN_POINT('Ctrl Pts',(-1.67543235427339,57.495,-5.77224172513534));
#40438=CARTESIAN_POINT('Ctrl Pts',(-1.67543235427339,49.875,-5.77224172513534));
#40439=CARTESIAN_POINT('Ctrl Pts',(-1.66846492267669,57.495,-5.75488502996854));
#40440=CARTESIAN_POINT('Ctrl Pts',(-1.66846492267669,49.875,-5.75488502996854));
#40441=CARTESIAN_POINT('Ctrl Pts',(-1.66409560210811,57.495,-5.74278027398956));
#40442=CARTESIAN_POINT('Ctrl Pts',(-1.66409560210811,49.875,-5.74278027398956));
#40443=CARTESIAN_POINT('Ctrl Pts',(-1.66156260377489,57.495,-5.73511540682054));
#40444=CARTESIAN_POINT('Ctrl Pts',(-1.66156260377489,49.875,-5.73511540682054));
#40445=CARTESIAN_POINT('Ctrl Pts',(-1.66039107437148,57.495,-5.73138421404289));
#40446=CARTESIAN_POINT('Ctrl Pts',(-1.66039107437148,49.875,-5.73138421404289));
#40447=CARTESIAN_POINT('Ctrl Pts',(-2.50394540602692,51.145,-6.69081410619341));
#40448=CARTESIAN_POINT('Ctrl Pts',(-2.49477440711622,51.145,-6.6840872875067));
#40449=CARTESIAN_POINT('Ctrl Pts',(-2.47653809829367,51.145,-6.67061900235319));
#40450=CARTESIAN_POINT('Ctrl Pts',(-2.44950070161195,51.145,-6.65037263123044));
#40451=CARTESIAN_POINT('Ctrl Pts',(-2.41408612451247,51.145,-6.62328942425873));
#40452=CARTESIAN_POINT('Ctrl Pts',(-2.37088387159997,51.145,-6.58928830924833));
#40453=CARTESIAN_POINT('Ctrl Pts',(-2.32875748935431,51.145,-6.55514062276576));
#40454=CARTESIAN_POINT('Ctrl Pts',(-2.28771778279682,51.145,-6.52084865967131));
#40455=CARTESIAN_POINT('Ctrl Pts',(-2.24777479550452,51.145,-6.48641743997165));
#40456=CARTESIAN_POINT('Ctrl Pts',(-2.20893514043546,51.145,-6.45185553518355));
#40457=CARTESIAN_POINT('Ctrl Pts',(-2.17120312938032,51.145,-6.41717671306116));
#40458=CARTESIAN_POINT('Ctrl Pts',(-2.13458349574322,51.145,-6.38240181135686));
#40459=CARTESIAN_POINT('Ctrl Pts',(-2.09908352929886,51.145,-6.34756091533109));
#40460=CARTESIAN_POINT('Ctrl Pts',(-2.06471490843566,51.145,-6.31269482043472));
#40461=CARTESIAN_POINT('Ctrl Pts',(-2.03149622201774,51.145,-6.27785854554207));
#40462=CARTESIAN_POINT('Ctrl Pts',(-1.99945211810842,51.145,-6.24311798195999));
#40463=CARTESIAN_POINT('Ctrl Pts',(-1.96860861168855,51.145,-6.20853885514991));
#40464=CARTESIAN_POINT('Ctrl Pts',(-1.93898880419738,51.145,-6.17417680788948));
#40465=CARTESIAN_POINT('Ctrl Pts',(-1.91060895733316,51.145,-6.14006878432979));
#40466=CARTESIAN_POINT('Ctrl Pts',(-1.88347219921807,51.145,-6.10621926889293));
#40467=CARTESIAN_POINT('Ctrl Pts',(-1.85756929242873,51.145,-6.07260331771224));
#40468=CARTESIAN_POINT('Ctrl Pts',(-1.83289254541003,51.145,-6.03920034699142));
#40469=CARTESIAN_POINT('Ctrl Pts',(-1.80944727788364,51.145,-6.00602283509636));
#40470=CARTESIAN_POINT('Ctrl Pts',(-1.78726264793637,51.145,-5.97314358084405));
#40471=CARTESIAN_POINT('Ctrl Pts',(-1.76640606389863,51.145,-5.94073262861954));
#40472=CARTESIAN_POINT('Ctrl Pts',(-1.74698425466385,51.145,-5.90906068827417));
#40473=CARTESIAN_POINT('Ctrl Pts',(-1.72912206102237,51.145,-5.87844620539466));
#40474=CARTESIAN_POINT('Ctrl Pts',(-1.71294534020681,51.145,-5.84921363316514));
#40475=CARTESIAN_POINT('Ctrl Pts',(-1.69856379474193,51.145,-5.8216513201319));
#40476=CARTESIAN_POINT('Ctrl Pts',(-1.68604879760681,51.145,-5.79595877235173));
#40477=CARTESIAN_POINT('Ctrl Pts',(-1.67543235427339,51.145,-5.77224172513534));
#40478=CARTESIAN_POINT('Ctrl Pts',(-1.66846492267669,51.145,-5.75488502996854));
#40479=CARTESIAN_POINT('Ctrl Pts',(-1.66409560210811,51.145,-5.74278027398956));
#40480=CARTESIAN_POINT('Ctrl Pts',(-1.66156260377489,51.145,-5.73511540682054));
#40481=CARTESIAN_POINT('Ctrl Pts',(-1.66039107437148,51.145,-5.73138421404289));
#40482=CARTESIAN_POINT('Origin',(0.,54.32,0.));
#40483=CARTESIAN_POINT('',(-3.34686616149372,51.145,-4.18409499139877));
#40484=CARTESIAN_POINT('Origin',(0.,51.145,0.));
#40485=CARTESIAN_POINT('',(-3.34686616149372,54.32,-4.18409499139877));
#40486=CARTESIAN_POINT('Origin',(-3.72730711280926,57.495,-4.65970441290367));
#40487=CARTESIAN_POINT('',(-3.72730711280926,51.145,-4.65970441290367));
#40488=CARTESIAN_POINT('',(-3.72730711280926,51.145,-4.65970441290367));
#40489=CARTESIAN_POINT('',(-3.72730711280926,57.495,-4.65970441290367));
#40490=CARTESIAN_POINT('Origin',(-1.15195721078055E-12,57.495,-1.15136842610855E-12));
#40491=CARTESIAN_POINT('',(-4.87380761862879,51.145,-5.22328778611671));
#40492=CARTESIAN_POINT('',(-4.87380761862879,57.495,-5.22328778611671));
#40493=CARTESIAN_POINT('',(-5.22328778611671,51.145,-4.87380761862879));
#40494=CARTESIAN_POINT('Origin',(-1.15195721078055E-12,51.145,-1.15136842610855E-12));
#40495=CARTESIAN_POINT('',(-5.22328778611671,57.495,-4.87380761862879));
#40496=CARTESIAN_POINT('Ctrl Pts',(-4.65970441290367,57.495,-3.72730711280926));
#40497=CARTESIAN_POINT('Ctrl Pts',(-4.65970441290367,49.875,-3.72730711280926));
#40498=CARTESIAN_POINT('Ctrl Pts',(-4.66270326064961,57.495,-3.72981733050576));
#40499=CARTESIAN_POINT('Ctrl Pts',(-4.66270326064961,49.875,-3.72981733050576));
#40500=CARTESIAN_POINT('Ctrl Pts',(-4.6688153380502,57.495,-3.73509073349854));
#40501=CARTESIAN_POINT('Ctrl Pts',(-4.6688153380502,49.875,-3.73509073349854));
#40502=CARTESIAN_POINT('Ctrl Pts',(-4.67832660775297,57.495,-3.7437597489088));
#40503=CARTESIAN_POINT('Ctrl Pts',(-4.67832660775297,49.875,-3.7437597489088));
#40504=CARTESIAN_POINT('Ctrl Pts',(-4.69169578253142,57.495,-3.7568389360361));
#40505=CARTESIAN_POINT('Ctrl Pts',(-4.69169578253142,49.875,-3.7568389360361));
#40506=CARTESIAN_POINT('Ctrl Pts',(-4.70954474005187,57.495,-3.77572337177426));
#40507=CARTESIAN_POINT('Ctrl Pts',(-4.70954474005187,49.875,-3.77572337177426));
#40508=CARTESIAN_POINT('Ctrl Pts',(-4.72849227702429,57.495,-3.79711783384759));
#40509=CARTESIAN_POINT('Ctrl Pts',(-4.72849227702429,49.875,-3.79711783384759));
#40510=CARTESIAN_POINT('Ctrl Pts',(-4.74845295472311,57.495,-3.82095228990398));
#40511=CARTESIAN_POINT('Ctrl Pts',(-4.74845295472311,49.875,-3.82095228990398));
#40512=CARTESIAN_POINT('Ctrl Pts',(-4.76926976684248,57.495,-3.84708445224628));
#40513=CARTESIAN_POINT('Ctrl Pts',(-4.76926976684248,49.875,-3.84708445224628));
#40514=CARTESIAN_POINT('Ctrl Pts',(-4.79071829540097,57.495,-3.87530262274579));
#40515=CARTESIAN_POINT('Ctrl Pts',(-4.79071829540097,49.875,-3.87530262274579));
#40516=CARTESIAN_POINT('Ctrl Pts',(-4.81254694822028,57.495,-3.90536636162316));
#40517=CARTESIAN_POINT('Ctrl Pts',(-4.81254694822028,49.875,-3.90536636162316));
#40518=CARTESIAN_POINT('Ctrl Pts',(-4.83450929444277,57.495,-3.93703846717723));
#40519=CARTESIAN_POINT('Ctrl Pts',(-4.83450929444277,49.875,-3.93703846717723));
#40520=CARTESIAN_POINT('Ctrl Pts',(-4.85639607415679,57.495,-3.97011673859275));
#40521=CARTESIAN_POINT('Ctrl Pts',(-4.85639607415679,49.875,-3.97011673859275));
#40522=CARTESIAN_POINT('Ctrl Pts',(-4.8780759828866,57.495,-4.00447382552398));
#40523=CARTESIAN_POINT('Ctrl Pts',(-4.8780759828866,49.875,-4.00447382552398));
#40524=CARTESIAN_POINT('Ctrl Pts',(-4.89949292161193,57.495,-4.04005493051016));
#40525=CARTESIAN_POINT('Ctrl Pts',(-4.89949292161193,49.875,-4.04005493051016));
#40526=CARTESIAN_POINT('Ctrl Pts',(-4.92063739759527,57.495,-4.07685036350543));
#40527=CARTESIAN_POINT('Ctrl Pts',(-4.92063739759527,49.875,-4.07685036350543));
#40528=CARTESIAN_POINT('Ctrl Pts',(-4.94152548435404,57.495,-4.11487510765792));
#40529=CARTESIAN_POINT('Ctrl Pts',(-4.94152548435404,49.875,-4.11487510765792));
#40530=CARTESIAN_POINT('Ctrl Pts',(-4.9621766920072,57.495,-4.15414724283855));
#40531=CARTESIAN_POINT('Ctrl Pts',(-4.9621766920072,49.875,-4.15414724283855));
#40532=CARTESIAN_POINT('Ctrl Pts',(-4.98258807456953,57.495,-4.19466216292523));
#40533=CARTESIAN_POINT('Ctrl Pts',(-4.98258807456953,49.875,-4.19466216292523));
#40534=CARTESIAN_POINT('Ctrl Pts',(-5.00273172317852,57.495,-4.23639070615327));
#40535=CARTESIAN_POINT('Ctrl Pts',(-5.00273172317852,49.875,-4.23639070615327));
#40536=CARTESIAN_POINT('Ctrl Pts',(-5.02256507114883,57.495,-4.27929023600664));
#40537=CARTESIAN_POINT('Ctrl Pts',(-5.02256507114883,49.875,-4.27929023600664));
#40538=CARTESIAN_POINT('Ctrl Pts',(-5.04203735157409,57.495,-4.32331156573186));
#40539=CARTESIAN_POINT('Ctrl Pts',(-5.04203735157409,49.875,-4.32331156573186));
#40540=CARTESIAN_POINT('Ctrl Pts',(-5.06109712122993,57.495,-4.36840670797621));
#40541=CARTESIAN_POINT('Ctrl Pts',(-5.06109712122993,49.875,-4.36840670797621));
#40542=CARTESIAN_POINT('Ctrl Pts',(-5.07970066295481,57.495,-4.41453743405689));
#40543=CARTESIAN_POINT('Ctrl Pts',(-5.07970066295481,49.875,-4.41453743405689));
#40544=CARTESIAN_POINT('Ctrl Pts',(-5.09781475579234,57.495,-4.46167734280668));
#40545=CARTESIAN_POINT('Ctrl Pts',(-5.09781475579234,49.875,-4.46167734280668));
#40546=CARTESIAN_POINT('Ctrl Pts',(-5.11541439426219,57.495,-4.50980818622117));
#40547=CARTESIAN_POINT('Ctrl Pts',(-5.11541439426219,49.875,-4.50980818622117));
#40548=CARTESIAN_POINT('Ctrl Pts',(-5.13248213818673,57.495,-4.55891761694258));
#40549=CARTESIAN_POINT('Ctrl Pts',(-5.13248213818673,49.875,-4.55891761694258));
#40550=CARTESIAN_POINT('Ctrl Pts',(-5.14900691787061,57.495,-4.60899638270436));
#40551=CARTESIAN_POINT('Ctrl Pts',(-5.14900691787061,49.875,-4.60899638270436));
#40552=CARTESIAN_POINT('Ctrl Pts',(-5.16498334493441,57.495,-4.66003509375248));
#40553=CARTESIAN_POINT('Ctrl Pts',(-5.16498334493441,49.875,-4.66003509375248));
#40554=CARTESIAN_POINT('Ctrl Pts',(-5.1804106250073,57.495,-4.71202254995837));
#40555=CARTESIAN_POINT('Ctrl Pts',(-5.1804106250073,49.875,-4.71202254995837));
#40556=CARTESIAN_POINT('Ctrl Pts',(-5.1952907728175,57.495,-4.764947890579));
#40557=CARTESIAN_POINT('Ctrl Pts',(-5.1952907728175,49.875,-4.764947890579));
#40558=CARTESIAN_POINT('Ctrl Pts',(-5.2067598214933,57.495,-4.8080309881172));
#40559=CARTESIAN_POINT('Ctrl Pts',(-5.2067598214933,49.875,-4.8080309881172));
#40560=CARTESIAN_POINT('Ctrl Pts',(-5.21511826561693,57.495,-4.84075823631811));
#40561=CARTESIAN_POINT('Ctrl Pts',(-5.21511826561693,49.875,-4.84075823631811));
#40562=CARTESIAN_POINT('Ctrl Pts',(-5.22058260535447,57.495,-4.86276047837853));
#40563=CARTESIAN_POINT('Ctrl Pts',(-5.22058260535447,49.875,-4.86276047837853));
#40564=CARTESIAN_POINT('Ctrl Pts',(-5.22328778611671,57.495,-4.87380761862879));
#40565=CARTESIAN_POINT('Ctrl Pts',(-5.22328778611671,49.875,-4.87380761862879));
#40566=CARTESIAN_POINT('',(-4.65970441290367,51.145,-3.72730711280926));
#40567=CARTESIAN_POINT('Ctrl Pts',(-4.65970441290367,51.145,-3.72730711280926));
#40568=CARTESIAN_POINT('Ctrl Pts',(-4.66270326064961,51.145,-3.72981733050576));
#40569=CARTESIAN_POINT('Ctrl Pts',(-4.6688153380502,51.145,-3.73509073349854));
#40570=CARTESIAN_POINT('Ctrl Pts',(-4.67832660775297,51.145,-3.7437597489088));
#40571=CARTESIAN_POINT('Ctrl Pts',(-4.69169578253142,51.145,-3.7568389360361));
#40572=CARTESIAN_POINT('Ctrl Pts',(-4.70954474005187,51.145,-3.77572337177426));
#40573=CARTESIAN_POINT('Ctrl Pts',(-4.72849227702429,51.145,-3.79711783384759));
#40574=CARTESIAN_POINT('Ctrl Pts',(-4.74845295472311,51.145,-3.82095228990398));
#40575=CARTESIAN_POINT('Ctrl Pts',(-4.76926976684248,51.145,-3.84708445224628));
#40576=CARTESIAN_POINT('Ctrl Pts',(-4.79071829540097,51.145,-3.87530262274579));
#40577=CARTESIAN_POINT('Ctrl Pts',(-4.81254694822028,51.145,-3.90536636162316));
#40578=CARTESIAN_POINT('Ctrl Pts',(-4.83450929444277,51.145,-3.93703846717723));
#40579=CARTESIAN_POINT('Ctrl Pts',(-4.85639607415679,51.145,-3.97011673859275));
#40580=CARTESIAN_POINT('Ctrl Pts',(-4.8780759828866,51.145,-4.00447382552398));
#40581=CARTESIAN_POINT('Ctrl Pts',(-4.89949292161193,51.145,-4.04005493051016));
#40582=CARTESIAN_POINT('Ctrl Pts',(-4.92063739759527,51.145,-4.07685036350543));
#40583=CARTESIAN_POINT('Ctrl Pts',(-4.94152548435404,51.145,-4.11487510765792));
#40584=CARTESIAN_POINT('Ctrl Pts',(-4.9621766920072,51.145,-4.15414724283855));
#40585=CARTESIAN_POINT('Ctrl Pts',(-4.98258807456953,51.145,-4.19466216292523));
#40586=CARTESIAN_POINT('Ctrl Pts',(-5.00273172317852,51.145,-4.23639070615327));
#40587=CARTESIAN_POINT('Ctrl Pts',(-5.02256507114883,51.145,-4.27929023600664));
#40588=CARTESIAN_POINT('Ctrl Pts',(-5.04203735157409,51.145,-4.32331156573186));
#40589=CARTESIAN_POINT('Ctrl Pts',(-5.06109712122993,51.145,-4.36840670797621));
#40590=CARTESIAN_POINT('Ctrl Pts',(-5.07970066295481,51.145,-4.41453743405689));
#40591=CARTESIAN_POINT('Ctrl Pts',(-5.09781475579234,51.145,-4.46167734280668));
#40592=CARTESIAN_POINT('Ctrl Pts',(-5.11541439426219,51.145,-4.50980818622117));
#40593=CARTESIAN_POINT('Ctrl Pts',(-5.13248213818673,51.145,-4.55891761694258));
#40594=CARTESIAN_POINT('Ctrl Pts',(-5.14900691787061,51.145,-4.60899638270436));
#40595=CARTESIAN_POINT('Ctrl Pts',(-5.16498334493441,51.145,-4.66003509375248));
#40596=CARTESIAN_POINT('Ctrl Pts',(-5.1804106250073,51.145,-4.71202254995837));
#40597=CARTESIAN_POINT('Ctrl Pts',(-5.1952907728175,51.145,-4.764947890579));
#40598=CARTESIAN_POINT('Ctrl Pts',(-5.2067598214933,51.145,-4.8080309881172));
#40599=CARTESIAN_POINT('Ctrl Pts',(-5.21511826561693,51.145,-4.84075823631811));
#40600=CARTESIAN_POINT('Ctrl Pts',(-5.22058260535447,51.145,-4.86276047837853));
#40601=CARTESIAN_POINT('Ctrl Pts',(-5.22328778611671,51.145,-4.87380761862879));
#40602=CARTESIAN_POINT('',(-4.65970441290367,57.495,-3.72730711280926));
#40603=CARTESIAN_POINT('Origin',(-4.06695907338649,57.495,-3.25316890053365));
#40604=CARTESIAN_POINT('',(-4.18409499139877,51.145,-3.34686616149372));
#40605=CARTESIAN_POINT('',(-4.18409499139877,54.32,-3.34686616149372));
#40606=CARTESIAN_POINT('',(-4.06695907338649,51.145,-3.25316890053365));
#40607=CARTESIAN_POINT('Ctrl Pts',(-4.87380761862879,57.495,-5.22328778611671));
#40608=CARTESIAN_POINT('Ctrl Pts',(-4.87380761862879,49.875,-5.22328778611671));
#40609=CARTESIAN_POINT('Ctrl Pts',(-4.86276047837859,57.495,-5.2205826053545));
#40610=CARTESIAN_POINT('Ctrl Pts',(-4.86276047837859,49.875,-5.2205826053545));
#40611=CARTESIAN_POINT('Ctrl Pts',(-4.84075823631825,57.495,-5.21511826561704));
#40612=CARTESIAN_POINT('Ctrl Pts',(-4.84075823631825,49.875,-5.21511826561704));
#40613=CARTESIAN_POINT('Ctrl Pts',(-4.80803098811744,57.495,-5.20675982149348));
#40614=CARTESIAN_POINT('Ctrl Pts',(-4.80803098811744,49.875,-5.20675982149348));
#40615=CARTESIAN_POINT('Ctrl Pts',(-4.7649478905793,57.495,-5.19529077281773));
#40616=CARTESIAN_POINT('Ctrl Pts',(-4.7649478905793,49.875,-5.19529077281773));
#40617=CARTESIAN_POINT('Ctrl Pts',(-4.71202254995864,57.495,-5.18041062500752));
#40618=CARTESIAN_POINT('Ctrl Pts',(-4.71202254995864,49.875,-5.18041062500752));
#40619=CARTESIAN_POINT('Ctrl Pts',(-4.66003509375265,57.495,-5.16498334493456));
#40620=CARTESIAN_POINT('Ctrl Pts',(-4.66003509375265,49.875,-5.16498334493456));
#40621=CARTESIAN_POINT('Ctrl Pts',(-4.60899638270439,57.495,-5.14900691787064));
#40622=CARTESIAN_POINT('Ctrl Pts',(-4.60899638270439,49.875,-5.14900691787064));
#40623=CARTESIAN_POINT('Ctrl Pts',(-4.5589176169425,57.495,-5.13248213818666));
#40624=CARTESIAN_POINT('Ctrl Pts',(-4.5589176169425,49.875,-5.13248213818666));
#40625=CARTESIAN_POINT('Ctrl Pts',(-4.50980818622101,57.495,-5.11541439426204));
#40626=CARTESIAN_POINT('Ctrl Pts',(-4.50980818622101,49.875,-5.11541439426204));
#40627=CARTESIAN_POINT('Ctrl Pts',(-4.4616773428065,57.495,-5.09781475579217));
#40628=CARTESIAN_POINT('Ctrl Pts',(-4.4616773428065,49.875,-5.09781475579217));
#40629=CARTESIAN_POINT('Ctrl Pts',(-4.41453743405677,57.495,-5.07970066295468));
#40630=CARTESIAN_POINT('Ctrl Pts',(-4.41453743405677,49.875,-5.07970066295468));
#40631=CARTESIAN_POINT('Ctrl Pts',(-4.36840670797617,57.495,-5.06109712122989));
#40632=CARTESIAN_POINT('Ctrl Pts',(-4.36840670797617,49.875,-5.06109712122989));
#40633=CARTESIAN_POINT('Ctrl Pts',(-4.3233115657319,57.495,-5.04203735157413));
#40634=CARTESIAN_POINT('Ctrl Pts',(-4.3233115657319,49.875,-5.04203735157413));
#40635=CARTESIAN_POINT('Ctrl Pts',(-4.27929023600674,57.495,-5.02256507114894));
#40636=CARTESIAN_POINT('Ctrl Pts',(-4.27929023600674,49.875,-5.02256507114894));
#40637=CARTESIAN_POINT('Ctrl Pts',(-4.23639070615337,57.495,-5.00273172317863));
#40638=CARTESIAN_POINT('Ctrl Pts',(-4.23639070615337,49.875,-5.00273172317863));
#40639=CARTESIAN_POINT('Ctrl Pts',(-4.1946621629253,57.495,-4.98258807456961));
#40640=CARTESIAN_POINT('Ctrl Pts',(-4.1946621629253,49.875,-4.98258807456961));
#40641=CARTESIAN_POINT('Ctrl Pts',(-4.15414724283858,57.495,-4.96217669200723));
#40642=CARTESIAN_POINT('Ctrl Pts',(-4.15414724283858,49.875,-4.96217669200723));
#40643=CARTESIAN_POINT('Ctrl Pts',(-4.11487510765791,57.495,-4.94152548435402));
#40644=CARTESIAN_POINT('Ctrl Pts',(-4.11487510765791,49.875,-4.94152548435402));
#40645=CARTESIAN_POINT('Ctrl Pts',(-4.07685036350539,57.495,-4.92063739759521));
#40646=CARTESIAN_POINT('Ctrl Pts',(-4.07685036350539,49.875,-4.92063739759521));
#40647=CARTESIAN_POINT('Ctrl Pts',(-4.04005493051012,57.495,-4.89949292161185));
#40648=CARTESIAN_POINT('Ctrl Pts',(-4.04005493051012,49.875,-4.89949292161185));
#40649=CARTESIAN_POINT('Ctrl Pts',(-4.00447382552396,57.495,-4.87807598288654));
#40650=CARTESIAN_POINT('Ctrl Pts',(-4.00447382552396,49.875,-4.87807598288654));
#40651=CARTESIAN_POINT('Ctrl Pts',(-3.97011673859274,57.495,-4.85639607415676));
#40652=CARTESIAN_POINT('Ctrl Pts',(-3.97011673859274,49.875,-4.85639607415676));
#40653=CARTESIAN_POINT('Ctrl Pts',(-3.93703846717724,57.495,-4.83450929444279));
#40654=CARTESIAN_POINT('Ctrl Pts',(-3.93703846717724,49.875,-4.83450929444279));
#40655=CARTESIAN_POINT('Ctrl Pts',(-3.90536636162318,57.495,-4.81254694822034));
#40656=CARTESIAN_POINT('Ctrl Pts',(-3.90536636162318,49.875,-4.81254694822034));
#40657=CARTESIAN_POINT('Ctrl Pts',(-3.8753026227458,57.495,-4.79071829540103));
#40658=CARTESIAN_POINT('Ctrl Pts',(-3.8753026227458,49.875,-4.79071829540103));
#40659=CARTESIAN_POINT('Ctrl Pts',(-3.84708445224627,57.495,-4.76926976684252));
#40660=CARTESIAN_POINT('Ctrl Pts',(-3.84708445224627,49.875,-4.76926976684252));
#40661=CARTESIAN_POINT('Ctrl Pts',(-3.82095228990397,57.495,-4.74845295472312));
#40662=CARTESIAN_POINT('Ctrl Pts',(-3.82095228990397,49.875,-4.74845295472312));
#40663=CARTESIAN_POINT('Ctrl Pts',(-3.7971178338476,57.495,-4.72849227702427));
#40664=CARTESIAN_POINT('Ctrl Pts',(-3.7971178338476,49.875,-4.72849227702427));
#40665=CARTESIAN_POINT('Ctrl Pts',(-3.77572337177431,57.495,-4.7095447400518));
#40666=CARTESIAN_POINT('Ctrl Pts',(-3.77572337177431,49.875,-4.7095447400518));
#40667=CARTESIAN_POINT('Ctrl Pts',(-3.75683893603616,57.495,-4.69169578253132));
#40668=CARTESIAN_POINT('Ctrl Pts',(-3.75683893603616,49.875,-4.69169578253132));
#40669=CARTESIAN_POINT('Ctrl Pts',(-3.74375974890886,57.495,-4.67832660775287));
#40670=CARTESIAN_POINT('Ctrl Pts',(-3.74375974890886,49.875,-4.67832660775287));
#40671=CARTESIAN_POINT('Ctrl Pts',(-3.73509073349858,57.495,-4.66881533805013));
#40672=CARTESIAN_POINT('Ctrl Pts',(-3.73509073349858,49.875,-4.66881533805013));
#40673=CARTESIAN_POINT('Ctrl Pts',(-3.72981733050578,57.495,-4.66270326064959));
#40674=CARTESIAN_POINT('Ctrl Pts',(-3.72981733050578,49.875,-4.66270326064959));
#40675=CARTESIAN_POINT('Ctrl Pts',(-3.72730711280926,57.495,-4.65970441290367));
#40676=CARTESIAN_POINT('Ctrl Pts',(-3.72730711280926,49.875,-4.65970441290367));
#40677=CARTESIAN_POINT('Ctrl Pts',(-4.87380761862879,51.145,-5.22328778611671));
#40678=CARTESIAN_POINT('Ctrl Pts',(-4.86276047837859,51.145,-5.2205826053545));
#40679=CARTESIAN_POINT('Ctrl Pts',(-4.84075823631825,51.145,-5.21511826561704));
#40680=CARTESIAN_POINT('Ctrl Pts',(-4.80803098811744,51.145,-5.20675982149348));
#40681=CARTESIAN_POINT('Ctrl Pts',(-4.7649478905793,51.145,-5.19529077281773));
#40682=CARTESIAN_POINT('Ctrl Pts',(-4.71202254995864,51.145,-5.18041062500752));
#40683=CARTESIAN_POINT('Ctrl Pts',(-4.66003509375265,51.145,-5.16498334493456));
#40684=CARTESIAN_POINT('Ctrl Pts',(-4.60899638270439,51.145,-5.14900691787064));
#40685=CARTESIAN_POINT('Ctrl Pts',(-4.5589176169425,51.145,-5.13248213818666));
#40686=CARTESIAN_POINT('Ctrl Pts',(-4.50980818622101,51.145,-5.11541439426204));
#40687=CARTESIAN_POINT('Ctrl Pts',(-4.4616773428065,51.145,-5.09781475579217));
#40688=CARTESIAN_POINT('Ctrl Pts',(-4.41453743405677,51.145,-5.07970066295468));
#40689=CARTESIAN_POINT('Ctrl Pts',(-4.36840670797617,51.145,-5.06109712122989));
#40690=CARTESIAN_POINT('Ctrl Pts',(-4.3233115657319,51.145,-5.04203735157413));
#40691=CARTESIAN_POINT('Ctrl Pts',(-4.27929023600674,51.145,-5.02256507114894));
#40692=CARTESIAN_POINT('Ctrl Pts',(-4.23639070615337,51.145,-5.00273172317863));
#40693=CARTESIAN_POINT('Ctrl Pts',(-4.1946621629253,51.145,-4.98258807456961));
#40694=CARTESIAN_POINT('Ctrl Pts',(-4.15414724283858,51.145,-4.96217669200723));
#40695=CARTESIAN_POINT('Ctrl Pts',(-4.11487510765791,51.145,-4.94152548435402));
#40696=CARTESIAN_POINT('Ctrl Pts',(-4.07685036350539,51.145,-4.92063739759521));
#40697=CARTESIAN_POINT('Ctrl Pts',(-4.04005493051012,51.145,-4.89949292161185));
#40698=CARTESIAN_POINT('Ctrl Pts',(-4.00447382552396,51.145,-4.87807598288654));
#40699=CARTESIAN_POINT('Ctrl Pts',(-3.97011673859274,51.145,-4.85639607415676));
#40700=CARTESIAN_POINT('Ctrl Pts',(-3.93703846717724,51.145,-4.83450929444279));
#40701=CARTESIAN_POINT('Ctrl Pts',(-3.90536636162318,51.145,-4.81254694822034));
#40702=CARTESIAN_POINT('Ctrl Pts',(-3.8753026227458,51.145,-4.79071829540103));
#40703=CARTESIAN_POINT('Ctrl Pts',(-3.84708445224627,51.145,-4.76926976684252));
#40704=CARTESIAN_POINT('Ctrl Pts',(-3.82095228990397,51.145,-4.74845295472312));
#40705=CARTESIAN_POINT('Ctrl Pts',(-3.7971178338476,51.145,-4.72849227702427));
#40706=CARTESIAN_POINT('Ctrl Pts',(-3.77572337177431,51.145,-4.7095447400518));
#40707=CARTESIAN_POINT('Ctrl Pts',(-3.75683893603616,51.145,-4.69169578253132));
#40708=CARTESIAN_POINT('Ctrl Pts',(-3.74375974890886,51.145,-4.67832660775287));
#40709=CARTESIAN_POINT('Ctrl Pts',(-3.73509073349858,51.145,-4.66881533805013));
#40710=CARTESIAN_POINT('Ctrl Pts',(-3.72981733050578,51.145,-4.66270326064959));
#40711=CARTESIAN_POINT('Ctrl Pts',(-3.72730711280926,51.145,-4.65970441290367));
#40712=CARTESIAN_POINT('Origin',(0.,54.32,0.));
#40713=CARTESIAN_POINT('',(-4.69328497730872,51.145,-2.58480949428933));
#40714=CARTESIAN_POINT('Origin',(0.,51.145,0.));
#40715=CARTESIAN_POINT('',(-4.69328497730872,54.32,-2.58480949428933));
#40716=CARTESIAN_POINT('Origin',(-5.22677443144495,57.495,-2.87862685522556));
#40717=CARTESIAN_POINT('',(-5.22677443144495,51.145,-2.87862685522556));
#40718=CARTESIAN_POINT('',(-5.22677443144495,51.145,-2.87862685522556));
#40719=CARTESIAN_POINT('',(-5.22677443144495,57.495,-2.87862685522556));
#40720=CARTESIAN_POINT('Origin',(-1.50487931058895E-12,57.495,-6.22890783902202E-13));
#40721=CARTESIAN_POINT('',(-6.50167680247051,51.145,-2.96056324982543));
#40722=CARTESIAN_POINT('',(-6.50167680247051,57.495,-2.96056324982543));
#40723=CARTESIAN_POINT('',(-6.69081410619341,51.145,-2.50394540602692));
#40724=CARTESIAN_POINT('Origin',(-1.50487931058895E-12,51.145,-6.22890783902202E-13));
#40725=CARTESIAN_POINT('',(-6.69081410619341,57.495,-2.50394540602692));
#40726=CARTESIAN_POINT('Ctrl Pts',(-5.73138421404289,57.495,-1.66039107437148));
#40727=CARTESIAN_POINT('Ctrl Pts',(-5.73138421404289,49.875,-1.66039107437148));
#40728=CARTESIAN_POINT('Ctrl Pts',(-5.73511540682056,57.495,-1.66156260377487));
#40729=CARTESIAN_POINT('Ctrl Pts',(-5.73511540682056,49.875,-1.66156260377487));
#40730=CARTESIAN_POINT('Ctrl Pts',(-5.7427802739896,57.495,-1.66409560210805));
#40731=CARTESIAN_POINT('Ctrl Pts',(-5.7427802739896,49.875,-1.66409560210805));
#40732=CARTESIAN_POINT('Ctrl Pts',(-5.75488502996861,57.495,-1.6684649226766));
#40733=CARTESIAN_POINT('Ctrl Pts',(-5.75488502996861,49.875,-1.6684649226766));
#40734=CARTESIAN_POINT('Ctrl Pts',(-5.77224172513541,57.495,-1.67543235427329));
#40735=CARTESIAN_POINT('Ctrl Pts',(-5.77224172513541,49.875,-1.67543235427329));
#40736=CARTESIAN_POINT('Ctrl Pts',(-5.79595877235177,57.495,-1.68604879760674));
#40737=CARTESIAN_POINT('Ctrl Pts',(-5.79595877235177,49.875,-1.68604879760674));
#40738=CARTESIAN_POINT('Ctrl Pts',(-5.82165132013192,57.495,-1.69856379474191));
#40739=CARTESIAN_POINT('Ctrl Pts',(-5.82165132013192,49.875,-1.69856379474191));
#40740=CARTESIAN_POINT('Ctrl Pts',(-5.84921363316513,57.495,-1.71294534020683));
#40741=CARTESIAN_POINT('Ctrl Pts',(-5.84921363316513,49.875,-1.71294534020683));
#40742=CARTESIAN_POINT('Ctrl Pts',(-5.87844620539462,57.495,-1.7291220610224));
#40743=CARTESIAN_POINT('Ctrl Pts',(-5.87844620539462,49.875,-1.7291220610224));
#40744=CARTESIAN_POINT('Ctrl Pts',(-5.90906068827411,57.495,-1.74698425466387));
#40745=CARTESIAN_POINT('Ctrl Pts',(-5.90906068827411,49.875,-1.74698425466387));
#40746=CARTESIAN_POINT('Ctrl Pts',(-5.94073262861949,57.495,-1.76640606389864));
#40747=CARTESIAN_POINT('Ctrl Pts',(-5.94073262861949,49.875,-1.76640606389864));
#40748=CARTESIAN_POINT('Ctrl Pts',(-5.97314358084403,57.495,-1.78726264793636));
#40749=CARTESIAN_POINT('Ctrl Pts',(-5.97314358084403,49.875,-1.78726264793636));
#40750=CARTESIAN_POINT('Ctrl Pts',(-6.00602283509639,57.495,-1.80944727788364));
#40751=CARTESIAN_POINT('Ctrl Pts',(-6.00602283509639,49.875,-1.80944727788364));
#40752=CARTESIAN_POINT('Ctrl Pts',(-6.03920034699149,57.495,-1.83289254541003));
#40753=CARTESIAN_POINT('Ctrl Pts',(-6.03920034699149,49.875,-1.83289254541003));
#40754=CARTESIAN_POINT('Ctrl Pts',(-6.07260331771232,57.495,-1.85756929242873));
#40755=CARTESIAN_POINT('Ctrl Pts',(-6.07260331771232,49.875,-1.85756929242873));
#40756=CARTESIAN_POINT('Ctrl Pts',(-6.10621926889299,57.495,-1.88347219921808));
#40757=CARTESIAN_POINT('Ctrl Pts',(-6.10621926889299,49.875,-1.88347219921808));
#40758=CARTESIAN_POINT('Ctrl Pts',(-6.14006878432982,57.495,-1.91060895733317));
#40759=CARTESIAN_POINT('Ctrl Pts',(-6.14006878432982,49.875,-1.91060895733317));
#40760=CARTESIAN_POINT('Ctrl Pts',(-6.17417680788945,57.495,-1.93898880419737));
#40761=CARTESIAN_POINT('Ctrl Pts',(-6.17417680788945,49.875,-1.93898880419737));
#40762=CARTESIAN_POINT('Ctrl Pts',(-6.20853885514981,57.495,-1.96860861168851));
#40763=CARTESIAN_POINT('Ctrl Pts',(-6.20853885514981,49.875,-1.96860861168851));
#40764=CARTESIAN_POINT('Ctrl Pts',(-6.24311798195985,57.495,-1.99945211810837));
#40765=CARTESIAN_POINT('Ctrl Pts',(-6.24311798195985,49.875,-1.99945211810837));
#40766=CARTESIAN_POINT('Ctrl Pts',(-6.27785854554194,57.495,-2.03149622201768));
#40767=CARTESIAN_POINT('Ctrl Pts',(-6.27785854554194,49.875,-2.03149622201768));
#40768=CARTESIAN_POINT('Ctrl Pts',(-6.31269482043467,57.495,-2.06471490843563));
#40769=CARTESIAN_POINT('Ctrl Pts',(-6.31269482043467,49.875,-2.06471490843563));
#40770=CARTESIAN_POINT('Ctrl Pts',(-6.34756091533115,57.495,-2.09908352929888));
#40771=CARTESIAN_POINT('Ctrl Pts',(-6.34756091533115,49.875,-2.09908352929888));
#40772=CARTESIAN_POINT('Ctrl Pts',(-6.38240181135703,57.495,-2.13458349574329));
#40773=CARTESIAN_POINT('Ctrl Pts',(-6.38240181135703,49.875,-2.13458349574329));
#40774=CARTESIAN_POINT('Ctrl Pts',(-6.41717671306138,57.495,-2.17120312938042));
#40775=CARTESIAN_POINT('Ctrl Pts',(-6.41717671306138,49.875,-2.17120312938042));
#40776=CARTESIAN_POINT('Ctrl Pts',(-6.45185553518375,57.495,-2.20893514043555));
#40777=CARTESIAN_POINT('Ctrl Pts',(-6.45185553518375,49.875,-2.20893514043555));
#40778=CARTESIAN_POINT('Ctrl Pts',(-6.48641743997175,57.495,-2.24777479550457));
#40779=CARTESIAN_POINT('Ctrl Pts',(-6.48641743997175,49.875,-2.24777479550457));
#40780=CARTESIAN_POINT('Ctrl Pts',(-6.52084865967127,57.495,-2.2877177827968));
#40781=CARTESIAN_POINT('Ctrl Pts',(-6.52084865967127,49.875,-2.2877177827968));
#40782=CARTESIAN_POINT('Ctrl Pts',(-6.55514062276556,57.495,-2.32875748935421));
#40783=CARTESIAN_POINT('Ctrl Pts',(-6.55514062276556,49.875,-2.32875748935421));
#40784=CARTESIAN_POINT('Ctrl Pts',(-6.58928830924802,57.495,-2.37088387159981));
#40785=CARTESIAN_POINT('Ctrl Pts',(-6.58928830924802,49.875,-2.37088387159981));
#40786=CARTESIAN_POINT('Ctrl Pts',(-6.6232894242584,57.495,-2.41408612451229));
#40787=CARTESIAN_POINT('Ctrl Pts',(-6.6232894242584,49.875,-2.41408612451229));
#40788=CARTESIAN_POINT('Ctrl Pts',(-6.65037263123018,57.495,-2.4495007016118));
#40789=CARTESIAN_POINT('Ctrl Pts',(-6.65037263123018,49.875,-2.4495007016118));
#40790=CARTESIAN_POINT('Ctrl Pts',(-6.67061900235304,57.495,-2.47653809829358));
#40791=CARTESIAN_POINT('Ctrl Pts',(-6.67061900235304,49.875,-2.47653809829358));
#40792=CARTESIAN_POINT('Ctrl Pts',(-6.68408728750664,57.495,-2.49477440711619));
#40793=CARTESIAN_POINT('Ctrl Pts',(-6.68408728750664,49.875,-2.49477440711619));
#40794=CARTESIAN_POINT('Ctrl Pts',(-6.69081410619341,57.495,-2.50394540602692));
#40795=CARTESIAN_POINT('Ctrl Pts',(-6.69081410619341,49.875,-2.50394540602692));
#40796=CARTESIAN_POINT('',(-5.73138421404289,51.145,-1.66039107437148));
#40797=CARTESIAN_POINT('Ctrl Pts',(-5.73138421404289,51.145,-1.66039107437148));
#40798=CARTESIAN_POINT('Ctrl Pts',(-5.73511540682056,51.145,-1.66156260377487));
#40799=CARTESIAN_POINT('Ctrl Pts',(-5.7427802739896,51.145,-1.66409560210805));
#40800=CARTESIAN_POINT('Ctrl Pts',(-5.75488502996861,51.145,-1.6684649226766));
#40801=CARTESIAN_POINT('Ctrl Pts',(-5.77224172513541,51.145,-1.67543235427329));
#40802=CARTESIAN_POINT('Ctrl Pts',(-5.79595877235177,51.145,-1.68604879760674));
#40803=CARTESIAN_POINT('Ctrl Pts',(-5.82165132013192,51.145,-1.69856379474191));
#40804=CARTESIAN_POINT('Ctrl Pts',(-5.84921363316513,51.145,-1.71294534020683));
#40805=CARTESIAN_POINT('Ctrl Pts',(-5.87844620539462,51.145,-1.7291220610224));
#40806=CARTESIAN_POINT('Ctrl Pts',(-5.90906068827411,51.145,-1.74698425466387));
#40807=CARTESIAN_POINT('Ctrl Pts',(-5.94073262861949,51.145,-1.76640606389864));
#40808=CARTESIAN_POINT('Ctrl Pts',(-5.97314358084403,51.145,-1.78726264793636));
#40809=CARTESIAN_POINT('Ctrl Pts',(-6.00602283509639,51.145,-1.80944727788364));
#40810=CARTESIAN_POINT('Ctrl Pts',(-6.03920034699149,51.145,-1.83289254541003));
#40811=CARTESIAN_POINT('Ctrl Pts',(-6.07260331771232,51.145,-1.85756929242873));
#40812=CARTESIAN_POINT('Ctrl Pts',(-6.10621926889299,51.145,-1.88347219921808));
#40813=CARTESIAN_POINT('Ctrl Pts',(-6.14006878432982,51.145,-1.91060895733317));
#40814=CARTESIAN_POINT('Ctrl Pts',(-6.17417680788945,51.145,-1.93898880419737));
#40815=CARTESIAN_POINT('Ctrl Pts',(-6.20853885514981,51.145,-1.96860861168851));
#40816=CARTESIAN_POINT('Ctrl Pts',(-6.24311798195985,51.145,-1.99945211810837));
#40817=CARTESIAN_POINT('Ctrl Pts',(-6.27785854554194,51.145,-2.03149622201768));
#40818=CARTESIAN_POINT('Ctrl Pts',(-6.31269482043467,51.145,-2.06471490843563));
#40819=CARTESIAN_POINT('Ctrl Pts',(-6.34756091533115,51.145,-2.09908352929888));
#40820=CARTESIAN_POINT('Ctrl Pts',(-6.38240181135703,51.145,-2.13458349574329));
#40821=CARTESIAN_POINT('Ctrl Pts',(-6.41717671306138,51.145,-2.17120312938042));
#40822=CARTESIAN_POINT('Ctrl Pts',(-6.45185553518375,51.145,-2.20893514043555));
#40823=CARTESIAN_POINT('Ctrl Pts',(-6.48641743997175,51.145,-2.24777479550457));
#40824=CARTESIAN_POINT('Ctrl Pts',(-6.52084865967127,51.145,-2.2877177827968));
#40825=CARTESIAN_POINT('Ctrl Pts',(-6.55514062276556,51.145,-2.32875748935421));
#40826=CARTESIAN_POINT('Ctrl Pts',(-6.58928830924802,51.145,-2.37088387159981));
#40827=CARTESIAN_POINT('Ctrl Pts',(-6.6232894242584,51.145,-2.41408612451229));
#40828=CARTESIAN_POINT('Ctrl Pts',(-6.65037263123018,51.145,-2.4495007016118));
#40829=CARTESIAN_POINT('Ctrl Pts',(-6.67061900235304,51.145,-2.47653809829358));
#40830=CARTESIAN_POINT('Ctrl Pts',(-6.68408728750664,51.145,-2.49477440711619));
#40831=CARTESIAN_POINT('Ctrl Pts',(-6.69081410619341,51.145,-2.50394540602692));
#40832=CARTESIAN_POINT('',(-5.73138421404289,57.495,-1.66039107437148));
#40833=CARTESIAN_POINT('Origin',(-5.00231408838243,57.495,-1.44917830551339));
#40834=CARTESIAN_POINT('',(-5.1463899549833,51.145,-1.4909173120086));
#40835=CARTESIAN_POINT('',(-5.1463899549833,54.32,-1.4909173120086));
#40836=CARTESIAN_POINT('',(-5.00231408838243,51.145,-1.44917830551339));
#40837=CARTESIAN_POINT('Ctrl Pts',(-6.50167680247051,57.495,-2.96056324982543));
#40838=CARTESIAN_POINT('Ctrl Pts',(-6.50167680247051,49.875,-2.96056324982543));
#40839=CARTESIAN_POINT('Ctrl Pts',(-6.49043534784131,57.495,-2.96229154623625));
#40840=CARTESIAN_POINT('Ctrl Pts',(-6.49043534784131,49.875,-2.96229154623625));
#40841=CARTESIAN_POINT('Ctrl Pts',(-6.46801681444607,57.495,-2.96566304810549));
#40842=CARTESIAN_POINT('Ctrl Pts',(-6.46801681444607,49.875,-2.96566304810549));
#40843=CARTESIAN_POINT('Ctrl Pts',(-6.43458214159149,57.495,-2.97046502832945));
#40844=CARTESIAN_POINT('Ctrl Pts',(-6.43458214159149,49.875,-2.97046502832945));
#40845=CARTESIAN_POINT('Ctrl Pts',(-6.39038953466561,57.495,-2.97635619664337));
#40846=CARTESIAN_POINT('Ctrl Pts',(-6.39038953466561,49.875,-2.97635619664337));
#40847=CARTESIAN_POINT('Ctrl Pts',(-6.33579850967689,57.495,-2.98286238364857));
#40848=CARTESIAN_POINT('Ctrl Pts',(-6.33579850967689,49.875,-2.98286238364857));
#40849=CARTESIAN_POINT('Ctrl Pts',(-6.28186459845047,57.495,-2.98850417352769));
#40850=CARTESIAN_POINT('Ctrl Pts',(-6.28186459845047,49.875,-2.98850417352769));
#40851=CARTESIAN_POINT('Ctrl Pts',(-6.22859706400147,57.495,-2.99327554868811));
#40852=CARTESIAN_POINT('Ctrl Pts',(-6.22859706400147,49.875,-2.99327554868811));
#40853=CARTESIAN_POINT('Ctrl Pts',(-6.17600655789209,57.495,-2.99717295692919));
#40854=CARTESIAN_POINT('Ctrl Pts',(-6.17600655789209,49.875,-2.99717295692919));
#40855=CARTESIAN_POINT('Ctrl Pts',(-6.12410381716742,57.495,-3.00019778316108));
#40856=CARTESIAN_POINT('Ctrl Pts',(-6.12410381716742,49.875,-3.00019778316108));
#40857=CARTESIAN_POINT('Ctrl Pts',(-6.07290162599622,57.495,-3.00235671375967));
#40858=CARTESIAN_POINT('Ctrl Pts',(-6.07290162599622,49.875,-3.00235671375967));
#40859=CARTESIAN_POINT('Ctrl Pts',(-6.02241806591666,57.495,-3.00366113621883));
#40860=CARTESIAN_POINT('Ctrl Pts',(-6.02241806591666,49.875,-3.00366113621883));
#40861=CARTESIAN_POINT('Ctrl Pts',(-5.97267956506952,57.495,-3.00412716938109));
#40862=CARTESIAN_POINT('Ctrl Pts',(-5.97267956506952,49.875,-3.00412716938109));
#40863=CARTESIAN_POINT('Ctrl Pts',(-5.9237232280624,57.495,-3.00377540211877));
#40864=CARTESIAN_POINT('Ctrl Pts',(-5.9237232280624,49.875,-3.00377540211877));
#40865=CARTESIAN_POINT('Ctrl Pts',(-5.87560110342631,57.495,-3.00263159433912));
#40866=CARTESIAN_POINT('Ctrl Pts',(-5.87560110342631,49.875,-3.00263159433912));
#40867=CARTESIAN_POINT('Ctrl Pts',(-5.82837721216385,57.495,-3.00072490941932));
#40868=CARTESIAN_POINT('Ctrl Pts',(-5.82837721216385,49.875,-3.00072490941932));
#40869=CARTESIAN_POINT('Ctrl Pts',(-5.78211642456387,57.495,-2.99808342690946));
#40870=CARTESIAN_POINT('Ctrl Pts',(-5.78211642456387,49.875,-2.99808342690946));
#40871=CARTESIAN_POINT('Ctrl Pts',(-5.73687442119613,57.495,-2.9947301570106));
#40872=CARTESIAN_POINT('Ctrl Pts',(-5.73687442119613,49.875,-2.9947301570106));
#40873=CARTESIAN_POINT('Ctrl Pts',(-5.69268882427748,57.495,-2.9906797244254));
#40874=CARTESIAN_POINT('Ctrl Pts',(-5.69268882427748,49.875,-2.9906797244254));
#40875=CARTESIAN_POINT('Ctrl Pts',(-5.64956501668959,57.495,-2.98593308820271));
#40876=CARTESIAN_POINT('Ctrl Pts',(-5.64956501668959,49.875,-2.98593308820271));
#40877=CARTESIAN_POINT('Ctrl Pts',(-5.6074788286105,57.495,-2.98047914221));
#40878=CARTESIAN_POINT('Ctrl Pts',(-5.6074788286105,49.875,-2.98047914221));
#40879=CARTESIAN_POINT('Ctrl Pts',(-5.56641026634749,57.495,-2.97430877025609));
#40880=CARTESIAN_POINT('Ctrl Pts',(-5.56641026634749,49.875,-2.97430877025609));
#40881=CARTESIAN_POINT('Ctrl Pts',(-5.52637191504895,57.495,-2.96742703426683));
#40882=CARTESIAN_POINT('Ctrl Pts',(-5.52637191504895,49.875,-2.96742703426683));
#40883=CARTESIAN_POINT('Ctrl Pts',(-5.48743586913296,57.495,-2.9598647928985));
#40884=CARTESIAN_POINT('Ctrl Pts',(-5.48743586913296,49.875,-2.9598647928985));
#40885=CARTESIAN_POINT('Ctrl Pts',(-5.44977003302482,57.495,-2.95169462080131));
#40886=CARTESIAN_POINT('Ctrl Pts',(-5.44977003302482,49.875,-2.95169462080131));
#40887=CARTESIAN_POINT('Ctrl Pts',(-5.41364129622045,57.495,-2.94303247002258));
#40888=CARTESIAN_POINT('Ctrl Pts',(-5.41364129622045,49.875,-2.94303247002258));
#40889=CARTESIAN_POINT('Ctrl Pts',(-5.37936310952307,57.495,-2.93401523982671));
#40890=CARTESIAN_POINT('Ctrl Pts',(-5.37936310952307,49.875,-2.93401523982671));
#40891=CARTESIAN_POINT('Ctrl Pts',(-5.34725389048201,57.495,-2.92478335875774));
#40892=CARTESIAN_POINT('Ctrl Pts',(-5.34725389048201,49.875,-2.92478335875774));
#40893=CARTESIAN_POINT('Ctrl Pts',(-5.31759510370885,57.495,-2.91546314862891));
#40894=CARTESIAN_POINT('Ctrl Pts',(-5.31759510370885,49.875,-2.91546314862891));
#40895=CARTESIAN_POINT('Ctrl Pts',(-5.29057828960676,57.495,-2.90614521320837));
#40896=CARTESIAN_POINT('Ctrl Pts',(-5.29057828960676,49.875,-2.90614521320837));
#40897=CARTESIAN_POINT('Ctrl Pts',(-5.26630084561719,57.495,-2.89688168736508));
#40898=CARTESIAN_POINT('Ctrl Pts',(-5.26630084561719,49.875,-2.89688168736508));
#40899=CARTESIAN_POINT('Ctrl Pts',(-5.24910109063628,57.495,-2.88953536864313));
#40900=CARTESIAN_POINT('Ctrl Pts',(-5.24910109063628,49.875,-2.88953536864313));
#40901=CARTESIAN_POINT('Ctrl Pts',(-5.23745215939571,57.495,-2.884065589809));
#40902=CARTESIAN_POINT('Ctrl Pts',(-5.23745215939571,49.875,-2.884065589809));
#40903=CARTESIAN_POINT('Ctrl Pts',(-5.23024117954545,57.495,-2.88043681055505));
#40904=CARTESIAN_POINT('Ctrl Pts',(-5.23024117954545,49.875,-2.88043681055505));
#40905=CARTESIAN_POINT('Ctrl Pts',(-5.22677443144495,57.495,-2.87862685522556));
#40906=CARTESIAN_POINT('Ctrl Pts',(-5.22677443144495,49.875,-2.87862685522556));
#40907=CARTESIAN_POINT('Ctrl Pts',(-6.50167680247051,51.145,-2.96056324982543));
#40908=CARTESIAN_POINT('Ctrl Pts',(-6.49043534784131,51.145,-2.96229154623625));
#40909=CARTESIAN_POINT('Ctrl Pts',(-6.46801681444607,51.145,-2.96566304810549));
#40910=CARTESIAN_POINT('Ctrl Pts',(-6.43458214159149,51.145,-2.97046502832945));
#40911=CARTESIAN_POINT('Ctrl Pts',(-6.39038953466561,51.145,-2.97635619664337));
#40912=CARTESIAN_POINT('Ctrl Pts',(-6.33579850967689,51.145,-2.98286238364857));
#40913=CARTESIAN_POINT('Ctrl Pts',(-6.28186459845047,51.145,-2.98850417352769));
#40914=CARTESIAN_POINT('Ctrl Pts',(-6.22859706400147,51.145,-2.99327554868811));
#40915=CARTESIAN_POINT('Ctrl Pts',(-6.17600655789209,51.145,-2.99717295692919));
#40916=CARTESIAN_POINT('Ctrl Pts',(-6.12410381716742,51.145,-3.00019778316108));
#40917=CARTESIAN_POINT('Ctrl Pts',(-6.07290162599622,51.145,-3.00235671375967));
#40918=CARTESIAN_POINT('Ctrl Pts',(-6.02241806591666,51.145,-3.00366113621883));
#40919=CARTESIAN_POINT('Ctrl Pts',(-5.97267956506952,51.145,-3.00412716938109));
#40920=CARTESIAN_POINT('Ctrl Pts',(-5.9237232280624,51.145,-3.00377540211877));
#40921=CARTESIAN_POINT('Ctrl Pts',(-5.87560110342631,51.145,-3.00263159433912));
#40922=CARTESIAN_POINT('Ctrl Pts',(-5.82837721216385,51.145,-3.00072490941932));
#40923=CARTESIAN_POINT('Ctrl Pts',(-5.78211642456387,51.145,-2.99808342690946));
#40924=CARTESIAN_POINT('Ctrl Pts',(-5.73687442119613,51.145,-2.9947301570106));
#40925=CARTESIAN_POINT('Ctrl Pts',(-5.69268882427748,51.145,-2.9906797244254));
#40926=CARTESIAN_POINT('Ctrl Pts',(-5.64956501668959,51.145,-2.98593308820271));
#40927=CARTESIAN_POINT('Ctrl Pts',(-5.6074788286105,51.145,-2.98047914221));
#40928=CARTESIAN_POINT('Ctrl Pts',(-5.56641026634749,51.145,-2.97430877025609));
#40929=CARTESIAN_POINT('Ctrl Pts',(-5.52637191504895,51.145,-2.96742703426683));
#40930=CARTESIAN_POINT('Ctrl Pts',(-5.48743586913296,51.145,-2.9598647928985));
#40931=CARTESIAN_POINT('Ctrl Pts',(-5.44977003302482,51.145,-2.95169462080131));
#40932=CARTESIAN_POINT('Ctrl Pts',(-5.41364129622045,51.145,-2.94303247002258));
#40933=CARTESIAN_POINT('Ctrl Pts',(-5.37936310952307,51.145,-2.93401523982671));
#40934=CARTESIAN_POINT('Ctrl Pts',(-5.34725389048201,51.145,-2.92478335875774));
#40935=CARTESIAN_POINT('Ctrl Pts',(-5.31759510370885,51.145,-2.91546314862891));
#40936=CARTESIAN_POINT('Ctrl Pts',(-5.29057828960676,51.145,-2.90614521320837));
#40937=CARTESIAN_POINT('Ctrl Pts',(-5.26630084561719,51.145,-2.89688168736508));
#40938=CARTESIAN_POINT('Ctrl Pts',(-5.24910109063628,51.145,-2.88953536864313));
#40939=CARTESIAN_POINT('Ctrl Pts',(-5.23745215939571,51.145,-2.884065589809));
#40940=CARTESIAN_POINT('Ctrl Pts',(-5.23024117954545,51.145,-2.88043681055505));
#40941=CARTESIAN_POINT('Ctrl Pts',(-5.22677443144495,51.145,-2.87862685522556));
#40942=CARTESIAN_POINT('Origin',(0.,54.32,0.));
#40943=CARTESIAN_POINT('',(-5.32519370006274,51.145,-0.592010183030743));
#40944=CARTESIAN_POINT('Origin',(0.,51.145,0.));
#40945=CARTESIAN_POINT('',(-5.32519370006274,54.32,-0.592010183030743));
#40946=CARTESIAN_POINT('Origin',(-5.93051272372135,57.495,-0.659304453656786));
#40947=CARTESIAN_POINT('',(-5.93051272372135,51.145,-0.659304453656786));
#40948=CARTESIAN_POINT('',(-5.93051272372135,51.145,-0.659304453656786));
#40949=CARTESIAN_POINT('',(-5.93051272372135,57.495,-0.659304453656786));
#40950=CARTESIAN_POINT('Origin',(-1.6286971771251E-12,57.495,4.16333634234533E-16));
#40951=CARTESIAN_POINT('',(-7.13972463098307,51.145,-0.247119796320916));
#40952=CARTESIAN_POINT('',(-7.13972463098307,57.495,-0.247119796320916));
#40953=CARTESIAN_POINT('',(-7.13972463098307,51.145,0.24711979632092));
#40954=CARTESIAN_POINT('Origin',(-1.6286971771251E-12,51.145,4.16333634234533E-16));
#40955=CARTESIAN_POINT('',(-7.13972463098307,57.495,0.24711979632092));
#40956=CARTESIAN_POINT('Ctrl Pts',(-5.93051272372135,57.495,0.659304453656788));
#40957=CARTESIAN_POINT('Ctrl Pts',(-5.93051272372135,49.875,0.659304453656788));
#40958=CARTESIAN_POINT('Ctrl Pts',(-5.9344082212537,57.495,0.659649967278237));
#40959=CARTESIAN_POINT('Ctrl Pts',(-5.9344082212537,49.875,0.659649967278237));
#40960=CARTESIAN_POINT('Ctrl Pts',(-5.94245897164691,57.495,0.660242999639201));
#40961=CARTESIAN_POINT('Ctrl Pts',(-5.94245897164691,49.875,0.660242999639201));
#40962=CARTESIAN_POINT('Ctrl Pts',(-5.95531437453424,57.495,0.660838563360922));
#40963=CARTESIAN_POINT('Ctrl Pts',(-5.95531437453424,49.875,0.660838563360922));
#40964=CARTESIAN_POINT('Ctrl Pts',(-5.97401619058907,57.495,0.661043615595512));
#40965=CARTESIAN_POINT('Ctrl Pts',(-5.97401619058907,49.875,0.661043615595512));
#40966=CARTESIAN_POINT('Ctrl Pts',(-5.99999062205823,57.495,0.660311421925997));
#40967=CARTESIAN_POINT('Ctrl Pts',(-5.99999062205823,49.875,0.660311421925997));
#40968=CARTESIAN_POINT('Ctrl Pts',(-6.0285167231501,57.495,0.658581184594089));
#40969=CARTESIAN_POINT('Ctrl Pts',(-6.0285167231501,49.875,0.658581184594089));
#40970=CARTESIAN_POINT('Ctrl Pts',(-6.05948455921138,57.495,0.655842009648634));
#40971=CARTESIAN_POINT('Ctrl Pts',(-6.05948455921138,49.875,0.655842009648634));
#40972=CARTESIAN_POINT('Ctrl Pts',(-6.09268249742298,57.495,0.65208348946162));
#40973=CARTESIAN_POINT('Ctrl Pts',(-6.09268249742298,49.875,0.65208348946162));
#40974=CARTESIAN_POINT('Ctrl Pts',(-6.12780215712604,57.495,0.64729662973892));
#40975=CARTESIAN_POINT('Ctrl Pts',(-6.12780215712604,49.875,0.64729662973892));
#40976=CARTESIAN_POINT('Ctrl Pts',(-6.16449561918676,57.495,0.641473544543615));
#40977=CARTESIAN_POINT('Ctrl Pts',(-6.16449561918676,49.875,0.641473544543615));
#40978=CARTESIAN_POINT('Ctrl Pts',(-6.20242090374318,57.495,0.634607707876565));
#40979=CARTESIAN_POINT('Ctrl Pts',(-6.20242090374318,49.875,0.634607707876565));
#40980=CARTESIAN_POINT('Ctrl Pts',(-6.24128706412515,57.495,0.626694128202842));
#40981=CARTESIAN_POINT('Ctrl Pts',(-6.24128706412515,49.875,0.626694128202842));
#40982=CARTESIAN_POINT('Ctrl Pts',(-6.2809112037544,57.495,0.617730009530307));
#40983=CARTESIAN_POINT('Ctrl Pts',(-6.2809112037544,49.875,0.617730009530307));
#40984=CARTESIAN_POINT('Ctrl Pts',(-6.32121490697716,57.495,0.607714431517402));
#40985=CARTESIAN_POINT('Ctrl Pts',(-6.32121490697716,49.875,0.607714431517402));
#40986=CARTESIAN_POINT('Ctrl Pts',(-6.36218460951727,57.495,0.596647533682211));
#40987=CARTESIAN_POINT('Ctrl Pts',(-6.36218460951727,49.875,0.596647533682211));
#40988=CARTESIAN_POINT('Ctrl Pts',(-6.40384227175352,57.495,0.584530087032238));
#40989=CARTESIAN_POINT('Ctrl Pts',(-6.40384227175352,49.875,0.584530087032238));
#40990=CARTESIAN_POINT('Ctrl Pts',(-6.44621447382266,57.495,0.57136310290558));
#40991=CARTESIAN_POINT('Ctrl Pts',(-6.44621447382266,49.875,0.57136310290558));
#40992=CARTESIAN_POINT('Ctrl Pts',(-6.4892958755784,57.495,0.557147755196277));
#40993=CARTESIAN_POINT('Ctrl Pts',(-6.4892958755784,49.875,0.557147755196277));
#40994=CARTESIAN_POINT('Ctrl Pts',(-6.53304612199323,57.495,0.54188492983995));
#40995=CARTESIAN_POINT('Ctrl Pts',(-6.53304612199323,49.875,0.54188492983995));
#40996=CARTESIAN_POINT('Ctrl Pts',(-6.57740496530571,57.495,0.525574676214356));
#40997=CARTESIAN_POINT('Ctrl Pts',(-6.57740496530571,49.875,0.525574676214356));
#40998=CARTESIAN_POINT('Ctrl Pts',(-6.62230172760513,57.495,0.508215876982669));
#40999=CARTESIAN_POINT('Ctrl Pts',(-6.62230172760513,49.875,0.508215876982669));
#41000=CARTESIAN_POINT('Ctrl Pts',(-6.66766610085618,57.495,0.489806088474623));
#41001=CARTESIAN_POINT('Ctrl Pts',(-6.66766610085618,49.875,0.489806088474623));
#41002=CARTESIAN_POINT('Ctrl Pts',(-6.71344014059664,57.495,0.470341429749656));
#41003=CARTESIAN_POINT('Ctrl Pts',(-6.71344014059664,49.875,0.470341429749656));
#41004=CARTESIAN_POINT('Ctrl Pts',(-6.75958168761858,57.495,0.449817078488629));
#41005=CARTESIAN_POINT('Ctrl Pts',(-6.75958168761858,49.875,0.449817078488629));
#41006=CARTESIAN_POINT('Ctrl Pts',(-6.80606015708966,57.495,0.428228256434473));
#41007=CARTESIAN_POINT('Ctrl Pts',(-6.80606015708966,49.875,0.428228256434473));
#41008=CARTESIAN_POINT('Ctrl Pts',(-6.85285448604159,57.495,0.405571362419756));
#41009=CARTESIAN_POINT('Ctrl Pts',(-6.85285448604159,49.875,0.405571362419756));
#41010=CARTESIAN_POINT('Ctrl Pts',(-6.89995030467727,57.495,0.381845111328235));
#41011=CARTESIAN_POINT('Ctrl Pts',(-6.89995030467727,49.875,0.381845111328235));
#41012=CARTESIAN_POINT('Ctrl Pts',(-6.94733716327837,57.495,0.357052332559036));
#41013=CARTESIAN_POINT('Ctrl Pts',(-6.94733716327837,49.875,0.357052332559036));
#41014=CARTESIAN_POINT('Ctrl Pts',(-6.99500658045299,57.495,0.331200384094009));
#41015=CARTESIAN_POINT('Ctrl Pts',(-6.99500658045299,49.875,0.331200384094009));
#41016=CARTESIAN_POINT('Ctrl Pts',(-7.0429523011241,57.495,0.304298370266205));
#41017=CARTESIAN_POINT('Ctrl Pts',(-7.0429523011241,49.875,0.304298370266205));
#41018=CARTESIAN_POINT('Ctrl Pts',(-7.0815264936403,57.495,0.28194386193484));
#41019=CARTESIAN_POINT('Ctrl Pts',(-7.0815264936403,49.875,0.28194386193484));
#41020=CARTESIAN_POINT('Ctrl Pts',(-7.11057846529273,57.495,0.264712515322387));
#41021=CARTESIAN_POINT('Ctrl Pts',(-7.11057846529273,49.875,0.264712515322387));
#41022=CARTESIAN_POINT('Ctrl Pts',(-7.13000027153808,57.495,0.253018452443276));
#41023=CARTESIAN_POINT('Ctrl Pts',(-7.13000027153808,49.875,0.253018452443276));
#41024=CARTESIAN_POINT('Ctrl Pts',(-7.13972463098307,57.495,0.247119796320917));
#41025=CARTESIAN_POINT('Ctrl Pts',(-7.13972463098307,49.875,0.247119796320917));
#41026=CARTESIAN_POINT('',(-5.93051272372135,51.145,0.659304453656788));
#41027=CARTESIAN_POINT('Ctrl Pts',(-5.93051272372135,51.145,0.659304453656788));
#41028=CARTESIAN_POINT('Ctrl Pts',(-5.9344082212537,51.145,0.659649967278237));
#41029=CARTESIAN_POINT('Ctrl Pts',(-5.94245897164691,51.145,0.660242999639201));
#41030=CARTESIAN_POINT('Ctrl Pts',(-5.95531437453424,51.145,0.660838563360922));
#41031=CARTESIAN_POINT('Ctrl Pts',(-5.97401619058907,51.145,0.661043615595512));
#41032=CARTESIAN_POINT('Ctrl Pts',(-5.99999062205823,51.145,0.660311421925997));
#41033=CARTESIAN_POINT('Ctrl Pts',(-6.0285167231501,51.145,0.658581184594089));
#41034=CARTESIAN_POINT('Ctrl Pts',(-6.05948455921138,51.145,0.655842009648634));
#41035=CARTESIAN_POINT('Ctrl Pts',(-6.09268249742298,51.145,0.65208348946162));
#41036=CARTESIAN_POINT('Ctrl Pts',(-6.12780215712604,51.145,0.64729662973892));
#41037=CARTESIAN_POINT('Ctrl Pts',(-6.16449561918676,51.145,0.641473544543615));
#41038=CARTESIAN_POINT('Ctrl Pts',(-6.20242090374318,51.145,0.634607707876565));
#41039=CARTESIAN_POINT('Ctrl Pts',(-6.24128706412515,51.145,0.626694128202842));
#41040=CARTESIAN_POINT('Ctrl Pts',(-6.2809112037544,51.145,0.617730009530307));
#41041=CARTESIAN_POINT('Ctrl Pts',(-6.32121490697716,51.145,0.607714431517402));
#41042=CARTESIAN_POINT('Ctrl Pts',(-6.36218460951727,51.145,0.596647533682211));
#41043=CARTESIAN_POINT('Ctrl Pts',(-6.40384227175352,51.145,0.584530087032238));
#41044=CARTESIAN_POINT('Ctrl Pts',(-6.44621447382266,51.145,0.57136310290558));
#41045=CARTESIAN_POINT('Ctrl Pts',(-6.4892958755784,51.145,0.557147755196277));
#41046=CARTESIAN_POINT('Ctrl Pts',(-6.53304612199323,51.145,0.54188492983995));
#41047=CARTESIAN_POINT('Ctrl Pts',(-6.57740496530571,51.145,0.525574676214356));
#41048=CARTESIAN_POINT('Ctrl Pts',(-6.62230172760513,51.145,0.508215876982669));
#41049=CARTESIAN_POINT('Ctrl Pts',(-6.66766610085618,51.145,0.489806088474623));
#41050=CARTESIAN_POINT('Ctrl Pts',(-6.71344014059664,51.145,0.470341429749656));
#41051=CARTESIAN_POINT('Ctrl Pts',(-6.75958168761858,51.145,0.449817078488629));
#41052=CARTESIAN_POINT('Ctrl Pts',(-6.80606015708966,51.145,0.428228256434473));
#41053=CARTESIAN_POINT('Ctrl Pts',(-6.85285448604159,51.145,0.405571362419756));
#41054=CARTESIAN_POINT('Ctrl Pts',(-6.89995030467727,51.145,0.381845111328235));
#41055=CARTESIAN_POINT('Ctrl Pts',(-6.94733716327837,51.145,0.357052332559036));
#41056=CARTESIAN_POINT('Ctrl Pts',(-6.99500658045299,51.145,0.331200384094009));
#41057=CARTESIAN_POINT('Ctrl Pts',(-7.0429523011241,51.145,0.304298370266205));
#41058=CARTESIAN_POINT('Ctrl Pts',(-7.0815264936403,51.145,0.28194386193484));
#41059=CARTESIAN_POINT('Ctrl Pts',(-7.11057846529273,51.145,0.264712515322387));
#41060=CARTESIAN_POINT('Ctrl Pts',(-7.13000027153808,51.145,0.253018452443276));
#41061=CARTESIAN_POINT('Ctrl Pts',(-7.13972463098307,51.145,0.247119796320917));
#41062=CARTESIAN_POINT('',(-5.93051272372135,57.495,0.659304453656788));
#41063=CARTESIAN_POINT('Origin',(-5.17611212951227,57.495,0.575436549687218));
#41064=CARTESIAN_POINT('',(-5.32519370006274,51.145,0.592010183030744));
#41065=CARTESIAN_POINT('',(-5.32519370006274,54.32,0.592010183030744));
#41066=CARTESIAN_POINT('',(-5.17611212951227,51.145,0.575436549687218));
#41067=CARTESIAN_POINT('Ctrl Pts',(-7.13972463098307,57.495,-0.247119796320916));
#41068=CARTESIAN_POINT('Ctrl Pts',(-7.13972463098307,49.875,-0.247119796320916));
#41069=CARTESIAN_POINT('Ctrl Pts',(-7.13000027153814,57.495,-0.253018452443266));
#41070=CARTESIAN_POINT('Ctrl Pts',(-7.13000027153814,49.875,-0.253018452443266));
#41071=CARTESIAN_POINT('Ctrl Pts',(-7.1105784652929,57.495,-0.264712515322364));
#41072=CARTESIAN_POINT('Ctrl Pts',(-7.1105784652929,49.875,-0.264712515322364));
#41073=CARTESIAN_POINT('Ctrl Pts',(-7.0815264936406,57.495,-0.281943861934803));
#41074=CARTESIAN_POINT('Ctrl Pts',(-7.0815264936406,49.875,-0.281943861934803));
#41075=CARTESIAN_POINT('Ctrl Pts',(-7.04295230112448,57.495,-0.304298370266162));
#41076=CARTESIAN_POINT('Ctrl Pts',(-7.04295230112448,49.875,-0.304298370266162));
#41077=CARTESIAN_POINT('Ctrl Pts',(-6.99500658045334,57.495,-0.331200384093975));
#41078=CARTESIAN_POINT('Ctrl Pts',(-6.99500658045334,49.875,-0.331200384093975));
#41079=CARTESIAN_POINT('Ctrl Pts',(-6.94733716327859,57.495,-0.357052332559016));
#41080=CARTESIAN_POINT('Ctrl Pts',(-6.94733716327859,49.875,-0.357052332559016));
#41081=CARTESIAN_POINT('Ctrl Pts',(-6.89995030467732,57.495,-0.381845111328231));
#41082=CARTESIAN_POINT('Ctrl Pts',(-6.89995030467732,49.875,-0.381845111328231));
#41083=CARTESIAN_POINT('Ctrl Pts',(-6.85285448604147,57.495,-0.405571362419762));
#41084=CARTESIAN_POINT('Ctrl Pts',(-6.85285448604147,49.875,-0.405571362419762));
#41085=CARTESIAN_POINT('Ctrl Pts',(-6.80606015708944,57.495,-0.428228256434481));
#41086=CARTESIAN_POINT('Ctrl Pts',(-6.80606015708944,49.875,-0.428228256434481));
#41087=CARTESIAN_POINT('Ctrl Pts',(-6.75958168761835,57.495,-0.449817078488634));
#41088=CARTESIAN_POINT('Ctrl Pts',(-6.75958168761835,49.875,-0.449817078488634));
#41089=CARTESIAN_POINT('Ctrl Pts',(-6.71344014059646,57.495,-0.470341429749656));
#41090=CARTESIAN_POINT('Ctrl Pts',(-6.71344014059646,49.875,-0.470341429749656));
#41091=CARTESIAN_POINT('Ctrl Pts',(-6.66766610085612,57.495,-0.48980608847462));
#41092=CARTESIAN_POINT('Ctrl Pts',(-6.66766610085612,49.875,-0.48980608847462));
#41093=CARTESIAN_POINT('Ctrl Pts',(-6.62230172760518,57.495,-0.508215876982667));
#41094=CARTESIAN_POINT('Ctrl Pts',(-6.62230172760518,49.875,-0.508215876982667));
#41095=CARTESIAN_POINT('Ctrl Pts',(-6.57740496530586,57.495,-0.52557467621436));
#41096=CARTESIAN_POINT('Ctrl Pts',(-6.57740496530586,49.875,-0.52557467621436));
#41097=CARTESIAN_POINT('Ctrl Pts',(-6.53304612199338,57.495,-0.541884929839958));
#41098=CARTESIAN_POINT('Ctrl Pts',(-6.53304612199338,49.875,-0.541884929839958));
#41099=CARTESIAN_POINT('Ctrl Pts',(-6.48929587557851,57.495,-0.557147755196287));
#41100=CARTESIAN_POINT('Ctrl Pts',(-6.48929587557851,49.875,-0.557147755196287));
#41101=CARTESIAN_POINT('Ctrl Pts',(-6.4462144738227,57.495,-0.571363102905585));
#41102=CARTESIAN_POINT('Ctrl Pts',(-6.4462144738227,49.875,-0.571363102905585));
#41103=CARTESIAN_POINT('Ctrl Pts',(-6.40384227175349,57.495,-0.584530087032233));
#41104=CARTESIAN_POINT('Ctrl Pts',(-6.40384227175349,49.875,-0.584530087032233));
#41105=CARTESIAN_POINT('Ctrl Pts',(-6.36218460951721,57.495,-0.596647533682195));
#41106=CARTESIAN_POINT('Ctrl Pts',(-6.36218460951721,49.875,-0.596647533682195));
#41107=CARTESIAN_POINT('Ctrl Pts',(-6.32121490697708,57.495,-0.607714431517378));
#41108=CARTESIAN_POINT('Ctrl Pts',(-6.32121490697708,49.875,-0.607714431517378));
#41109=CARTESIAN_POINT('Ctrl Pts',(-6.28091120375433,57.495,-0.617730009530283));
#41110=CARTESIAN_POINT('Ctrl Pts',(-6.28091120375433,49.875,-0.617730009530283));
#41111=CARTESIAN_POINT('Ctrl Pts',(-6.24128706412512,57.495,-0.626694128202827));
#41112=CARTESIAN_POINT('Ctrl Pts',(-6.24128706412512,49.875,-0.626694128202827));
#41113=CARTESIAN_POINT('Ctrl Pts',(-6.2024209037432,57.495,-0.63460770787657));
#41114=CARTESIAN_POINT('Ctrl Pts',(-6.2024209037432,49.875,-0.63460770787657));
#41115=CARTESIAN_POINT('Ctrl Pts',(-6.16449561918681,57.495,-0.641473544543642));
#41116=CARTESIAN_POINT('Ctrl Pts',(-6.16449561918681,49.875,-0.641473544543642));
#41117=CARTESIAN_POINT('Ctrl Pts',(-6.12780215712609,57.495,-0.647296629738964));
#41118=CARTESIAN_POINT('Ctrl Pts',(-6.12780215712609,49.875,-0.647296629738964));
#41119=CARTESIAN_POINT('Ctrl Pts',(-6.092682497423,57.495,-0.652083489461663));
#41120=CARTESIAN_POINT('Ctrl Pts',(-6.092682497423,49.875,-0.652083489461663));
#41121=CARTESIAN_POINT('Ctrl Pts',(-6.05948455921138,57.495,-0.655842009648654));
#41122=CARTESIAN_POINT('Ctrl Pts',(-6.05948455921138,49.875,-0.655842009648654));
#41123=CARTESIAN_POINT('Ctrl Pts',(-6.02851672315009,57.495,-0.658581184594065));
#41124=CARTESIAN_POINT('Ctrl Pts',(-6.02851672315009,49.875,-0.658581184594065));
#41125=CARTESIAN_POINT('Ctrl Pts',(-5.99999062205821,57.495,-0.660311421925919));
#41126=CARTESIAN_POINT('Ctrl Pts',(-5.99999062205821,49.875,-0.660311421925919));
#41127=CARTESIAN_POINT('Ctrl Pts',(-5.97401619058905,57.495,-0.661043615595395));
#41128=CARTESIAN_POINT('Ctrl Pts',(-5.97401619058905,49.875,-0.661043615595395));
#41129=CARTESIAN_POINT('Ctrl Pts',(-5.95531437453421,57.495,-0.660838563360812));
#41130=CARTESIAN_POINT('Ctrl Pts',(-5.95531437453421,49.875,-0.660838563360812));
#41131=CARTESIAN_POINT('Ctrl Pts',(-5.94245897164689,57.495,-0.660242999639131));
#41132=CARTESIAN_POINT('Ctrl Pts',(-5.94245897164689,49.875,-0.660242999639131));
#41133=CARTESIAN_POINT('Ctrl Pts',(-5.93440822125369,57.495,-0.659649967278209));
#41134=CARTESIAN_POINT('Ctrl Pts',(-5.93440822125369,49.875,-0.659649967278209));
#41135=CARTESIAN_POINT('Ctrl Pts',(-5.93051272372135,57.495,-0.659304453656786));
#41136=CARTESIAN_POINT('Ctrl Pts',(-5.93051272372135,49.875,-0.659304453656786));
#41137=CARTESIAN_POINT('Ctrl Pts',(-7.13972463098307,51.145,-0.247119796320916));
#41138=CARTESIAN_POINT('Ctrl Pts',(-7.13000027153814,51.145,-0.253018452443266));
#41139=CARTESIAN_POINT('Ctrl Pts',(-7.1105784652929,51.145,-0.264712515322364));
#41140=CARTESIAN_POINT('Ctrl Pts',(-7.0815264936406,51.145,-0.281943861934803));
#41141=CARTESIAN_POINT('Ctrl Pts',(-7.04295230112448,51.145,-0.304298370266162));
#41142=CARTESIAN_POINT('Ctrl Pts',(-6.99500658045334,51.145,-0.331200384093975));
#41143=CARTESIAN_POINT('Ctrl Pts',(-6.94733716327859,51.145,-0.357052332559016));
#41144=CARTESIAN_POINT('Ctrl Pts',(-6.89995030467732,51.145,-0.381845111328231));
#41145=CARTESIAN_POINT('Ctrl Pts',(-6.85285448604147,51.145,-0.405571362419762));
#41146=CARTESIAN_POINT('Ctrl Pts',(-6.80606015708944,51.145,-0.428228256434481));
#41147=CARTESIAN_POINT('Ctrl Pts',(-6.75958168761835,51.145,-0.449817078488634));
#41148=CARTESIAN_POINT('Ctrl Pts',(-6.71344014059646,51.145,-0.470341429749656));
#41149=CARTESIAN_POINT('Ctrl Pts',(-6.66766610085612,51.145,-0.48980608847462));
#41150=CARTESIAN_POINT('Ctrl Pts',(-6.62230172760518,51.145,-0.508215876982667));
#41151=CARTESIAN_POINT('Ctrl Pts',(-6.57740496530586,51.145,-0.52557467621436));
#41152=CARTESIAN_POINT('Ctrl Pts',(-6.53304612199338,51.145,-0.541884929839958));
#41153=CARTESIAN_POINT('Ctrl Pts',(-6.48929587557851,51.145,-0.557147755196287));
#41154=CARTESIAN_POINT('Ctrl Pts',(-6.4462144738227,51.145,-0.571363102905585));
#41155=CARTESIAN_POINT('Ctrl Pts',(-6.40384227175349,51.145,-0.584530087032233));
#41156=CARTESIAN_POINT('Ctrl Pts',(-6.36218460951721,51.145,-0.596647533682195));
#41157=CARTESIAN_POINT('Ctrl Pts',(-6.32121490697708,51.145,-0.607714431517378));
#41158=CARTESIAN_POINT('Ctrl Pts',(-6.28091120375433,51.145,-0.617730009530283));
#41159=CARTESIAN_POINT('Ctrl Pts',(-6.24128706412512,51.145,-0.626694128202827));
#41160=CARTESIAN_POINT('Ctrl Pts',(-6.2024209037432,51.145,-0.63460770787657));
#41161=CARTESIAN_POINT('Ctrl Pts',(-6.16449561918681,51.145,-0.641473544543642));
#41162=CARTESIAN_POINT('Ctrl Pts',(-6.12780215712609,51.145,-0.647296629738964));
#41163=CARTESIAN_POINT('Ctrl Pts',(-6.092682497423,51.145,-0.652083489461663));
#41164=CARTESIAN_POINT('Ctrl Pts',(-6.05948455921138,51.145,-0.655842009648654));
#41165=CARTESIAN_POINT('Ctrl Pts',(-6.02851672315009,51.145,-0.658581184594065));
#41166=CARTESIAN_POINT('Ctrl Pts',(-5.99999062205821,51.145,-0.660311421925919));
#41167=CARTESIAN_POINT('Ctrl Pts',(-5.97401619058905,51.145,-0.661043615595395));
#41168=CARTESIAN_POINT('Ctrl Pts',(-5.95531437453421,51.145,-0.660838563360812));
#41169=CARTESIAN_POINT('Ctrl Pts',(-5.94245897164689,51.145,-0.660242999639131));
#41170=CARTESIAN_POINT('Ctrl Pts',(-5.93440822125369,51.145,-0.659649967278209));
#41171=CARTESIAN_POINT('Ctrl Pts',(-5.93051272372135,51.145,-0.659304453656786));
#41172=CARTESIAN_POINT('Origin',(0.,54.32,0.));
#41173=CARTESIAN_POINT('',(-5.1463899549833,51.145,1.4909173120086));
#41174=CARTESIAN_POINT('Origin',(0.,51.145,0.));
#41175=CARTESIAN_POINT('',(-5.1463899549833,54.32,1.4909173120086));
#41176=CARTESIAN_POINT('Origin',(-5.73138421404289,57.495,1.66039107437148));
#41177=CARTESIAN_POINT('',(-5.73138421404289,51.145,1.66039107437148));
#41178=CARTESIAN_POINT('',(-5.73138421404289,51.145,1.66039107437148));
#41179=CARTESIAN_POINT('',(-5.73138421404289,57.495,1.66039107437148));
#41180=CARTESIAN_POINT('Origin',(-1.50456066262064E-12,57.495,6.23660068148933E-13));
#41181=CARTESIAN_POINT('',(-6.69081410619341,51.145,2.50394540602692));
#41182=CARTESIAN_POINT('',(-6.69081410619341,57.495,2.50394540602692));
#41183=CARTESIAN_POINT('',(-6.5016768024705,51.145,2.96056324982543));
#41184=CARTESIAN_POINT('Origin',(-1.50456066262064E-12,51.145,6.23660068148933E-13));
#41185=CARTESIAN_POINT('',(-6.5016768024705,57.495,2.96056324982543));
#41186=CARTESIAN_POINT('Ctrl Pts',(-5.22677443144495,57.495,2.87862685522557));
#41187=CARTESIAN_POINT('Ctrl Pts',(-5.22677443144495,49.875,2.87862685522557));
#41188=CARTESIAN_POINT('Ctrl Pts',(-5.23024117954545,57.495,2.88043681055507));
#41189=CARTESIAN_POINT('Ctrl Pts',(-5.23024117954545,49.875,2.88043681055507));
#41190=CARTESIAN_POINT('Ctrl Pts',(-5.2374521593957,57.495,2.88406558980908));
#41191=CARTESIAN_POINT('Ctrl Pts',(-5.2374521593957,49.875,2.88406558980908));
#41192=CARTESIAN_POINT('Ctrl Pts',(-5.24910109063627,57.495,2.88953536864324));
#41193=CARTESIAN_POINT('Ctrl Pts',(-5.24910109063627,49.875,2.88953536864324));
#41194=CARTESIAN_POINT('Ctrl Pts',(-5.26630084561717,57.495,2.8968816873652));
#41195=CARTESIAN_POINT('Ctrl Pts',(-5.26630084561717,49.875,2.8968816873652));
#41196=CARTESIAN_POINT('Ctrl Pts',(-5.29057828960674,57.495,2.90614521320845));
#41197=CARTESIAN_POINT('Ctrl Pts',(-5.29057828960674,49.875,2.90614521320845));
#41198=CARTESIAN_POINT('Ctrl Pts',(-5.31759510370885,57.495,2.91546314862894));
#41199=CARTESIAN_POINT('Ctrl Pts',(-5.31759510370885,49.875,2.91546314862894));
#41200=CARTESIAN_POINT('Ctrl Pts',(-5.34725389048201,57.495,2.92478335875772));
#41201=CARTESIAN_POINT('Ctrl Pts',(-5.34725389048201,49.875,2.92478335875772));
#41202=CARTESIAN_POINT('Ctrl Pts',(-5.37936310952307,57.495,2.93401523982666));
#41203=CARTESIAN_POINT('Ctrl Pts',(-5.37936310952307,49.875,2.93401523982666));
#41204=CARTESIAN_POINT('Ctrl Pts',(-5.41364129622042,57.495,2.94303247002252));
#41205=CARTESIAN_POINT('Ctrl Pts',(-5.41364129622042,49.875,2.94303247002252));
#41206=CARTESIAN_POINT('Ctrl Pts',(-5.44977003302479,57.495,2.95169462080126));
#41207=CARTESIAN_POINT('Ctrl Pts',(-5.44977003302479,49.875,2.95169462080126));
#41208=CARTESIAN_POINT('Ctrl Pts',(-5.48743586913294,57.495,2.95986479289848));
#41209=CARTESIAN_POINT('Ctrl Pts',(-5.48743586913294,49.875,2.95986479289848));
#41210=CARTESIAN_POINT('Ctrl Pts',(-5.52637191504897,57.495,2.96742703426686));
#41211=CARTESIAN_POINT('Ctrl Pts',(-5.52637191504897,49.875,2.96742703426686));
#41212=CARTESIAN_POINT('Ctrl Pts',(-5.56641026634754,57.495,2.97430877025613));
#41213=CARTESIAN_POINT('Ctrl Pts',(-5.56641026634754,49.875,2.97430877025613));
#41214=CARTESIAN_POINT('Ctrl Pts',(-5.60747882861056,57.495,2.98047914221005));
#41215=CARTESIAN_POINT('Ctrl Pts',(-5.60747882861056,49.875,2.98047914221005));
#41216=CARTESIAN_POINT('Ctrl Pts',(-5.64956501668965,57.495,2.98593308820275));
#41217=CARTESIAN_POINT('Ctrl Pts',(-5.64956501668965,49.875,2.98593308820275));
#41218=CARTESIAN_POINT('Ctrl Pts',(-5.6926888242775,57.495,2.99067972442542));
#41219=CARTESIAN_POINT('Ctrl Pts',(-5.6926888242775,49.875,2.99067972442542));
#41220=CARTESIAN_POINT('Ctrl Pts',(-5.7368744211961,57.495,2.99473015701058));
#41221=CARTESIAN_POINT('Ctrl Pts',(-5.7368744211961,49.875,2.99473015701058));
#41222=CARTESIAN_POINT('Ctrl Pts',(-5.78211642456377,57.495,2.99808342690941));
#41223=CARTESIAN_POINT('Ctrl Pts',(-5.78211642456377,49.875,2.99808342690941));
#41224=CARTESIAN_POINT('Ctrl Pts',(-5.82837721216372,57.495,3.00072490941925));
#41225=CARTESIAN_POINT('Ctrl Pts',(-5.82837721216372,49.875,3.00072490941925));
#41226=CARTESIAN_POINT('Ctrl Pts',(-5.87560110342618,57.495,3.00263159433907));
#41227=CARTESIAN_POINT('Ctrl Pts',(-5.87560110342618,49.875,3.00263159433907));
#41228=CARTESIAN_POINT('Ctrl Pts',(-5.92372322806235,57.495,3.00377540211876));
#41229=CARTESIAN_POINT('Ctrl Pts',(-5.92372322806235,49.875,3.00377540211876));
#41230=CARTESIAN_POINT('Ctrl Pts',(-5.97267956506957,57.495,3.00412716938111));
#41231=CARTESIAN_POINT('Ctrl Pts',(-5.97267956506957,49.875,3.00412716938111));
#41232=CARTESIAN_POINT('Ctrl Pts',(-6.02241806591683,57.495,3.00366113621889));
#41233=CARTESIAN_POINT('Ctrl Pts',(-6.02241806591683,49.875,3.00366113621889));
#41234=CARTESIAN_POINT('Ctrl Pts',(-6.07290162599645,57.495,3.00235671375975));
#41235=CARTESIAN_POINT('Ctrl Pts',(-6.07290162599645,49.875,3.00235671375975));
#41236=CARTESIAN_POINT('Ctrl Pts',(-6.12410381716763,57.495,3.00019778316116));
#41237=CARTESIAN_POINT('Ctrl Pts',(-6.12410381716763,49.875,3.00019778316116));
#41238=CARTESIAN_POINT('Ctrl Pts',(-6.1760065578922,57.495,2.99717295692923));
#41239=CARTESIAN_POINT('Ctrl Pts',(-6.1760065578922,49.875,2.99717295692923));
#41240=CARTESIAN_POINT('Ctrl Pts',(-6.22859706400143,57.495,2.9932755486881));
#41241=CARTESIAN_POINT('Ctrl Pts',(-6.22859706400143,49.875,2.9932755486881));
#41242=CARTESIAN_POINT('Ctrl Pts',(-6.28186459845025,57.495,2.98850417352762));
#41243=CARTESIAN_POINT('Ctrl Pts',(-6.28186459845025,49.875,2.98850417352762));
#41244=CARTESIAN_POINT('Ctrl Pts',(-6.33579850967655,57.495,2.98286238364847));
#41245=CARTESIAN_POINT('Ctrl Pts',(-6.33579850967655,49.875,2.98286238364847));
#41246=CARTESIAN_POINT('Ctrl Pts',(-6.39038953466525,57.495,2.97635619664327));
#41247=CARTESIAN_POINT('Ctrl Pts',(-6.39038953466525,49.875,2.97635619664327));
#41248=CARTESIAN_POINT('Ctrl Pts',(-6.43458214159119,57.495,2.97046502832937));
#41249=CARTESIAN_POINT('Ctrl Pts',(-6.43458214159119,49.875,2.97046502832937));
#41250=CARTESIAN_POINT('Ctrl Pts',(-6.4680168144459,57.495,2.96566304810545));
#41251=CARTESIAN_POINT('Ctrl Pts',(-6.4680168144459,49.875,2.96566304810545));
#41252=CARTESIAN_POINT('Ctrl Pts',(-6.49043534784125,57.495,2.96229154623624));
#41253=CARTESIAN_POINT('Ctrl Pts',(-6.49043534784125,49.875,2.96229154623624));
#41254=CARTESIAN_POINT('Ctrl Pts',(-6.5016768024705,57.495,2.96056324982543));
#41255=CARTESIAN_POINT('Ctrl Pts',(-6.5016768024705,49.875,2.96056324982543));
#41256=CARTESIAN_POINT('',(-5.22677443144495,51.145,2.87862685522557));
#41257=CARTESIAN_POINT('Ctrl Pts',(-5.22677443144495,51.145,2.87862685522557));
#41258=CARTESIAN_POINT('Ctrl Pts',(-5.23024117954545,51.145,2.88043681055507));
#41259=CARTESIAN_POINT('Ctrl Pts',(-5.2374521593957,51.145,2.88406558980908));
#41260=CARTESIAN_POINT('Ctrl Pts',(-5.24910109063627,51.145,2.88953536864324));
#41261=CARTESIAN_POINT('Ctrl Pts',(-5.26630084561717,51.145,2.8968816873652));
#41262=CARTESIAN_POINT('Ctrl Pts',(-5.29057828960674,51.145,2.90614521320845));
#41263=CARTESIAN_POINT('Ctrl Pts',(-5.31759510370885,51.145,2.91546314862894));
#41264=CARTESIAN_POINT('Ctrl Pts',(-5.34725389048201,51.145,2.92478335875772));
#41265=CARTESIAN_POINT('Ctrl Pts',(-5.37936310952307,51.145,2.93401523982666));
#41266=CARTESIAN_POINT('Ctrl Pts',(-5.41364129622042,51.145,2.94303247002252));
#41267=CARTESIAN_POINT('Ctrl Pts',(-5.44977003302479,51.145,2.95169462080126));
#41268=CARTESIAN_POINT('Ctrl Pts',(-5.48743586913294,51.145,2.95986479289848));
#41269=CARTESIAN_POINT('Ctrl Pts',(-5.52637191504897,51.145,2.96742703426686));
#41270=CARTESIAN_POINT('Ctrl Pts',(-5.56641026634754,51.145,2.97430877025613));
#41271=CARTESIAN_POINT('Ctrl Pts',(-5.60747882861056,51.145,2.98047914221005));
#41272=CARTESIAN_POINT('Ctrl Pts',(-5.64956501668965,51.145,2.98593308820275));
#41273=CARTESIAN_POINT('Ctrl Pts',(-5.6926888242775,51.145,2.99067972442542));
#41274=CARTESIAN_POINT('Ctrl Pts',(-5.7368744211961,51.145,2.99473015701058));
#41275=CARTESIAN_POINT('Ctrl Pts',(-5.78211642456377,51.145,2.99808342690941));
#41276=CARTESIAN_POINT('Ctrl Pts',(-5.82837721216372,51.145,3.00072490941925));
#41277=CARTESIAN_POINT('Ctrl Pts',(-5.87560110342618,51.145,3.00263159433907));
#41278=CARTESIAN_POINT('Ctrl Pts',(-5.92372322806235,51.145,3.00377540211876));
#41279=CARTESIAN_POINT('Ctrl Pts',(-5.97267956506957,51.145,3.00412716938111));
#41280=CARTESIAN_POINT('Ctrl Pts',(-6.02241806591683,51.145,3.00366113621889));
#41281=CARTESIAN_POINT('Ctrl Pts',(-6.07290162599645,51.145,3.00235671375975));
#41282=CARTESIAN_POINT('Ctrl Pts',(-6.12410381716763,51.145,3.00019778316116));
#41283=CARTESIAN_POINT('Ctrl Pts',(-6.1760065578922,51.145,2.99717295692923));
#41284=CARTESIAN_POINT('Ctrl Pts',(-6.22859706400143,51.145,2.9932755486881));
#41285=CARTESIAN_POINT('Ctrl Pts',(-6.28186459845025,51.145,2.98850417352762));
#41286=CARTESIAN_POINT('Ctrl Pts',(-6.33579850967655,51.145,2.98286238364847));
#41287=CARTESIAN_POINT('Ctrl Pts',(-6.39038953466525,51.145,2.97635619664327));
#41288=CARTESIAN_POINT('Ctrl Pts',(-6.43458214159119,51.145,2.97046502832937));
#41289=CARTESIAN_POINT('Ctrl Pts',(-6.4680168144459,51.145,2.96566304810545));
#41290=CARTESIAN_POINT('Ctrl Pts',(-6.49043534784125,51.145,2.96229154623624));
#41291=CARTESIAN_POINT('Ctrl Pts',(-6.5016768024705,51.145,2.96056324982543));
#41292=CARTESIAN_POINT('',(-5.22677443144495,57.495,2.87862685522557));
#41293=CARTESIAN_POINT('Origin',(-4.56189402049717,57.495,2.51244640654327));
#41294=CARTESIAN_POINT('',(-4.69328497730872,51.145,2.58480949428933));
#41295=CARTESIAN_POINT('',(-4.69328497730872,54.32,2.58480949428933));
#41296=CARTESIAN_POINT('',(-4.56189402049717,51.145,2.51244640654327));
#41297=CARTESIAN_POINT('Ctrl Pts',(-6.69081410619341,57.495,2.50394540602692));
#41298=CARTESIAN_POINT('Ctrl Pts',(-6.69081410619341,49.875,2.50394540602692));
#41299=CARTESIAN_POINT('Ctrl Pts',(-6.6840872875067,57.495,2.49477440711622));
#41300=CARTESIAN_POINT('Ctrl Pts',(-6.6840872875067,49.875,2.49477440711622));
#41301=CARTESIAN_POINT('Ctrl Pts',(-6.67061900235319,57.495,2.47653809829367));
#41302=CARTESIAN_POINT('Ctrl Pts',(-6.67061900235319,49.875,2.47653809829367));
#41303=CARTESIAN_POINT('Ctrl Pts',(-6.65037263123044,57.495,2.44950070161195));
#41304=CARTESIAN_POINT('Ctrl Pts',(-6.65037263123044,49.875,2.44950070161195));
#41305=CARTESIAN_POINT('Ctrl Pts',(-6.62328942425873,57.495,2.41408612451247));
#41306=CARTESIAN_POINT('Ctrl Pts',(-6.62328942425873,49.875,2.41408612451247));
#41307=CARTESIAN_POINT('Ctrl Pts',(-6.58928830924833,57.495,2.37088387159997));
#41308=CARTESIAN_POINT('Ctrl Pts',(-6.58928830924833,49.875,2.37088387159997));
#41309=CARTESIAN_POINT('Ctrl Pts',(-6.55514062276576,57.495,2.32875748935431));
#41310=CARTESIAN_POINT('Ctrl Pts',(-6.55514062276576,49.875,2.32875748935431));
#41311=CARTESIAN_POINT('Ctrl Pts',(-6.52084865967131,57.495,2.28771778279682));
#41312=CARTESIAN_POINT('Ctrl Pts',(-6.52084865967131,49.875,2.28771778279682));
#41313=CARTESIAN_POINT('Ctrl Pts',(-6.48641743997165,57.495,2.24777479550452));
#41314=CARTESIAN_POINT('Ctrl Pts',(-6.48641743997165,49.875,2.24777479550452));
#41315=CARTESIAN_POINT('Ctrl Pts',(-6.45185553518355,57.495,2.20893514043546));
#41316=CARTESIAN_POINT('Ctrl Pts',(-6.45185553518355,49.875,2.20893514043546));
#41317=CARTESIAN_POINT('Ctrl Pts',(-6.41717671306116,57.495,2.17120312938032));
#41318=CARTESIAN_POINT('Ctrl Pts',(-6.41717671306116,49.875,2.17120312938032));
#41319=CARTESIAN_POINT('Ctrl Pts',(-6.38240181135686,57.495,2.13458349574322));
#41320=CARTESIAN_POINT('Ctrl Pts',(-6.38240181135686,49.875,2.13458349574322));
#41321=CARTESIAN_POINT('Ctrl Pts',(-6.34756091533109,57.495,2.09908352929886));
#41322=CARTESIAN_POINT('Ctrl Pts',(-6.34756091533109,49.875,2.09908352929886));
#41323=CARTESIAN_POINT('Ctrl Pts',(-6.31269482043472,57.495,2.06471490843565));
#41324=CARTESIAN_POINT('Ctrl Pts',(-6.31269482043472,49.875,2.06471490843565));
#41325=CARTESIAN_POINT('Ctrl Pts',(-6.27785854554207,57.495,2.03149622201774));
#41326=CARTESIAN_POINT('Ctrl Pts',(-6.27785854554207,49.875,2.03149622201774));
#41327=CARTESIAN_POINT('Ctrl Pts',(-6.24311798195999,57.495,1.99945211810842));
#41328=CARTESIAN_POINT('Ctrl Pts',(-6.24311798195999,49.875,1.99945211810842));
#41329=CARTESIAN_POINT('Ctrl Pts',(-6.20853885514991,57.495,1.96860861168855));
#41330=CARTESIAN_POINT('Ctrl Pts',(-6.20853885514991,49.875,1.96860861168855));
#41331=CARTESIAN_POINT('Ctrl Pts',(-6.17417680788948,57.495,1.93898880419738));
#41332=CARTESIAN_POINT('Ctrl Pts',(-6.17417680788948,49.875,1.93898880419738));
#41333=CARTESIAN_POINT('Ctrl Pts',(-6.14006878432979,57.495,1.91060895733316));
#41334=CARTESIAN_POINT('Ctrl Pts',(-6.14006878432979,49.875,1.91060895733316));
#41335=CARTESIAN_POINT('Ctrl Pts',(-6.10621926889293,57.495,1.88347219921807));
#41336=CARTESIAN_POINT('Ctrl Pts',(-6.10621926889293,49.875,1.88347219921807));
#41337=CARTESIAN_POINT('Ctrl Pts',(-6.07260331771224,57.495,1.85756929242873));
#41338=CARTESIAN_POINT('Ctrl Pts',(-6.07260331771224,49.875,1.85756929242873));
#41339=CARTESIAN_POINT('Ctrl Pts',(-6.03920034699142,57.495,1.83289254541003));
#41340=CARTESIAN_POINT('Ctrl Pts',(-6.03920034699142,49.875,1.83289254541003));
#41341=CARTESIAN_POINT('Ctrl Pts',(-6.00602283509636,57.495,1.80944727788364));
#41342=CARTESIAN_POINT('Ctrl Pts',(-6.00602283509636,49.875,1.80944727788364));
#41343=CARTESIAN_POINT('Ctrl Pts',(-5.97314358084405,57.495,1.78726264793637));
#41344=CARTESIAN_POINT('Ctrl Pts',(-5.97314358084405,49.875,1.78726264793637));
#41345=CARTESIAN_POINT('Ctrl Pts',(-5.94073262861954,57.495,1.76640606389863));
#41346=CARTESIAN_POINT('Ctrl Pts',(-5.94073262861954,49.875,1.76640606389863));
#41347=CARTESIAN_POINT('Ctrl Pts',(-5.90906068827417,57.495,1.74698425466385));
#41348=CARTESIAN_POINT('Ctrl Pts',(-5.90906068827417,49.875,1.74698425466385));
#41349=CARTESIAN_POINT('Ctrl Pts',(-5.87844620539466,57.495,1.72912206102237));
#41350=CARTESIAN_POINT('Ctrl Pts',(-5.87844620539466,49.875,1.72912206102237));
#41351=CARTESIAN_POINT('Ctrl Pts',(-5.84921363316514,57.495,1.71294534020681));
#41352=CARTESIAN_POINT('Ctrl Pts',(-5.84921363316514,49.875,1.71294534020681));
#41353=CARTESIAN_POINT('Ctrl Pts',(-5.8216513201319,57.495,1.69856379474193));
#41354=CARTESIAN_POINT('Ctrl Pts',(-5.8216513201319,49.875,1.69856379474193));
#41355=CARTESIAN_POINT('Ctrl Pts',(-5.79595877235173,57.495,1.68604879760681));
#41356=CARTESIAN_POINT('Ctrl Pts',(-5.79595877235173,49.875,1.68604879760681));
#41357=CARTESIAN_POINT('Ctrl Pts',(-5.77224172513534,57.495,1.67543235427339));
#41358=CARTESIAN_POINT('Ctrl Pts',(-5.77224172513534,49.875,1.67543235427339));
#41359=CARTESIAN_POINT('Ctrl Pts',(-5.75488502996854,57.495,1.66846492267669));
#41360=CARTESIAN_POINT('Ctrl Pts',(-5.75488502996854,49.875,1.66846492267669));
#41361=CARTESIAN_POINT('Ctrl Pts',(-5.74278027398956,57.495,1.6640956021081));
#41362=CARTESIAN_POINT('Ctrl Pts',(-5.74278027398956,49.875,1.6640956021081));
#41363=CARTESIAN_POINT('Ctrl Pts',(-5.73511540682054,57.495,1.66156260377489));
#41364=CARTESIAN_POINT('Ctrl Pts',(-5.73511540682054,49.875,1.66156260377489));
#41365=CARTESIAN_POINT('Ctrl Pts',(-5.73138421404289,57.495,1.66039107437148));
#41366=CARTESIAN_POINT('Ctrl Pts',(-5.73138421404289,49.875,1.66039107437148));
#41367=CARTESIAN_POINT('Ctrl Pts',(-6.69081410619341,51.145,2.50394540602692));
#41368=CARTESIAN_POINT('Ctrl Pts',(-6.6840872875067,51.145,2.49477440711622));
#41369=CARTESIAN_POINT('Ctrl Pts',(-6.67061900235319,51.145,2.47653809829367));
#41370=CARTESIAN_POINT('Ctrl Pts',(-6.65037263123044,51.145,2.44950070161195));
#41371=CARTESIAN_POINT('Ctrl Pts',(-6.62328942425873,51.145,2.41408612451247));
#41372=CARTESIAN_POINT('Ctrl Pts',(-6.58928830924833,51.145,2.37088387159997));
#41373=CARTESIAN_POINT('Ctrl Pts',(-6.55514062276576,51.145,2.32875748935431));
#41374=CARTESIAN_POINT('Ctrl Pts',(-6.52084865967131,51.145,2.28771778279682));
#41375=CARTESIAN_POINT('Ctrl Pts',(-6.48641743997165,51.145,2.24777479550452));
#41376=CARTESIAN_POINT('Ctrl Pts',(-6.45185553518355,51.145,2.20893514043546));
#41377=CARTESIAN_POINT('Ctrl Pts',(-6.41717671306116,51.145,2.17120312938032));
#41378=CARTESIAN_POINT('Ctrl Pts',(-6.38240181135686,51.145,2.13458349574322));
#41379=CARTESIAN_POINT('Ctrl Pts',(-6.34756091533109,51.145,2.09908352929886));
#41380=CARTESIAN_POINT('Ctrl Pts',(-6.31269482043472,51.145,2.06471490843565));
#41381=CARTESIAN_POINT('Ctrl Pts',(-6.27785854554207,51.145,2.03149622201774));
#41382=CARTESIAN_POINT('Ctrl Pts',(-6.24311798195999,51.145,1.99945211810842));
#41383=CARTESIAN_POINT('Ctrl Pts',(-6.20853885514991,51.145,1.96860861168855));
#41384=CARTESIAN_POINT('Ctrl Pts',(-6.17417680788948,51.145,1.93898880419738));
#41385=CARTESIAN_POINT('Ctrl Pts',(-6.14006878432979,51.145,1.91060895733316));
#41386=CARTESIAN_POINT('Ctrl Pts',(-6.10621926889293,51.145,1.88347219921807));
#41387=CARTESIAN_POINT('Ctrl Pts',(-6.07260331771224,51.145,1.85756929242873));
#41388=CARTESIAN_POINT('Ctrl Pts',(-6.03920034699142,51.145,1.83289254541003));
#41389=CARTESIAN_POINT('Ctrl Pts',(-6.00602283509636,51.145,1.80944727788364));
#41390=CARTESIAN_POINT('Ctrl Pts',(-5.97314358084405,51.145,1.78726264793637));
#41391=CARTESIAN_POINT('Ctrl Pts',(-5.94073262861954,51.145,1.76640606389863));
#41392=CARTESIAN_POINT('Ctrl Pts',(-5.90906068827417,51.145,1.74698425466385));
#41393=CARTESIAN_POINT('Ctrl Pts',(-5.87844620539466,51.145,1.72912206102237));
#41394=CARTESIAN_POINT('Ctrl Pts',(-5.84921363316514,51.145,1.71294534020681));
#41395=CARTESIAN_POINT('Ctrl Pts',(-5.8216513201319,51.145,1.69856379474193));
#41396=CARTESIAN_POINT('Ctrl Pts',(-5.79595877235173,51.145,1.68604879760681));
#41397=CARTESIAN_POINT('Ctrl Pts',(-5.77224172513534,51.145,1.67543235427339));
#41398=CARTESIAN_POINT('Ctrl Pts',(-5.75488502996854,51.145,1.66846492267669));
#41399=CARTESIAN_POINT('Ctrl Pts',(-5.74278027398956,51.145,1.6640956021081));
#41400=CARTESIAN_POINT('Ctrl Pts',(-5.73511540682054,51.145,1.66156260377489));
#41401=CARTESIAN_POINT('Ctrl Pts',(-5.73138421404289,51.145,1.66039107437148));
#41402=CARTESIAN_POINT('Origin',(0.,54.32,0.));
#41403=CARTESIAN_POINT('',(-4.18409499139877,51.145,3.34686616149372));
#41404=CARTESIAN_POINT('Origin',(0.,51.145,0.));
#41405=CARTESIAN_POINT('',(-4.18409499139877,54.32,3.34686616149372));
#41406=CARTESIAN_POINT('Origin',(-4.65970441290367,57.495,3.72730711280926));
#41407=CARTESIAN_POINT('',(-4.65970441290367,51.145,3.72730711280926));
#41408=CARTESIAN_POINT('',(-4.65970441290367,51.145,3.72730711280926));
#41409=CARTESIAN_POINT('',(-4.65970441290367,57.495,3.72730711280926));
#41410=CARTESIAN_POINT('Origin',(-1.15136842610855E-12,57.495,1.15195721078055E-12));
#41411=CARTESIAN_POINT('',(-5.22328778611671,51.145,4.87380761862879));
#41412=CARTESIAN_POINT('',(-5.22328778611671,57.495,4.87380761862879));
#41413=CARTESIAN_POINT('',(-4.87380761862879,51.145,5.22328778611671));
#41414=CARTESIAN_POINT('Origin',(-1.15136842610855E-12,51.145,1.15195721078055E-12));
#41415=CARTESIAN_POINT('',(-4.87380761862879,57.495,5.22328778611671));
#41416=CARTESIAN_POINT('Ctrl Pts',(-3.72730711280926,57.495,4.65970441290367));
#41417=CARTESIAN_POINT('Ctrl Pts',(-3.72730711280926,49.875,4.65970441290367));
#41418=CARTESIAN_POINT('Ctrl Pts',(-3.72981733050576,57.495,4.66270326064961));
#41419=CARTESIAN_POINT('Ctrl Pts',(-3.72981733050576,49.875,4.66270326064961));
#41420=CARTESIAN_POINT('Ctrl Pts',(-3.73509073349854,57.495,4.6688153380502));
#41421=CARTESIAN_POINT('Ctrl Pts',(-3.73509073349854,49.875,4.6688153380502));
#41422=CARTESIAN_POINT('Ctrl Pts',(-3.7437597489088,57.495,4.67832660775297));
#41423=CARTESIAN_POINT('Ctrl Pts',(-3.7437597489088,49.875,4.67832660775297));
#41424=CARTESIAN_POINT('Ctrl Pts',(-3.7568389360361,57.495,4.69169578253142));
#41425=CARTESIAN_POINT('Ctrl Pts',(-3.7568389360361,49.875,4.69169578253142));
#41426=CARTESIAN_POINT('Ctrl Pts',(-3.77572337177426,57.495,4.70954474005187));
#41427=CARTESIAN_POINT('Ctrl Pts',(-3.77572337177426,49.875,4.70954474005187));
#41428=CARTESIAN_POINT('Ctrl Pts',(-3.79711783384759,57.495,4.72849227702429));
#41429=CARTESIAN_POINT('Ctrl Pts',(-3.79711783384759,49.875,4.72849227702429));
#41430=CARTESIAN_POINT('Ctrl Pts',(-3.82095228990398,57.495,4.74845295472311));
#41431=CARTESIAN_POINT('Ctrl Pts',(-3.82095228990398,49.875,4.74845295472311));
#41432=CARTESIAN_POINT('Ctrl Pts',(-3.84708445224628,57.495,4.76926976684248));
#41433=CARTESIAN_POINT('Ctrl Pts',(-3.84708445224628,49.875,4.76926976684248));
#41434=CARTESIAN_POINT('Ctrl Pts',(-3.87530262274579,57.495,4.79071829540097));
#41435=CARTESIAN_POINT('Ctrl Pts',(-3.87530262274579,49.875,4.79071829540097));
#41436=CARTESIAN_POINT('Ctrl Pts',(-3.90536636162316,57.495,4.81254694822028));
#41437=CARTESIAN_POINT('Ctrl Pts',(-3.90536636162316,49.875,4.81254694822028));
#41438=CARTESIAN_POINT('Ctrl Pts',(-3.93703846717723,57.495,4.83450929444277));
#41439=CARTESIAN_POINT('Ctrl Pts',(-3.93703846717723,49.875,4.83450929444277));
#41440=CARTESIAN_POINT('Ctrl Pts',(-3.97011673859275,57.495,4.85639607415679));
#41441=CARTESIAN_POINT('Ctrl Pts',(-3.97011673859275,49.875,4.85639607415679));
#41442=CARTESIAN_POINT('Ctrl Pts',(-4.00447382552398,57.495,4.8780759828866));
#41443=CARTESIAN_POINT('Ctrl Pts',(-4.00447382552398,49.875,4.8780759828866));
#41444=CARTESIAN_POINT('Ctrl Pts',(-4.04005493051016,57.495,4.89949292161193));
#41445=CARTESIAN_POINT('Ctrl Pts',(-4.04005493051016,49.875,4.89949292161193));
#41446=CARTESIAN_POINT('Ctrl Pts',(-4.07685036350543,57.495,4.92063739759527));
#41447=CARTESIAN_POINT('Ctrl Pts',(-4.07685036350543,49.875,4.92063739759527));
#41448=CARTESIAN_POINT('Ctrl Pts',(-4.11487510765792,57.495,4.94152548435404));
#41449=CARTESIAN_POINT('Ctrl Pts',(-4.11487510765792,49.875,4.94152548435404));
#41450=CARTESIAN_POINT('Ctrl Pts',(-4.15414724283855,57.495,4.9621766920072));
#41451=CARTESIAN_POINT('Ctrl Pts',(-4.15414724283855,49.875,4.9621766920072));
#41452=CARTESIAN_POINT('Ctrl Pts',(-4.19466216292523,57.495,4.98258807456953));
#41453=CARTESIAN_POINT('Ctrl Pts',(-4.19466216292523,49.875,4.98258807456953));
#41454=CARTESIAN_POINT('Ctrl Pts',(-4.23639070615327,57.495,5.00273172317852));
#41455=CARTESIAN_POINT('Ctrl Pts',(-4.23639070615327,49.875,5.00273172317852));
#41456=CARTESIAN_POINT('Ctrl Pts',(-4.27929023600664,57.495,5.02256507114883));
#41457=CARTESIAN_POINT('Ctrl Pts',(-4.27929023600664,49.875,5.02256507114883));
#41458=CARTESIAN_POINT('Ctrl Pts',(-4.32331156573186,57.495,5.04203735157409));
#41459=CARTESIAN_POINT('Ctrl Pts',(-4.32331156573186,49.875,5.04203735157409));
#41460=CARTESIAN_POINT('Ctrl Pts',(-4.36840670797621,57.495,5.06109712122993));
#41461=CARTESIAN_POINT('Ctrl Pts',(-4.36840670797621,49.875,5.06109712122993));
#41462=CARTESIAN_POINT('Ctrl Pts',(-4.41453743405689,57.495,5.07970066295481));
#41463=CARTESIAN_POINT('Ctrl Pts',(-4.41453743405689,49.875,5.07970066295481));
#41464=CARTESIAN_POINT('Ctrl Pts',(-4.46167734280668,57.495,5.09781475579234));
#41465=CARTESIAN_POINT('Ctrl Pts',(-4.46167734280668,49.875,5.09781475579234));
#41466=CARTESIAN_POINT('Ctrl Pts',(-4.50980818622117,57.495,5.11541439426219));
#41467=CARTESIAN_POINT('Ctrl Pts',(-4.50980818622117,49.875,5.11541439426219));
#41468=CARTESIAN_POINT('Ctrl Pts',(-4.55891761694258,57.495,5.13248213818673));
#41469=CARTESIAN_POINT('Ctrl Pts',(-4.55891761694258,49.875,5.13248213818673));
#41470=CARTESIAN_POINT('Ctrl Pts',(-4.60899638270436,57.495,5.14900691787061));
#41471=CARTESIAN_POINT('Ctrl Pts',(-4.60899638270436,49.875,5.14900691787061));
#41472=CARTESIAN_POINT('Ctrl Pts',(-4.66003509375248,57.495,5.16498334493441));
#41473=CARTESIAN_POINT('Ctrl Pts',(-4.66003509375248,49.875,5.16498334493441));
#41474=CARTESIAN_POINT('Ctrl Pts',(-4.71202254995837,57.495,5.1804106250073));
#41475=CARTESIAN_POINT('Ctrl Pts',(-4.71202254995837,49.875,5.1804106250073));
#41476=CARTESIAN_POINT('Ctrl Pts',(-4.764947890579,57.495,5.1952907728175));
#41477=CARTESIAN_POINT('Ctrl Pts',(-4.764947890579,49.875,5.1952907728175));
#41478=CARTESIAN_POINT('Ctrl Pts',(-4.8080309881172,57.495,5.2067598214933));
#41479=CARTESIAN_POINT('Ctrl Pts',(-4.8080309881172,49.875,5.2067598214933));
#41480=CARTESIAN_POINT('Ctrl Pts',(-4.84075823631812,57.495,5.21511826561693));
#41481=CARTESIAN_POINT('Ctrl Pts',(-4.84075823631812,49.875,5.21511826561693));
#41482=CARTESIAN_POINT('Ctrl Pts',(-4.86276047837854,57.495,5.22058260535447));
#41483=CARTESIAN_POINT('Ctrl Pts',(-4.86276047837854,49.875,5.22058260535447));
#41484=CARTESIAN_POINT('Ctrl Pts',(-4.87380761862879,57.495,5.22328778611671));
#41485=CARTESIAN_POINT('Ctrl Pts',(-4.87380761862879,49.875,5.22328778611671));
#41486=CARTESIAN_POINT('',(-3.72730711280926,51.145,4.65970441290367));
#41487=CARTESIAN_POINT('Ctrl Pts',(-3.72730711280926,51.145,4.65970441290367));
#41488=CARTESIAN_POINT('Ctrl Pts',(-3.72981733050576,51.145,4.66270326064961));
#41489=CARTESIAN_POINT('Ctrl Pts',(-3.73509073349854,51.145,4.6688153380502));
#41490=CARTESIAN_POINT('Ctrl Pts',(-3.7437597489088,51.145,4.67832660775297));
#41491=CARTESIAN_POINT('Ctrl Pts',(-3.7568389360361,51.145,4.69169578253142));
#41492=CARTESIAN_POINT('Ctrl Pts',(-3.77572337177426,51.145,4.70954474005187));
#41493=CARTESIAN_POINT('Ctrl Pts',(-3.79711783384759,51.145,4.72849227702429));
#41494=CARTESIAN_POINT('Ctrl Pts',(-3.82095228990398,51.145,4.74845295472311));
#41495=CARTESIAN_POINT('Ctrl Pts',(-3.84708445224628,51.145,4.76926976684248));
#41496=CARTESIAN_POINT('Ctrl Pts',(-3.87530262274579,51.145,4.79071829540097));
#41497=CARTESIAN_POINT('Ctrl Pts',(-3.90536636162316,51.145,4.81254694822028));
#41498=CARTESIAN_POINT('Ctrl Pts',(-3.93703846717723,51.145,4.83450929444277));
#41499=CARTESIAN_POINT('Ctrl Pts',(-3.97011673859275,51.145,4.85639607415679));
#41500=CARTESIAN_POINT('Ctrl Pts',(-4.00447382552398,51.145,4.8780759828866));
#41501=CARTESIAN_POINT('Ctrl Pts',(-4.04005493051016,51.145,4.89949292161193));
#41502=CARTESIAN_POINT('Ctrl Pts',(-4.07685036350543,51.145,4.92063739759527));
#41503=CARTESIAN_POINT('Ctrl Pts',(-4.11487510765792,51.145,4.94152548435404));
#41504=CARTESIAN_POINT('Ctrl Pts',(-4.15414724283855,51.145,4.9621766920072));
#41505=CARTESIAN_POINT('Ctrl Pts',(-4.19466216292523,51.145,4.98258807456953));
#41506=CARTESIAN_POINT('Ctrl Pts',(-4.23639070615327,51.145,5.00273172317852));
#41507=CARTESIAN_POINT('Ctrl Pts',(-4.27929023600664,51.145,5.02256507114883));
#41508=CARTESIAN_POINT('Ctrl Pts',(-4.32331156573186,51.145,5.04203735157409));
#41509=CARTESIAN_POINT('Ctrl Pts',(-4.36840670797621,51.145,5.06109712122993));
#41510=CARTESIAN_POINT('Ctrl Pts',(-4.41453743405689,51.145,5.07970066295481));
#41511=CARTESIAN_POINT('Ctrl Pts',(-4.46167734280668,51.145,5.09781475579234));
#41512=CARTESIAN_POINT('Ctrl Pts',(-4.50980818622117,51.145,5.11541439426219));
#41513=CARTESIAN_POINT('Ctrl Pts',(-4.55891761694258,51.145,5.13248213818673));
#41514=CARTESIAN_POINT('Ctrl Pts',(-4.60899638270436,51.145,5.14900691787061));
#41515=CARTESIAN_POINT('Ctrl Pts',(-4.66003509375248,51.145,5.16498334493441));
#41516=CARTESIAN_POINT('Ctrl Pts',(-4.71202254995837,51.145,5.1804106250073));
#41517=CARTESIAN_POINT('Ctrl Pts',(-4.764947890579,51.145,5.1952907728175));
#41518=CARTESIAN_POINT('Ctrl Pts',(-4.8080309881172,51.145,5.2067598214933));
#41519=CARTESIAN_POINT('Ctrl Pts',(-4.84075823631812,51.145,5.21511826561693));
#41520=CARTESIAN_POINT('Ctrl Pts',(-4.86276047837854,51.145,5.22058260535447));
#41521=CARTESIAN_POINT('Ctrl Pts',(-4.87380761862879,51.145,5.22328778611671));
#41522=CARTESIAN_POINT('',(-3.72730711280926,57.495,4.65970441290367));
#41523=CARTESIAN_POINT('Origin',(-3.25316890053365,57.495,4.06695907338649));
#41524=CARTESIAN_POINT('',(-3.34686616149372,51.145,4.18409499139877));
#41525=CARTESIAN_POINT('',(-3.34686616149372,54.32,4.18409499139877));
#41526=CARTESIAN_POINT('',(-3.25316890053365,51.145,4.06695907338649));
#41527=CARTESIAN_POINT('Ctrl Pts',(-5.22328778611671,57.495,4.87380761862879));
#41528=CARTESIAN_POINT('Ctrl Pts',(-5.22328778611671,49.875,4.87380761862879));
#41529=CARTESIAN_POINT('Ctrl Pts',(-5.22058260535451,57.495,4.86276047837859));
#41530=CARTESIAN_POINT('Ctrl Pts',(-5.22058260535451,49.875,4.86276047837859));
#41531=CARTESIAN_POINT('Ctrl Pts',(-5.21511826561704,57.495,4.84075823631825));
#41532=CARTESIAN_POINT('Ctrl Pts',(-5.21511826561704,49.875,4.84075823631825));
#41533=CARTESIAN_POINT('Ctrl Pts',(-5.20675982149348,57.495,4.80803098811744));
#41534=CARTESIAN_POINT('Ctrl Pts',(-5.20675982149348,49.875,4.80803098811744));
#41535=CARTESIAN_POINT('Ctrl Pts',(-5.19529077281773,57.495,4.7649478905793));
#41536=CARTESIAN_POINT('Ctrl Pts',(-5.19529077281773,49.875,4.7649478905793));
#41537=CARTESIAN_POINT('Ctrl Pts',(-5.18041062500752,57.495,4.71202254995864));
#41538=CARTESIAN_POINT('Ctrl Pts',(-5.18041062500752,49.875,4.71202254995864));
#41539=CARTESIAN_POINT('Ctrl Pts',(-5.16498334493456,57.495,4.66003509375265));
#41540=CARTESIAN_POINT('Ctrl Pts',(-5.16498334493456,49.875,4.66003509375265));
#41541=CARTESIAN_POINT('Ctrl Pts',(-5.14900691787064,57.495,4.60899638270439));
#41542=CARTESIAN_POINT('Ctrl Pts',(-5.14900691787064,49.875,4.60899638270439));
#41543=CARTESIAN_POINT('Ctrl Pts',(-5.13248213818666,57.495,4.5589176169425));
#41544=CARTESIAN_POINT('Ctrl Pts',(-5.13248213818666,49.875,4.5589176169425));
#41545=CARTESIAN_POINT('Ctrl Pts',(-5.11541439426204,57.495,4.50980818622101));
#41546=CARTESIAN_POINT('Ctrl Pts',(-5.11541439426204,49.875,4.50980818622101));
#41547=CARTESIAN_POINT('Ctrl Pts',(-5.09781475579217,57.495,4.4616773428065));
#41548=CARTESIAN_POINT('Ctrl Pts',(-5.09781475579217,49.875,4.4616773428065));
#41549=CARTESIAN_POINT('Ctrl Pts',(-5.07970066295468,57.495,4.41453743405677));
#41550=CARTESIAN_POINT('Ctrl Pts',(-5.07970066295468,49.875,4.41453743405677));
#41551=CARTESIAN_POINT('Ctrl Pts',(-5.06109712122989,57.495,4.36840670797617));
#41552=CARTESIAN_POINT('Ctrl Pts',(-5.06109712122989,49.875,4.36840670797617));
#41553=CARTESIAN_POINT('Ctrl Pts',(-5.04203735157413,57.495,4.3233115657319));
#41554=CARTESIAN_POINT('Ctrl Pts',(-5.04203735157413,49.875,4.3233115657319));
#41555=CARTESIAN_POINT('Ctrl Pts',(-5.02256507114894,57.495,4.27929023600674));
#41556=CARTESIAN_POINT('Ctrl Pts',(-5.02256507114894,49.875,4.27929023600674));
#41557=CARTESIAN_POINT('Ctrl Pts',(-5.00273172317863,57.495,4.23639070615337));
#41558=CARTESIAN_POINT('Ctrl Pts',(-5.00273172317863,49.875,4.23639070615337));
#41559=CARTESIAN_POINT('Ctrl Pts',(-4.98258807456962,57.495,4.1946621629253));
#41560=CARTESIAN_POINT('Ctrl Pts',(-4.98258807456962,49.875,4.1946621629253));
#41561=CARTESIAN_POINT('Ctrl Pts',(-4.96217669200723,57.495,4.15414724283858));
#41562=CARTESIAN_POINT('Ctrl Pts',(-4.96217669200723,49.875,4.15414724283858));
#41563=CARTESIAN_POINT('Ctrl Pts',(-4.94152548435402,57.495,4.11487510765791));
#41564=CARTESIAN_POINT('Ctrl Pts',(-4.94152548435402,49.875,4.11487510765791));
#41565=CARTESIAN_POINT('Ctrl Pts',(-4.92063739759521,57.495,4.07685036350539));
#41566=CARTESIAN_POINT('Ctrl Pts',(-4.92063739759521,49.875,4.07685036350539));
#41567=CARTESIAN_POINT('Ctrl Pts',(-4.89949292161185,57.495,4.04005493051012));
#41568=CARTESIAN_POINT('Ctrl Pts',(-4.89949292161185,49.875,4.04005493051012));
#41569=CARTESIAN_POINT('Ctrl Pts',(-4.87807598288654,57.495,4.00447382552396));
#41570=CARTESIAN_POINT('Ctrl Pts',(-4.87807598288654,49.875,4.00447382552396));
#41571=CARTESIAN_POINT('Ctrl Pts',(-4.85639607415676,57.495,3.97011673859274));
#41572=CARTESIAN_POINT('Ctrl Pts',(-4.85639607415676,49.875,3.97011673859274));
#41573=CARTESIAN_POINT('Ctrl Pts',(-4.83450929444279,57.495,3.93703846717724));
#41574=CARTESIAN_POINT('Ctrl Pts',(-4.83450929444279,49.875,3.93703846717724));
#41575=CARTESIAN_POINT('Ctrl Pts',(-4.81254694822034,57.495,3.90536636162318));
#41576=CARTESIAN_POINT('Ctrl Pts',(-4.81254694822034,49.875,3.90536636162318));
#41577=CARTESIAN_POINT('Ctrl Pts',(-4.79071829540103,57.495,3.8753026227458));
#41578=CARTESIAN_POINT('Ctrl Pts',(-4.79071829540103,49.875,3.8753026227458));
#41579=CARTESIAN_POINT('Ctrl Pts',(-4.76926976684252,57.495,3.84708445224627));
#41580=CARTESIAN_POINT('Ctrl Pts',(-4.76926976684252,49.875,3.84708445224627));
#41581=CARTESIAN_POINT('Ctrl Pts',(-4.74845295472312,57.495,3.82095228990397));
#41582=CARTESIAN_POINT('Ctrl Pts',(-4.74845295472312,49.875,3.82095228990397));
#41583=CARTESIAN_POINT('Ctrl Pts',(-4.72849227702427,57.495,3.7971178338476));
#41584=CARTESIAN_POINT('Ctrl Pts',(-4.72849227702427,49.875,3.7971178338476));
#41585=CARTESIAN_POINT('Ctrl Pts',(-4.7095447400518,57.495,3.77572337177431));
#41586=CARTESIAN_POINT('Ctrl Pts',(-4.7095447400518,49.875,3.77572337177431));
#41587=CARTESIAN_POINT('Ctrl Pts',(-4.69169578253132,57.495,3.75683893603616));
#41588=CARTESIAN_POINT('Ctrl Pts',(-4.69169578253132,49.875,3.75683893603616));
#41589=CARTESIAN_POINT('Ctrl Pts',(-4.67832660775287,57.495,3.74375974890886));
#41590=CARTESIAN_POINT('Ctrl Pts',(-4.67832660775287,49.875,3.74375974890886));
#41591=CARTESIAN_POINT('Ctrl Pts',(-4.66881533805013,57.495,3.73509073349858));
#41592=CARTESIAN_POINT('Ctrl Pts',(-4.66881533805013,49.875,3.73509073349858));
#41593=CARTESIAN_POINT('Ctrl Pts',(-4.66270326064959,57.495,3.72981733050578));
#41594=CARTESIAN_POINT('Ctrl Pts',(-4.66270326064959,49.875,3.72981733050578));
#41595=CARTESIAN_POINT('Ctrl Pts',(-4.65970441290367,57.495,3.72730711280926));
#41596=CARTESIAN_POINT('Ctrl Pts',(-4.65970441290367,49.875,3.72730711280926));
#41597=CARTESIAN_POINT('Ctrl Pts',(-5.22328778611671,51.145,4.87380761862879));
#41598=CARTESIAN_POINT('Ctrl Pts',(-5.22058260535451,51.145,4.86276047837859));
#41599=CARTESIAN_POINT('Ctrl Pts',(-5.21511826561704,51.145,4.84075823631825));
#41600=CARTESIAN_POINT('Ctrl Pts',(-5.20675982149348,51.145,4.80803098811744));
#41601=CARTESIAN_POINT('Ctrl Pts',(-5.19529077281773,51.145,4.7649478905793));
#41602=CARTESIAN_POINT('Ctrl Pts',(-5.18041062500752,51.145,4.71202254995864));
#41603=CARTESIAN_POINT('Ctrl Pts',(-5.16498334493456,51.145,4.66003509375265));
#41604=CARTESIAN_POINT('Ctrl Pts',(-5.14900691787064,51.145,4.60899638270439));
#41605=CARTESIAN_POINT('Ctrl Pts',(-5.13248213818666,51.145,4.5589176169425));
#41606=CARTESIAN_POINT('Ctrl Pts',(-5.11541439426204,51.145,4.50980818622101));
#41607=CARTESIAN_POINT('Ctrl Pts',(-5.09781475579217,51.145,4.4616773428065));
#41608=CARTESIAN_POINT('Ctrl Pts',(-5.07970066295468,51.145,4.41453743405677));
#41609=CARTESIAN_POINT('Ctrl Pts',(-5.06109712122989,51.145,4.36840670797617));
#41610=CARTESIAN_POINT('Ctrl Pts',(-5.04203735157413,51.145,4.3233115657319));
#41611=CARTESIAN_POINT('Ctrl Pts',(-5.02256507114894,51.145,4.27929023600674));
#41612=CARTESIAN_POINT('Ctrl Pts',(-5.00273172317863,51.145,4.23639070615337));
#41613=CARTESIAN_POINT('Ctrl Pts',(-4.98258807456962,51.145,4.1946621629253));
#41614=CARTESIAN_POINT('Ctrl Pts',(-4.96217669200723,51.145,4.15414724283858));
#41615=CARTESIAN_POINT('Ctrl Pts',(-4.94152548435402,51.145,4.11487510765791));
#41616=CARTESIAN_POINT('Ctrl Pts',(-4.92063739759521,51.145,4.07685036350539));
#41617=CARTESIAN_POINT('Ctrl Pts',(-4.89949292161185,51.145,4.04005493051012));
#41618=CARTESIAN_POINT('Ctrl Pts',(-4.87807598288654,51.145,4.00447382552396));
#41619=CARTESIAN_POINT('Ctrl Pts',(-4.85639607415676,51.145,3.97011673859274));
#41620=CARTESIAN_POINT('Ctrl Pts',(-4.83450929444279,51.145,3.93703846717724));
#41621=CARTESIAN_POINT('Ctrl Pts',(-4.81254694822034,51.145,3.90536636162318));
#41622=CARTESIAN_POINT('Ctrl Pts',(-4.79071829540103,51.145,3.8753026227458));
#41623=CARTESIAN_POINT('Ctrl Pts',(-4.76926976684252,51.145,3.84708445224627));
#41624=CARTESIAN_POINT('Ctrl Pts',(-4.74845295472312,51.145,3.82095228990397));
#41625=CARTESIAN_POINT('Ctrl Pts',(-4.72849227702427,51.145,3.7971178338476));
#41626=CARTESIAN_POINT('Ctrl Pts',(-4.7095447400518,51.145,3.77572337177431));
#41627=CARTESIAN_POINT('Ctrl Pts',(-4.69169578253132,51.145,3.75683893603616));
#41628=CARTESIAN_POINT('Ctrl Pts',(-4.67832660775287,51.145,3.74375974890886));
#41629=CARTESIAN_POINT('Ctrl Pts',(-4.66881533805013,51.145,3.73509073349858));
#41630=CARTESIAN_POINT('Ctrl Pts',(-4.66270326064959,51.145,3.72981733050578));
#41631=CARTESIAN_POINT('Ctrl Pts',(-4.65970441290367,51.145,3.72730711280926));
#41632=CARTESIAN_POINT('Origin',(0.,54.32,0.));
#41633=CARTESIAN_POINT('',(-2.58480949428933,51.145,4.69328497730872));
#41634=CARTESIAN_POINT('Origin',(0.,51.145,0.));
#41635=CARTESIAN_POINT('',(-2.58480949428933,54.32,4.69328497730872));
#41636=CARTESIAN_POINT('Origin',(-1.4491783055134,57.495,5.00231408838243));
#41637=CARTESIAN_POINT('',(-1.4909173120086,51.145,5.1463899549833));
#41638=CARTESIAN_POINT('',(-1.4909173120086,54.32,5.1463899549833));
#41639=CARTESIAN_POINT('',(-1.66039107437148,51.145,5.73138421404289));
#41640=CARTESIAN_POINT('',(-1.66039107437148,57.495,5.73138421404289));
#41641=CARTESIAN_POINT('',(-1.4491783055134,51.145,5.00231408838243));
#41642=CARTESIAN_POINT('Origin',(-2.87862685522557,57.495,5.22677443144495));
#41643=CARTESIAN_POINT('',(-2.87862685522557,51.145,5.22677443144495));
#41644=CARTESIAN_POINT('',(-2.87862685522557,51.145,5.22677443144495));
#41645=CARTESIAN_POINT('',(-2.87862685522557,57.495,5.22677443144495));
#41646=CARTESIAN_POINT('Origin',(-6.22890783902202E-13,57.495,1.50487931058895E-12));
#41647=CARTESIAN_POINT('',(-2.96056324982543,51.145,6.50167680247051));
#41648=CARTESIAN_POINT('',(-2.96056324982543,57.495,6.50167680247051));
#41649=CARTESIAN_POINT('',(-2.50394540602692,51.145,6.69081410619341));
#41650=CARTESIAN_POINT('Origin',(-6.22890783902202E-13,51.145,1.50487931058895E-12));
#41651=CARTESIAN_POINT('',(-2.50394540602692,57.495,6.69081410619341));
#41652=CARTESIAN_POINT('Ctrl Pts',(-1.66039107437148,57.495,5.73138421404289));
#41653=CARTESIAN_POINT('Ctrl Pts',(-1.66039107437148,49.875,5.73138421404289));
#41654=CARTESIAN_POINT('Ctrl Pts',(-1.66156260377487,57.495,5.73511540682056));
#41655=CARTESIAN_POINT('Ctrl Pts',(-1.66156260377487,49.875,5.73511540682056));
#41656=CARTESIAN_POINT('Ctrl Pts',(-1.66409560210805,57.495,5.7427802739896));
#41657=CARTESIAN_POINT('Ctrl Pts',(-1.66409560210805,49.875,5.7427802739896));
#41658=CARTESIAN_POINT('Ctrl Pts',(-1.6684649226766,57.495,5.75488502996861));
#41659=CARTESIAN_POINT('Ctrl Pts',(-1.6684649226766,49.875,5.75488502996861));
#41660=CARTESIAN_POINT('Ctrl Pts',(-1.67543235427329,57.495,5.77224172513541));
#41661=CARTESIAN_POINT('Ctrl Pts',(-1.67543235427329,49.875,5.77224172513541));
#41662=CARTESIAN_POINT('Ctrl Pts',(-1.68604879760674,57.495,5.79595877235177));
#41663=CARTESIAN_POINT('Ctrl Pts',(-1.68604879760674,49.875,5.79595877235177));
#41664=CARTESIAN_POINT('Ctrl Pts',(-1.69856379474191,57.495,5.82165132013192));
#41665=CARTESIAN_POINT('Ctrl Pts',(-1.69856379474191,49.875,5.82165132013192));
#41666=CARTESIAN_POINT('Ctrl Pts',(-1.71294534020683,57.495,5.84921363316513));
#41667=CARTESIAN_POINT('Ctrl Pts',(-1.71294534020683,49.875,5.84921363316513));
#41668=CARTESIAN_POINT('Ctrl Pts',(-1.7291220610224,57.495,5.87844620539462));
#41669=CARTESIAN_POINT('Ctrl Pts',(-1.7291220610224,49.875,5.87844620539462));
#41670=CARTESIAN_POINT('Ctrl Pts',(-1.74698425466387,57.495,5.90906068827411));
#41671=CARTESIAN_POINT('Ctrl Pts',(-1.74698425466387,49.875,5.90906068827411));
#41672=CARTESIAN_POINT('Ctrl Pts',(-1.76640606389864,57.495,5.94073262861949));
#41673=CARTESIAN_POINT('Ctrl Pts',(-1.76640606389864,49.875,5.94073262861949));
#41674=CARTESIAN_POINT('Ctrl Pts',(-1.78726264793636,57.495,5.97314358084403));
#41675=CARTESIAN_POINT('Ctrl Pts',(-1.78726264793636,49.875,5.97314358084403));
#41676=CARTESIAN_POINT('Ctrl Pts',(-1.80944727788364,57.495,6.0060228350964));
#41677=CARTESIAN_POINT('Ctrl Pts',(-1.80944727788364,49.875,6.0060228350964));
#41678=CARTESIAN_POINT('Ctrl Pts',(-1.83289254541003,57.495,6.03920034699149));
#41679=CARTESIAN_POINT('Ctrl Pts',(-1.83289254541003,49.875,6.03920034699149));
#41680=CARTESIAN_POINT('Ctrl Pts',(-1.85756929242873,57.495,6.07260331771232));
#41681=CARTESIAN_POINT('Ctrl Pts',(-1.85756929242873,49.875,6.07260331771232));
#41682=CARTESIAN_POINT('Ctrl Pts',(-1.88347219921808,57.495,6.10621926889299));
#41683=CARTESIAN_POINT('Ctrl Pts',(-1.88347219921808,49.875,6.10621926889299));
#41684=CARTESIAN_POINT('Ctrl Pts',(-1.91060895733317,57.495,6.14006878432982));
#41685=CARTESIAN_POINT('Ctrl Pts',(-1.91060895733317,49.875,6.14006878432982));
#41686=CARTESIAN_POINT('Ctrl Pts',(-1.93898880419737,57.495,6.17417680788945));
#41687=CARTESIAN_POINT('Ctrl Pts',(-1.93898880419737,49.875,6.17417680788945));
#41688=CARTESIAN_POINT('Ctrl Pts',(-1.96860861168851,57.495,6.20853885514981));
#41689=CARTESIAN_POINT('Ctrl Pts',(-1.96860861168851,49.875,6.20853885514981));
#41690=CARTESIAN_POINT('Ctrl Pts',(-1.99945211810837,57.495,6.24311798195985));
#41691=CARTESIAN_POINT('Ctrl Pts',(-1.99945211810837,49.875,6.24311798195985));
#41692=CARTESIAN_POINT('Ctrl Pts',(-2.03149622201768,57.495,6.27785854554194));
#41693=CARTESIAN_POINT('Ctrl Pts',(-2.03149622201768,49.875,6.27785854554194));
#41694=CARTESIAN_POINT('Ctrl Pts',(-2.06471490843563,57.495,6.31269482043467));
#41695=CARTESIAN_POINT('Ctrl Pts',(-2.06471490843563,49.875,6.31269482043467));
#41696=CARTESIAN_POINT('Ctrl Pts',(-2.09908352929888,57.495,6.34756091533115));
#41697=CARTESIAN_POINT('Ctrl Pts',(-2.09908352929888,49.875,6.34756091533115));
#41698=CARTESIAN_POINT('Ctrl Pts',(-2.13458349574329,57.495,6.38240181135703));
#41699=CARTESIAN_POINT('Ctrl Pts',(-2.13458349574329,49.875,6.38240181135703));
#41700=CARTESIAN_POINT('Ctrl Pts',(-2.17120312938042,57.495,6.41717671306138));
#41701=CARTESIAN_POINT('Ctrl Pts',(-2.17120312938042,49.875,6.41717671306138));
#41702=CARTESIAN_POINT('Ctrl Pts',(-2.20893514043555,57.495,6.45185553518375));
#41703=CARTESIAN_POINT('Ctrl Pts',(-2.20893514043555,49.875,6.45185553518375));
#41704=CARTESIAN_POINT('Ctrl Pts',(-2.24777479550457,57.495,6.48641743997175));
#41705=CARTESIAN_POINT('Ctrl Pts',(-2.24777479550457,49.875,6.48641743997175));
#41706=CARTESIAN_POINT('Ctrl Pts',(-2.2877177827968,57.495,6.52084865967127));
#41707=CARTESIAN_POINT('Ctrl Pts',(-2.2877177827968,49.875,6.52084865967127));
#41708=CARTESIAN_POINT('Ctrl Pts',(-2.32875748935421,57.495,6.55514062276556));
#41709=CARTESIAN_POINT('Ctrl Pts',(-2.32875748935421,49.875,6.55514062276556));
#41710=CARTESIAN_POINT('Ctrl Pts',(-2.37088387159981,57.495,6.58928830924802));
#41711=CARTESIAN_POINT('Ctrl Pts',(-2.37088387159981,49.875,6.58928830924802));
#41712=CARTESIAN_POINT('Ctrl Pts',(-2.41408612451229,57.495,6.6232894242584));
#41713=CARTESIAN_POINT('Ctrl Pts',(-2.41408612451229,49.875,6.6232894242584));
#41714=CARTESIAN_POINT('Ctrl Pts',(-2.4495007016118,57.495,6.65037263123018));
#41715=CARTESIAN_POINT('Ctrl Pts',(-2.4495007016118,49.875,6.65037263123018));
#41716=CARTESIAN_POINT('Ctrl Pts',(-2.47653809829358,57.495,6.67061900235304));
#41717=CARTESIAN_POINT('Ctrl Pts',(-2.47653809829358,49.875,6.67061900235304));
#41718=CARTESIAN_POINT('Ctrl Pts',(-2.49477440711619,57.495,6.68408728750664));
#41719=CARTESIAN_POINT('Ctrl Pts',(-2.49477440711619,49.875,6.68408728750664));
#41720=CARTESIAN_POINT('Ctrl Pts',(-2.50394540602692,57.495,6.69081410619341));
#41721=CARTESIAN_POINT('Ctrl Pts',(-2.50394540602692,49.875,6.69081410619341));
#41722=CARTESIAN_POINT('Ctrl Pts',(-1.66039107437148,51.145,5.73138421404289));
#41723=CARTESIAN_POINT('Ctrl Pts',(-1.66156260377487,51.145,5.73511540682056));
#41724=CARTESIAN_POINT('Ctrl Pts',(-1.66409560210805,51.145,5.7427802739896));
#41725=CARTESIAN_POINT('Ctrl Pts',(-1.6684649226766,51.145,5.75488502996861));
#41726=CARTESIAN_POINT('Ctrl Pts',(-1.67543235427329,51.145,5.77224172513541));
#41727=CARTESIAN_POINT('Ctrl Pts',(-1.68604879760674,51.145,5.79595877235177));
#41728=CARTESIAN_POINT('Ctrl Pts',(-1.69856379474191,51.145,5.82165132013192));
#41729=CARTESIAN_POINT('Ctrl Pts',(-1.71294534020683,51.145,5.84921363316513));
#41730=CARTESIAN_POINT('Ctrl Pts',(-1.7291220610224,51.145,5.87844620539462));
#41731=CARTESIAN_POINT('Ctrl Pts',(-1.74698425466387,51.145,5.90906068827411));
#41732=CARTESIAN_POINT('Ctrl Pts',(-1.76640606389864,51.145,5.94073262861949));
#41733=CARTESIAN_POINT('Ctrl Pts',(-1.78726264793636,51.145,5.97314358084403));
#41734=CARTESIAN_POINT('Ctrl Pts',(-1.80944727788364,51.145,6.0060228350964));
#41735=CARTESIAN_POINT('Ctrl Pts',(-1.83289254541003,51.145,6.03920034699149));
#41736=CARTESIAN_POINT('Ctrl Pts',(-1.85756929242873,51.145,6.07260331771232));
#41737=CARTESIAN_POINT('Ctrl Pts',(-1.88347219921808,51.145,6.10621926889299));
#41738=CARTESIAN_POINT('Ctrl Pts',(-1.91060895733317,51.145,6.14006878432982));
#41739=CARTESIAN_POINT('Ctrl Pts',(-1.93898880419737,51.145,6.17417680788945));
#41740=CARTESIAN_POINT('Ctrl Pts',(-1.96860861168851,51.145,6.20853885514981));
#41741=CARTESIAN_POINT('Ctrl Pts',(-1.99945211810837,51.145,6.24311798195985));
#41742=CARTESIAN_POINT('Ctrl Pts',(-2.03149622201768,51.145,6.27785854554194));
#41743=CARTESIAN_POINT('Ctrl Pts',(-2.06471490843563,51.145,6.31269482043467));
#41744=CARTESIAN_POINT('Ctrl Pts',(-2.09908352929888,51.145,6.34756091533115));
#41745=CARTESIAN_POINT('Ctrl Pts',(-2.13458349574329,51.145,6.38240181135703));
#41746=CARTESIAN_POINT('Ctrl Pts',(-2.17120312938042,51.145,6.41717671306138));
#41747=CARTESIAN_POINT('Ctrl Pts',(-2.20893514043555,51.145,6.45185553518375));
#41748=CARTESIAN_POINT('Ctrl Pts',(-2.24777479550457,51.145,6.48641743997175));
#41749=CARTESIAN_POINT('Ctrl Pts',(-2.2877177827968,51.145,6.52084865967127));
#41750=CARTESIAN_POINT('Ctrl Pts',(-2.32875748935421,51.145,6.55514062276556));
#41751=CARTESIAN_POINT('Ctrl Pts',(-2.37088387159981,51.145,6.58928830924802));
#41752=CARTESIAN_POINT('Ctrl Pts',(-2.41408612451229,51.145,6.6232894242584));
#41753=CARTESIAN_POINT('Ctrl Pts',(-2.4495007016118,51.145,6.65037263123018));
#41754=CARTESIAN_POINT('Ctrl Pts',(-2.47653809829358,51.145,6.67061900235304));
#41755=CARTESIAN_POINT('Ctrl Pts',(-2.49477440711619,51.145,6.68408728750664));
#41756=CARTESIAN_POINT('Ctrl Pts',(-2.50394540602692,51.145,6.69081410619341));
#41757=CARTESIAN_POINT('Ctrl Pts',(-2.96056324982543,57.495,6.50167680247051));
#41758=CARTESIAN_POINT('Ctrl Pts',(-2.96056324982543,49.875,6.50167680247051));
#41759=CARTESIAN_POINT('Ctrl Pts',(-2.96229154623625,57.495,6.49043534784131));
#41760=CARTESIAN_POINT('Ctrl Pts',(-2.96229154623625,49.875,6.49043534784131));
#41761=CARTESIAN_POINT('Ctrl Pts',(-2.96566304810549,57.495,6.46801681444607));
#41762=CARTESIAN_POINT('Ctrl Pts',(-2.96566304810549,49.875,6.46801681444607));
#41763=CARTESIAN_POINT('Ctrl Pts',(-2.97046502832945,57.495,6.43458214159149));
#41764=CARTESIAN_POINT('Ctrl Pts',(-2.97046502832945,49.875,6.43458214159149));
#41765=CARTESIAN_POINT('Ctrl Pts',(-2.97635619664337,57.495,6.39038953466561));
#41766=CARTESIAN_POINT('Ctrl Pts',(-2.97635619664337,49.875,6.39038953466561));
#41767=CARTESIAN_POINT('Ctrl Pts',(-2.98286238364857,57.495,6.33579850967689));
#41768=CARTESIAN_POINT('Ctrl Pts',(-2.98286238364857,49.875,6.33579850967689));
#41769=CARTESIAN_POINT('Ctrl Pts',(-2.98850417352769,57.495,6.28186459845047));
#41770=CARTESIAN_POINT('Ctrl Pts',(-2.98850417352769,49.875,6.28186459845047));
#41771=CARTESIAN_POINT('Ctrl Pts',(-2.99327554868811,57.495,6.22859706400147));
#41772=CARTESIAN_POINT('Ctrl Pts',(-2.99327554868811,49.875,6.22859706400147));
#41773=CARTESIAN_POINT('Ctrl Pts',(-2.99717295692919,57.495,6.17600655789209));
#41774=CARTESIAN_POINT('Ctrl Pts',(-2.99717295692919,49.875,6.17600655789209));
#41775=CARTESIAN_POINT('Ctrl Pts',(-3.00019778316108,57.495,6.12410381716742));
#41776=CARTESIAN_POINT('Ctrl Pts',(-3.00019778316108,49.875,6.12410381716742));
#41777=CARTESIAN_POINT('Ctrl Pts',(-3.00235671375967,57.495,6.07290162599622));
#41778=CARTESIAN_POINT('Ctrl Pts',(-3.00235671375967,49.875,6.07290162599622));
#41779=CARTESIAN_POINT('Ctrl Pts',(-3.00366113621883,57.495,6.02241806591666));
#41780=CARTESIAN_POINT('Ctrl Pts',(-3.00366113621883,49.875,6.02241806591666));
#41781=CARTESIAN_POINT('Ctrl Pts',(-3.00412716938109,57.495,5.97267956506952));
#41782=CARTESIAN_POINT('Ctrl Pts',(-3.00412716938109,49.875,5.97267956506952));
#41783=CARTESIAN_POINT('Ctrl Pts',(-3.00377540211877,57.495,5.9237232280624));
#41784=CARTESIAN_POINT('Ctrl Pts',(-3.00377540211877,49.875,5.9237232280624));
#41785=CARTESIAN_POINT('Ctrl Pts',(-3.00263159433912,57.495,5.87560110342631));
#41786=CARTESIAN_POINT('Ctrl Pts',(-3.00263159433912,49.875,5.87560110342631));
#41787=CARTESIAN_POINT('Ctrl Pts',(-3.00072490941932,57.495,5.82837721216385));
#41788=CARTESIAN_POINT('Ctrl Pts',(-3.00072490941932,49.875,5.82837721216385));
#41789=CARTESIAN_POINT('Ctrl Pts',(-2.99808342690946,57.495,5.78211642456387));
#41790=CARTESIAN_POINT('Ctrl Pts',(-2.99808342690946,49.875,5.78211642456387));
#41791=CARTESIAN_POINT('Ctrl Pts',(-2.9947301570106,57.495,5.73687442119613));
#41792=CARTESIAN_POINT('Ctrl Pts',(-2.9947301570106,49.875,5.73687442119613));
#41793=CARTESIAN_POINT('Ctrl Pts',(-2.9906797244254,57.495,5.69268882427748));
#41794=CARTESIAN_POINT('Ctrl Pts',(-2.9906797244254,49.875,5.69268882427748));
#41795=CARTESIAN_POINT('Ctrl Pts',(-2.98593308820271,57.495,5.64956501668959));
#41796=CARTESIAN_POINT('Ctrl Pts',(-2.98593308820271,49.875,5.64956501668959));
#41797=CARTESIAN_POINT('Ctrl Pts',(-2.98047914221,57.495,5.6074788286105));
#41798=CARTESIAN_POINT('Ctrl Pts',(-2.98047914221,49.875,5.6074788286105));
#41799=CARTESIAN_POINT('Ctrl Pts',(-2.97430877025609,57.495,5.56641026634749));
#41800=CARTESIAN_POINT('Ctrl Pts',(-2.97430877025609,49.875,5.56641026634749));
#41801=CARTESIAN_POINT('Ctrl Pts',(-2.96742703426683,57.495,5.52637191504895));
#41802=CARTESIAN_POINT('Ctrl Pts',(-2.96742703426683,49.875,5.52637191504895));
#41803=CARTESIAN_POINT('Ctrl Pts',(-2.9598647928985,57.495,5.48743586913296));
#41804=CARTESIAN_POINT('Ctrl Pts',(-2.9598647928985,49.875,5.48743586913296));
#41805=CARTESIAN_POINT('Ctrl Pts',(-2.95169462080131,57.495,5.44977003302482));
#41806=CARTESIAN_POINT('Ctrl Pts',(-2.95169462080131,49.875,5.44977003302482));
#41807=CARTESIAN_POINT('Ctrl Pts',(-2.94303247002258,57.495,5.41364129622045));
#41808=CARTESIAN_POINT('Ctrl Pts',(-2.94303247002258,49.875,5.41364129622045));
#41809=CARTESIAN_POINT('Ctrl Pts',(-2.93401523982671,57.495,5.37936310952307));
#41810=CARTESIAN_POINT('Ctrl Pts',(-2.93401523982671,49.875,5.37936310952307));
#41811=CARTESIAN_POINT('Ctrl Pts',(-2.92478335875774,57.495,5.34725389048201));
#41812=CARTESIAN_POINT('Ctrl Pts',(-2.92478335875774,49.875,5.34725389048201));
#41813=CARTESIAN_POINT('Ctrl Pts',(-2.91546314862891,57.495,5.31759510370885));
#41814=CARTESIAN_POINT('Ctrl Pts',(-2.91546314862891,49.875,5.31759510370885));
#41815=CARTESIAN_POINT('Ctrl Pts',(-2.90614521320837,57.495,5.29057828960676));
#41816=CARTESIAN_POINT('Ctrl Pts',(-2.90614521320837,49.875,5.29057828960676));
#41817=CARTESIAN_POINT('Ctrl Pts',(-2.89688168736508,57.495,5.26630084561719));
#41818=CARTESIAN_POINT('Ctrl Pts',(-2.89688168736508,49.875,5.26630084561719));
#41819=CARTESIAN_POINT('Ctrl Pts',(-2.88953536864313,57.495,5.24910109063628));
#41820=CARTESIAN_POINT('Ctrl Pts',(-2.88953536864313,49.875,5.24910109063628));
#41821=CARTESIAN_POINT('Ctrl Pts',(-2.884065589809,57.495,5.23745215939571));
#41822=CARTESIAN_POINT('Ctrl Pts',(-2.884065589809,49.875,5.23745215939571));
#41823=CARTESIAN_POINT('Ctrl Pts',(-2.88043681055505,57.495,5.23024117954545));
#41824=CARTESIAN_POINT('Ctrl Pts',(-2.88043681055505,49.875,5.23024117954545));
#41825=CARTESIAN_POINT('Ctrl Pts',(-2.87862685522557,57.495,5.22677443144495));
#41826=CARTESIAN_POINT('Ctrl Pts',(-2.87862685522557,49.875,5.22677443144495));
#41827=CARTESIAN_POINT('Ctrl Pts',(-2.96056324982543,51.145,6.50167680247051));
#41828=CARTESIAN_POINT('Ctrl Pts',(-2.96229154623625,51.145,6.49043534784131));
#41829=CARTESIAN_POINT('Ctrl Pts',(-2.96566304810549,51.145,6.46801681444607));
#41830=CARTESIAN_POINT('Ctrl Pts',(-2.97046502832945,51.145,6.43458214159149));
#41831=CARTESIAN_POINT('Ctrl Pts',(-2.97635619664337,51.145,6.39038953466561));
#41832=CARTESIAN_POINT('Ctrl Pts',(-2.98286238364857,51.145,6.33579850967689));
#41833=CARTESIAN_POINT('Ctrl Pts',(-2.98850417352769,51.145,6.28186459845047));
#41834=CARTESIAN_POINT('Ctrl Pts',(-2.99327554868811,51.145,6.22859706400147));
#41835=CARTESIAN_POINT('Ctrl Pts',(-2.99717295692919,51.145,6.17600655789209));
#41836=CARTESIAN_POINT('Ctrl Pts',(-3.00019778316108,51.145,6.12410381716742));
#41837=CARTESIAN_POINT('Ctrl Pts',(-3.00235671375967,51.145,6.07290162599622));
#41838=CARTESIAN_POINT('Ctrl Pts',(-3.00366113621883,51.145,6.02241806591666));
#41839=CARTESIAN_POINT('Ctrl Pts',(-3.00412716938109,51.145,5.97267956506952));
#41840=CARTESIAN_POINT('Ctrl Pts',(-3.00377540211877,51.145,5.9237232280624));
#41841=CARTESIAN_POINT('Ctrl Pts',(-3.00263159433912,51.145,5.87560110342631));
#41842=CARTESIAN_POINT('Ctrl Pts',(-3.00072490941932,51.145,5.82837721216385));
#41843=CARTESIAN_POINT('Ctrl Pts',(-2.99808342690946,51.145,5.78211642456387));
#41844=CARTESIAN_POINT('Ctrl Pts',(-2.9947301570106,51.145,5.73687442119613));
#41845=CARTESIAN_POINT('Ctrl Pts',(-2.9906797244254,51.145,5.69268882427748));
#41846=CARTESIAN_POINT('Ctrl Pts',(-2.98593308820271,51.145,5.64956501668959));
#41847=CARTESIAN_POINT('Ctrl Pts',(-2.98047914221,51.145,5.6074788286105));
#41848=CARTESIAN_POINT('Ctrl Pts',(-2.97430877025609,51.145,5.56641026634749));
#41849=CARTESIAN_POINT('Ctrl Pts',(-2.96742703426683,51.145,5.52637191504895));
#41850=CARTESIAN_POINT('Ctrl Pts',(-2.9598647928985,51.145,5.48743586913296));
#41851=CARTESIAN_POINT('Ctrl Pts',(-2.95169462080131,51.145,5.44977003302482));
#41852=CARTESIAN_POINT('Ctrl Pts',(-2.94303247002258,51.145,5.41364129622045));
#41853=CARTESIAN_POINT('Ctrl Pts',(-2.93401523982671,51.145,5.37936310952307));
#41854=CARTESIAN_POINT('Ctrl Pts',(-2.92478335875774,51.145,5.34725389048201));
#41855=CARTESIAN_POINT('Ctrl Pts',(-2.91546314862891,51.145,5.31759510370885));
#41856=CARTESIAN_POINT('Ctrl Pts',(-2.90614521320837,51.145,5.29057828960676));
#41857=CARTESIAN_POINT('Ctrl Pts',(-2.89688168736508,51.145,5.26630084561719));
#41858=CARTESIAN_POINT('Ctrl Pts',(-2.88953536864313,51.145,5.24910109063628));
#41859=CARTESIAN_POINT('Ctrl Pts',(-2.884065589809,51.145,5.23745215939571));
#41860=CARTESIAN_POINT('Ctrl Pts',(-2.88043681055505,51.145,5.23024117954545));
#41861=CARTESIAN_POINT('Ctrl Pts',(-2.87862685522557,51.145,5.22677443144495));
#41862=CARTESIAN_POINT('Origin',(3.261,51.145,0.));
#41863=CARTESIAN_POINT('',(0.592010183030744,51.145,5.32519370006274));
#41864=CARTESIAN_POINT('Origin',(0.,51.145,0.));
#41865=CARTESIAN_POINT('',(0.659304453656788,51.145,5.93051272372135));
#41866=CARTESIAN_POINT('',(0.575436549687218,51.145,5.17611212951227));
#41867=CARTESIAN_POINT('',(0.24711979632092,51.145,7.13972463098307));
#41868=CARTESIAN_POINT('Ctrl Pts',(0.659304453656788,51.145,5.93051272372135));
#41869=CARTESIAN_POINT('Ctrl Pts',(0.659649967278236,51.145,5.9344082212537));
#41870=CARTESIAN_POINT('Ctrl Pts',(0.660242999639201,51.145,5.94245897164691));
#41871=CARTESIAN_POINT('Ctrl Pts',(0.660838563360921,51.145,5.95531437453424));
#41872=CARTESIAN_POINT('Ctrl Pts',(0.661043615595512,51.145,5.97401619058907));
#41873=CARTESIAN_POINT('Ctrl Pts',(0.660311421925997,51.145,5.99999062205823));
#41874=CARTESIAN_POINT('Ctrl Pts',(0.658581184594088,51.145,6.0285167231501));
#41875=CARTESIAN_POINT('Ctrl Pts',(0.655842009648633,51.145,6.05948455921138));
#41876=CARTESIAN_POINT('Ctrl Pts',(0.652083489461619,51.145,6.09268249742298));
#41877=CARTESIAN_POINT('Ctrl Pts',(0.64729662973892,51.145,6.12780215712604));
#41878=CARTESIAN_POINT('Ctrl Pts',(0.641473544543614,51.145,6.16449561918676));
#41879=CARTESIAN_POINT('Ctrl Pts',(0.634607707876564,51.145,6.20242090374318));
#41880=CARTESIAN_POINT('Ctrl Pts',(0.626694128202842,51.145,6.24128706412515));
#41881=CARTESIAN_POINT('Ctrl Pts',(0.617730009530307,51.145,6.2809112037544));
#41882=CARTESIAN_POINT('Ctrl Pts',(0.607714431517401,51.145,6.32121490697716));
#41883=CARTESIAN_POINT('Ctrl Pts',(0.596647533682211,51.145,6.36218460951727));
#41884=CARTESIAN_POINT('Ctrl Pts',(0.584530087032237,51.145,6.40384227175352));
#41885=CARTESIAN_POINT('Ctrl Pts',(0.571363102905579,51.145,6.44621447382266));
#41886=CARTESIAN_POINT('Ctrl Pts',(0.557147755196277,51.145,6.4892958755784));
#41887=CARTESIAN_POINT('Ctrl Pts',(0.541884929839949,51.145,6.53304612199323));
#41888=CARTESIAN_POINT('Ctrl Pts',(0.525574676214356,51.145,6.57740496530571));
#41889=CARTESIAN_POINT('Ctrl Pts',(0.508215876982668,51.145,6.62230172760513));
#41890=CARTESIAN_POINT('Ctrl Pts',(0.489806088474622,51.145,6.66766610085618));
#41891=CARTESIAN_POINT('Ctrl Pts',(0.470341429749655,51.145,6.71344014059664));
#41892=CARTESIAN_POINT('Ctrl Pts',(0.449817078488629,51.145,6.75958168761858));
#41893=CARTESIAN_POINT('Ctrl Pts',(0.428228256434473,51.145,6.80606015708966));
#41894=CARTESIAN_POINT('Ctrl Pts',(0.405571362419756,51.145,6.85285448604159));
#41895=CARTESIAN_POINT('Ctrl Pts',(0.381845111328234,51.145,6.89995030467727));
#41896=CARTESIAN_POINT('Ctrl Pts',(0.357052332559035,51.145,6.94733716327837));
#41897=CARTESIAN_POINT('Ctrl Pts',(0.331200384094009,51.145,6.99500658045299));
#41898=CARTESIAN_POINT('Ctrl Pts',(0.304298370266204,51.145,7.0429523011241));
#41899=CARTESIAN_POINT('Ctrl Pts',(0.28194386193484,51.145,7.0815264936403));
#41900=CARTESIAN_POINT('Ctrl Pts',(0.264712515322387,51.145,7.11057846529273));
#41901=CARTESIAN_POINT('Ctrl Pts',(0.253018452443275,51.145,7.13000027153808));
#41902=CARTESIAN_POINT('Ctrl Pts',(0.247119796320917,51.145,7.13972463098307));
#41903=CARTESIAN_POINT('',(-0.247119796320916,51.145,7.13972463098307));
#41904=CARTESIAN_POINT('Origin',(4.16333634234434E-16,51.145,1.6286971771251E-12));
#41905=CARTESIAN_POINT('',(-0.659304453656787,51.145,5.93051272372135));
#41906=CARTESIAN_POINT('Ctrl Pts',(-0.247119796320916,51.145,7.13972463098307));
#41907=CARTESIAN_POINT('Ctrl Pts',(-0.253018452443266,51.145,7.13000027153814));
#41908=CARTESIAN_POINT('Ctrl Pts',(-0.264712515322364,51.145,7.1105784652929));
#41909=CARTESIAN_POINT('Ctrl Pts',(-0.281943861934804,51.145,7.0815264936406));
#41910=CARTESIAN_POINT('Ctrl Pts',(-0.304298370266163,51.145,7.04295230112448));
#41911=CARTESIAN_POINT('Ctrl Pts',(-0.331200384093975,51.145,6.99500658045334));
#41912=CARTESIAN_POINT('Ctrl Pts',(-0.357052332559017,51.145,6.94733716327859));
#41913=CARTESIAN_POINT('Ctrl Pts',(-0.381845111328231,51.145,6.89995030467732));
#41914=CARTESIAN_POINT('Ctrl Pts',(-0.405571362419762,51.145,6.85285448604147));
#41915=CARTESIAN_POINT('Ctrl Pts',(-0.428228256434482,51.145,6.80606015708944));
#41916=CARTESIAN_POINT('Ctrl Pts',(-0.449817078488635,51.145,6.75958168761835));
#41917=CARTESIAN_POINT('Ctrl Pts',(-0.470341429749656,51.145,6.71344014059646));
#41918=CARTESIAN_POINT('Ctrl Pts',(-0.48980608847462,51.145,6.66766610085612));
#41919=CARTESIAN_POINT('Ctrl Pts',(-0.508215876982667,51.145,6.62230172760518));
#41920=CARTESIAN_POINT('Ctrl Pts',(-0.52557467621436,51.145,6.57740496530586));
#41921=CARTESIAN_POINT('Ctrl Pts',(-0.541884929839958,51.145,6.53304612199338));
#41922=CARTESIAN_POINT('Ctrl Pts',(-0.557147755196287,51.145,6.48929587557851));
#41923=CARTESIAN_POINT('Ctrl Pts',(-0.571363102905585,51.145,6.4462144738227));
#41924=CARTESIAN_POINT('Ctrl Pts',(-0.584530087032233,51.145,6.40384227175349));
#41925=CARTESIAN_POINT('Ctrl Pts',(-0.596647533682196,51.145,6.36218460951721));
#41926=CARTESIAN_POINT('Ctrl Pts',(-0.607714431517378,51.145,6.32121490697708));
#41927=CARTESIAN_POINT('Ctrl Pts',(-0.617730009530283,51.145,6.28091120375433));
#41928=CARTESIAN_POINT('Ctrl Pts',(-0.626694128202828,51.145,6.24128706412512));
#41929=CARTESIAN_POINT('Ctrl Pts',(-0.63460770787657,51.145,6.2024209037432));
#41930=CARTESIAN_POINT('Ctrl Pts',(-0.641473544543643,51.145,6.16449561918681));
#41931=CARTESIAN_POINT('Ctrl Pts',(-0.647296629738964,51.145,6.12780215712609));
#41932=CARTESIAN_POINT('Ctrl Pts',(-0.652083489461663,51.145,6.092682497423));
#41933=CARTESIAN_POINT('Ctrl Pts',(-0.655842009648655,51.145,6.05948455921138));
#41934=CARTESIAN_POINT('Ctrl Pts',(-0.658581184594065,51.145,6.02851672315009));
#41935=CARTESIAN_POINT('Ctrl Pts',(-0.660311421925919,51.145,5.99999062205821));
#41936=CARTESIAN_POINT('Ctrl Pts',(-0.661043615595395,51.145,5.97401619058905));
#41937=CARTESIAN_POINT('Ctrl Pts',(-0.660838563360812,51.145,5.95531437453421));
#41938=CARTESIAN_POINT('Ctrl Pts',(-0.660242999639131,51.145,5.94245897164689));
#41939=CARTESIAN_POINT('Ctrl Pts',(-0.65964996727821,51.145,5.93440822125369));
#41940=CARTESIAN_POINT('Ctrl Pts',(-0.659304453656787,51.145,5.93051272372135));
#41941=CARTESIAN_POINT('',(-0.592010183030743,51.145,5.32519370006274));
#41942=CARTESIAN_POINT('',(-0.659304453656787,51.145,5.93051272372135));
#41943=CARTESIAN_POINT('Origin',(0.,51.145,0.));
#41944=CARTESIAN_POINT('',(-3.261,51.145,-3.99357321201952E-16));
#41945=CARTESIAN_POINT('Origin',(0.,51.145,0.));
#41946=CARTESIAN_POINT('Origin',(0.,54.32,0.));
#41947=CARTESIAN_POINT('',(0.592010183030744,54.32,5.32519370006274));
#41948=CARTESIAN_POINT('Origin',(0.575436549687218,57.495,5.17611212951227));
#41949=CARTESIAN_POINT('',(0.659304453656788,57.495,5.93051272372135));
#41950=CARTESIAN_POINT('Origin',(4.16333634234434E-16,57.495,1.6286971771251E-12));
#41951=CARTESIAN_POINT('',(-0.247119796320916,57.495,7.13972463098307));
#41952=CARTESIAN_POINT('',(0.24711979632092,57.495,7.13972463098307));
#41953=CARTESIAN_POINT('Ctrl Pts',(0.659304453656788,57.495,5.93051272372135));
#41954=CARTESIAN_POINT('Ctrl Pts',(0.659304453656788,49.875,5.93051272372135));
#41955=CARTESIAN_POINT('Ctrl Pts',(0.659649967278236,57.495,5.9344082212537));
#41956=CARTESIAN_POINT('Ctrl Pts',(0.659649967278236,49.875,5.9344082212537));
#41957=CARTESIAN_POINT('Ctrl Pts',(0.660242999639201,57.495,5.94245897164691));
#41958=CARTESIAN_POINT('Ctrl Pts',(0.660242999639201,49.875,5.94245897164691));
#41959=CARTESIAN_POINT('Ctrl Pts',(0.660838563360921,57.495,5.95531437453424));
#41960=CARTESIAN_POINT('Ctrl Pts',(0.660838563360921,49.875,5.95531437453424));
#41961=CARTESIAN_POINT('Ctrl Pts',(0.661043615595512,57.495,5.97401619058907));
#41962=CARTESIAN_POINT('Ctrl Pts',(0.661043615595512,49.875,5.97401619058907));
#41963=CARTESIAN_POINT('Ctrl Pts',(0.660311421925997,57.495,5.99999062205823));
#41964=CARTESIAN_POINT('Ctrl Pts',(0.660311421925997,49.875,5.99999062205823));
#41965=CARTESIAN_POINT('Ctrl Pts',(0.658581184594088,57.495,6.0285167231501));
#41966=CARTESIAN_POINT('Ctrl Pts',(0.658581184594088,49.875,6.0285167231501));
#41967=CARTESIAN_POINT('Ctrl Pts',(0.655842009648633,57.495,6.05948455921138));
#41968=CARTESIAN_POINT('Ctrl Pts',(0.655842009648633,49.875,6.05948455921138));
#41969=CARTESIAN_POINT('Ctrl Pts',(0.652083489461619,57.495,6.09268249742298));
#41970=CARTESIAN_POINT('Ctrl Pts',(0.652083489461619,49.875,6.09268249742298));
#41971=CARTESIAN_POINT('Ctrl Pts',(0.64729662973892,57.495,6.12780215712604));
#41972=CARTESIAN_POINT('Ctrl Pts',(0.64729662973892,49.875,6.12780215712604));
#41973=CARTESIAN_POINT('Ctrl Pts',(0.641473544543614,57.495,6.16449561918676));
#41974=CARTESIAN_POINT('Ctrl Pts',(0.641473544543614,49.875,6.16449561918676));
#41975=CARTESIAN_POINT('Ctrl Pts',(0.634607707876564,57.495,6.20242090374318));
#41976=CARTESIAN_POINT('Ctrl Pts',(0.634607707876564,49.875,6.20242090374318));
#41977=CARTESIAN_POINT('Ctrl Pts',(0.626694128202842,57.495,6.24128706412515));
#41978=CARTESIAN_POINT('Ctrl Pts',(0.626694128202842,49.875,6.24128706412515));
#41979=CARTESIAN_POINT('Ctrl Pts',(0.617730009530307,57.495,6.2809112037544));
#41980=CARTESIAN_POINT('Ctrl Pts',(0.617730009530307,49.875,6.2809112037544));
#41981=CARTESIAN_POINT('Ctrl Pts',(0.607714431517401,57.495,6.32121490697716));
#41982=CARTESIAN_POINT('Ctrl Pts',(0.607714431517401,49.875,6.32121490697716));
#41983=CARTESIAN_POINT('Ctrl Pts',(0.596647533682211,57.495,6.36218460951727));
#41984=CARTESIAN_POINT('Ctrl Pts',(0.596647533682211,49.875,6.36218460951727));
#41985=CARTESIAN_POINT('Ctrl Pts',(0.584530087032237,57.495,6.40384227175352));
#41986=CARTESIAN_POINT('Ctrl Pts',(0.584530087032237,49.875,6.40384227175352));
#41987=CARTESIAN_POINT('Ctrl Pts',(0.571363102905579,57.495,6.44621447382266));
#41988=CARTESIAN_POINT('Ctrl Pts',(0.571363102905579,49.875,6.44621447382266));
#41989=CARTESIAN_POINT('Ctrl Pts',(0.557147755196277,57.495,6.4892958755784));
#41990=CARTESIAN_POINT('Ctrl Pts',(0.557147755196277,49.875,6.4892958755784));
#41991=CARTESIAN_POINT('Ctrl Pts',(0.541884929839949,57.495,6.53304612199323));
#41992=CARTESIAN_POINT('Ctrl Pts',(0.541884929839949,49.875,6.53304612199323));
#41993=CARTESIAN_POINT('Ctrl Pts',(0.525574676214356,57.495,6.57740496530571));
#41994=CARTESIAN_POINT('Ctrl Pts',(0.525574676214356,49.875,6.57740496530571));
#41995=CARTESIAN_POINT('Ctrl Pts',(0.508215876982668,57.495,6.62230172760513));
#41996=CARTESIAN_POINT('Ctrl Pts',(0.508215876982668,49.875,6.62230172760513));
#41997=CARTESIAN_POINT('Ctrl Pts',(0.489806088474622,57.495,6.66766610085618));
#41998=CARTESIAN_POINT('Ctrl Pts',(0.489806088474622,49.875,6.66766610085618));
#41999=CARTESIAN_POINT('Ctrl Pts',(0.470341429749655,57.495,6.71344014059664));
#42000=CARTESIAN_POINT('Ctrl Pts',(0.470341429749655,49.875,6.71344014059664));
#42001=CARTESIAN_POINT('Ctrl Pts',(0.449817078488629,57.495,6.75958168761858));
#42002=CARTESIAN_POINT('Ctrl Pts',(0.449817078488629,49.875,6.75958168761858));
#42003=CARTESIAN_POINT('Ctrl Pts',(0.428228256434473,57.495,6.80606015708966));
#42004=CARTESIAN_POINT('Ctrl Pts',(0.428228256434473,49.875,6.80606015708966));
#42005=CARTESIAN_POINT('Ctrl Pts',(0.405571362419756,57.495,6.85285448604159));
#42006=CARTESIAN_POINT('Ctrl Pts',(0.405571362419756,49.875,6.85285448604159));
#42007=CARTESIAN_POINT('Ctrl Pts',(0.381845111328234,57.495,6.89995030467727));
#42008=CARTESIAN_POINT('Ctrl Pts',(0.381845111328234,49.875,6.89995030467727));
#42009=CARTESIAN_POINT('Ctrl Pts',(0.357052332559035,57.495,6.94733716327837));
#42010=CARTESIAN_POINT('Ctrl Pts',(0.357052332559035,49.875,6.94733716327837));
#42011=CARTESIAN_POINT('Ctrl Pts',(0.331200384094009,57.495,6.99500658045299));
#42012=CARTESIAN_POINT('Ctrl Pts',(0.331200384094009,49.875,6.99500658045299));
#42013=CARTESIAN_POINT('Ctrl Pts',(0.304298370266204,57.495,7.0429523011241));
#42014=CARTESIAN_POINT('Ctrl Pts',(0.304298370266204,49.875,7.0429523011241));
#42015=CARTESIAN_POINT('Ctrl Pts',(0.28194386193484,57.495,7.0815264936403));
#42016=CARTESIAN_POINT('Ctrl Pts',(0.28194386193484,49.875,7.0815264936403));
#42017=CARTESIAN_POINT('Ctrl Pts',(0.264712515322387,57.495,7.11057846529273));
#42018=CARTESIAN_POINT('Ctrl Pts',(0.264712515322387,49.875,7.11057846529273));
#42019=CARTESIAN_POINT('Ctrl Pts',(0.253018452443275,57.495,7.13000027153808));
#42020=CARTESIAN_POINT('Ctrl Pts',(0.253018452443275,49.875,7.13000027153808));
#42021=CARTESIAN_POINT('Ctrl Pts',(0.247119796320917,57.495,7.13972463098307));
#42022=CARTESIAN_POINT('Ctrl Pts',(0.247119796320917,49.875,7.13972463098307));
#42023=CARTESIAN_POINT('Origin',(-0.659304453656787,57.495,5.93051272372135));
#42024=CARTESIAN_POINT('',(-0.592010183030743,54.32,5.32519370006274));
#42025=CARTESIAN_POINT('',(-0.659304453656787,57.495,5.93051272372135));
#42026=CARTESIAN_POINT('Ctrl Pts',(-0.247119796320916,57.495,7.13972463098307));
#42027=CARTESIAN_POINT('Ctrl Pts',(-0.247119796320916,49.875,7.13972463098307));
#42028=CARTESIAN_POINT('Ctrl Pts',(-0.253018452443266,57.495,7.13000027153814));
#42029=CARTESIAN_POINT('Ctrl Pts',(-0.253018452443266,49.875,7.13000027153814));
#42030=CARTESIAN_POINT('Ctrl Pts',(-0.264712515322364,57.495,7.1105784652929));
#42031=CARTESIAN_POINT('Ctrl Pts',(-0.264712515322364,49.875,7.1105784652929));
#42032=CARTESIAN_POINT('Ctrl Pts',(-0.281943861934804,57.495,7.0815264936406));
#42033=CARTESIAN_POINT('Ctrl Pts',(-0.281943861934804,49.875,7.0815264936406));
#42034=CARTESIAN_POINT('Ctrl Pts',(-0.304298370266163,57.495,7.04295230112448));
#42035=CARTESIAN_POINT('Ctrl Pts',(-0.304298370266163,49.875,7.04295230112448));
#42036=CARTESIAN_POINT('Ctrl Pts',(-0.331200384093975,57.495,6.99500658045334));
#42037=CARTESIAN_POINT('Ctrl Pts',(-0.331200384093975,49.875,6.99500658045334));
#42038=CARTESIAN_POINT('Ctrl Pts',(-0.357052332559017,57.495,6.94733716327859));
#42039=CARTESIAN_POINT('Ctrl Pts',(-0.357052332559017,49.875,6.94733716327859));
#42040=CARTESIAN_POINT('Ctrl Pts',(-0.381845111328231,57.495,6.89995030467732));
#42041=CARTESIAN_POINT('Ctrl Pts',(-0.381845111328231,49.875,6.89995030467732));
#42042=CARTESIAN_POINT('Ctrl Pts',(-0.405571362419762,57.495,6.85285448604147));
#42043=CARTESIAN_POINT('Ctrl Pts',(-0.405571362419762,49.875,6.85285448604147));
#42044=CARTESIAN_POINT('Ctrl Pts',(-0.428228256434482,57.495,6.80606015708944));
#42045=CARTESIAN_POINT('Ctrl Pts',(-0.428228256434482,49.875,6.80606015708944));
#42046=CARTESIAN_POINT('Ctrl Pts',(-0.449817078488635,57.495,6.75958168761835));
#42047=CARTESIAN_POINT('Ctrl Pts',(-0.449817078488635,49.875,6.75958168761835));
#42048=CARTESIAN_POINT('Ctrl Pts',(-0.470341429749656,57.495,6.71344014059646));
#42049=CARTESIAN_POINT('Ctrl Pts',(-0.470341429749656,49.875,6.71344014059646));
#42050=CARTESIAN_POINT('Ctrl Pts',(-0.48980608847462,57.495,6.66766610085612));
#42051=CARTESIAN_POINT('Ctrl Pts',(-0.48980608847462,49.875,6.66766610085612));
#42052=CARTESIAN_POINT('Ctrl Pts',(-0.508215876982667,57.495,6.62230172760518));
#42053=CARTESIAN_POINT('Ctrl Pts',(-0.508215876982667,49.875,6.62230172760518));
#42054=CARTESIAN_POINT('Ctrl Pts',(-0.52557467621436,57.495,6.57740496530586));
#42055=CARTESIAN_POINT('Ctrl Pts',(-0.52557467621436,49.875,6.57740496530586));
#42056=CARTESIAN_POINT('Ctrl Pts',(-0.541884929839958,57.495,6.53304612199338));
#42057=CARTESIAN_POINT('Ctrl Pts',(-0.541884929839958,49.875,6.53304612199338));
#42058=CARTESIAN_POINT('Ctrl Pts',(-0.557147755196287,57.495,6.48929587557851));
#42059=CARTESIAN_POINT('Ctrl Pts',(-0.557147755196287,49.875,6.48929587557851));
#42060=CARTESIAN_POINT('Ctrl Pts',(-0.571363102905585,57.495,6.4462144738227));
#42061=CARTESIAN_POINT('Ctrl Pts',(-0.571363102905585,49.875,6.4462144738227));
#42062=CARTESIAN_POINT('Ctrl Pts',(-0.584530087032233,57.495,6.40384227175349));
#42063=CARTESIAN_POINT('Ctrl Pts',(-0.584530087032233,49.875,6.40384227175349));
#42064=CARTESIAN_POINT('Ctrl Pts',(-0.596647533682196,57.495,6.36218460951721));
#42065=CARTESIAN_POINT('Ctrl Pts',(-0.596647533682196,49.875,6.36218460951721));
#42066=CARTESIAN_POINT('Ctrl Pts',(-0.607714431517378,57.495,6.32121490697708));
#42067=CARTESIAN_POINT('Ctrl Pts',(-0.607714431517378,49.875,6.32121490697708));
#42068=CARTESIAN_POINT('Ctrl Pts',(-0.617730009530283,57.495,6.28091120375433));
#42069=CARTESIAN_POINT('Ctrl Pts',(-0.617730009530283,49.875,6.28091120375433));
#42070=CARTESIAN_POINT('Ctrl Pts',(-0.626694128202828,57.495,6.24128706412512));
#42071=CARTESIAN_POINT('Ctrl Pts',(-0.626694128202828,49.875,6.24128706412512));
#42072=CARTESIAN_POINT('Ctrl Pts',(-0.63460770787657,57.495,6.2024209037432));
#42073=CARTESIAN_POINT('Ctrl Pts',(-0.63460770787657,49.875,6.2024209037432));
#42074=CARTESIAN_POINT('Ctrl Pts',(-0.641473544543643,57.495,6.16449561918681));
#42075=CARTESIAN_POINT('Ctrl Pts',(-0.641473544543643,49.875,6.16449561918681));
#42076=CARTESIAN_POINT('Ctrl Pts',(-0.647296629738964,57.495,6.12780215712609));
#42077=CARTESIAN_POINT('Ctrl Pts',(-0.647296629738964,49.875,6.12780215712609));
#42078=CARTESIAN_POINT('Ctrl Pts',(-0.652083489461663,57.495,6.092682497423));
#42079=CARTESIAN_POINT('Ctrl Pts',(-0.652083489461663,49.875,6.092682497423));
#42080=CARTESIAN_POINT('Ctrl Pts',(-0.655842009648655,57.495,6.05948455921138));
#42081=CARTESIAN_POINT('Ctrl Pts',(-0.655842009648655,49.875,6.05948455921138));
#42082=CARTESIAN_POINT('Ctrl Pts',(-0.658581184594065,57.495,6.02851672315009));
#42083=CARTESIAN_POINT('Ctrl Pts',(-0.658581184594065,49.875,6.02851672315009));
#42084=CARTESIAN_POINT('Ctrl Pts',(-0.660311421925919,57.495,5.99999062205821));
#42085=CARTESIAN_POINT('Ctrl Pts',(-0.660311421925919,49.875,5.99999062205821));
#42086=CARTESIAN_POINT('Ctrl Pts',(-0.661043615595395,57.495,5.97401619058905));
#42087=CARTESIAN_POINT('Ctrl Pts',(-0.661043615595395,49.875,5.97401619058905));
#42088=CARTESIAN_POINT('Ctrl Pts',(-0.660838563360812,57.495,5.95531437453421));
#42089=CARTESIAN_POINT('Ctrl Pts',(-0.660838563360812,49.875,5.95531437453421));
#42090=CARTESIAN_POINT('Ctrl Pts',(-0.660242999639131,57.495,5.94245897164689));
#42091=CARTESIAN_POINT('Ctrl Pts',(-0.660242999639131,49.875,5.94245897164689));
#42092=CARTESIAN_POINT('Ctrl Pts',(-0.65964996727821,57.495,5.93440822125369));
#42093=CARTESIAN_POINT('Ctrl Pts',(-0.65964996727821,49.875,5.93440822125369));
#42094=CARTESIAN_POINT('Ctrl Pts',(-0.659304453656787,57.495,5.93051272372135));
#42095=CARTESIAN_POINT('Ctrl Pts',(-0.659304453656787,49.875,5.93051272372135));
#42096=CARTESIAN_POINT('Origin',(0.,54.32,0.));
#42097=CARTESIAN_POINT('Origin',(1.6,53.935,0.));
#42098=CARTESIAN_POINT('',(-3.261,53.935,-3.99357321201952E-16));
#42099=CARTESIAN_POINT('Origin',(0.,53.935,0.));
#42100=CARTESIAN_POINT('',(-1.6,53.935,-1.95943487863577E-16));
#42101=CARTESIAN_POINT('Origin',(0.,53.935,0.));
#42102=CARTESIAN_POINT('Origin',(0.,54.825,0.));
#42103=CARTESIAN_POINT('',(-1.6,55.715,-1.95943487863577E-16));
#42104=CARTESIAN_POINT('Origin',(0.,55.715,0.));
#42105=CARTESIAN_POINT('',(-1.6,54.825,-1.95943487863577E-16));
#42106=CARTESIAN_POINT('Origin',(4.477,55.715,0.));
#42107=CARTESIAN_POINT('',(-4.477,55.715,-5.4827437197827E-16));
#42108=CARTESIAN_POINT('Origin',(0.,55.715,0.));
#42109=CARTESIAN_POINT('Origin',(0.,56.605,0.));
#42110=CARTESIAN_POINT('',(-4.477,56.605,-5.4827437197827E-16));
#42111=CARTESIAN_POINT('Origin',(0.,52.54,0.));
#42112=CARTESIAN_POINT('',(-3.261,52.54,-3.99357321201952E-16));
#83192=UNCERTAINTY_MEASURE_WITH_UNIT(LENGTH_MEASURE(0.01),#83220,
'DISTANCE_ACCURACY_VALUE',
'Maximum model space distance between geometric entities at asserted c
onnectivities');
#83203=UNCERTAINTY_MEASURE_WITH_UNIT(LENGTH_MEASURE(0.01),#83220,
'DISTANCE_ACCURACY_VALUE',
'Maximum model space distance between geometric entities at asserted c
onnectivities');
#83208=(
GEOMETRIC_REPRESENTATION_CONTEXT(3)
GLOBAL_UNCERTAINTY_ASSIGNED_CONTEXT((#83192))
GLOBAL_UNIT_ASSIGNED_CONTEXT((#83220,#83222,#83223))
REPRESENTATION_CONTEXT('','3D')
);
#83219=(
GEOMETRIC_REPRESENTATION_CONTEXT(3)
GLOBAL_UNCERTAINTY_ASSIGNED_CONTEXT((#83203))
GLOBAL_UNIT_ASSIGNED_CONTEXT((#83220,#83222,#83223))
REPRESENTATION_CONTEXT('','3D')
);
#83220=(
LENGTH_UNIT()
NAMED_UNIT(*)
SI_UNIT(.MILLI.,.METRE.)
);
#83222=(
NAMED_UNIT(*)
PLANE_ANGLE_UNIT()
SI_UNIT($,.RADIAN.)
);
#83223=(
NAMED_UNIT(*)
SI_UNIT($,.STERADIAN.)
SOLID_ANGLE_UNIT()
);
#83228=SHAPE_DEFINITION_REPRESENTATION(#83243,#83303);
#83243=PRODUCT_DEFINITION_SHAPE('',$,#83319);
#83303=SHAPE_REPRESENTATION('',(#27453),#83208);
#83314=PRODUCT_DEFINITION_CONTEXT('part definition',#83361,'design');
#83319=PRODUCT_DEFINITION('16T 32P Metal Servo Gear',
'16T 32P Metal Servo Gear',#83334,#83314);
#83334=PRODUCT_DEFINITION_FORMATION('',$,#83367);
#83361=APPLICATION_CONTEXT(
'Core Data for Automotive Mechanical Design Process');
#83362=PRODUCT_CONTEXT('part definition',#83361,'mechanical');
#83367=PRODUCT('16T 32P Metal Servo Gear','16T 32P Metal Servo Gear',$,
(#83362));
#83382=PRESENTATION_STYLE_ASSIGNMENT((#83397));
#83397=SURFACE_STYLE_USAGE(.BOTH.,#83412);
#83412=SURFACE_SIDE_STYLE('',(#83427));
#83427=SURFACE_STYLE_FILL_AREA(#83442);
#83442=FILL_AREA_STYLE('Opaque(238,239,241)',(#83457));
#83457=FILL_AREA_STYLE_COLOUR('Opaque(238,239,241)',#83472);
#83472=COLOUR_RGB('Opaque(238,239,241)', 0.72549020, 0.75294118, 0.79215686);
ENDSEC;
END-ISO-10303-21;
